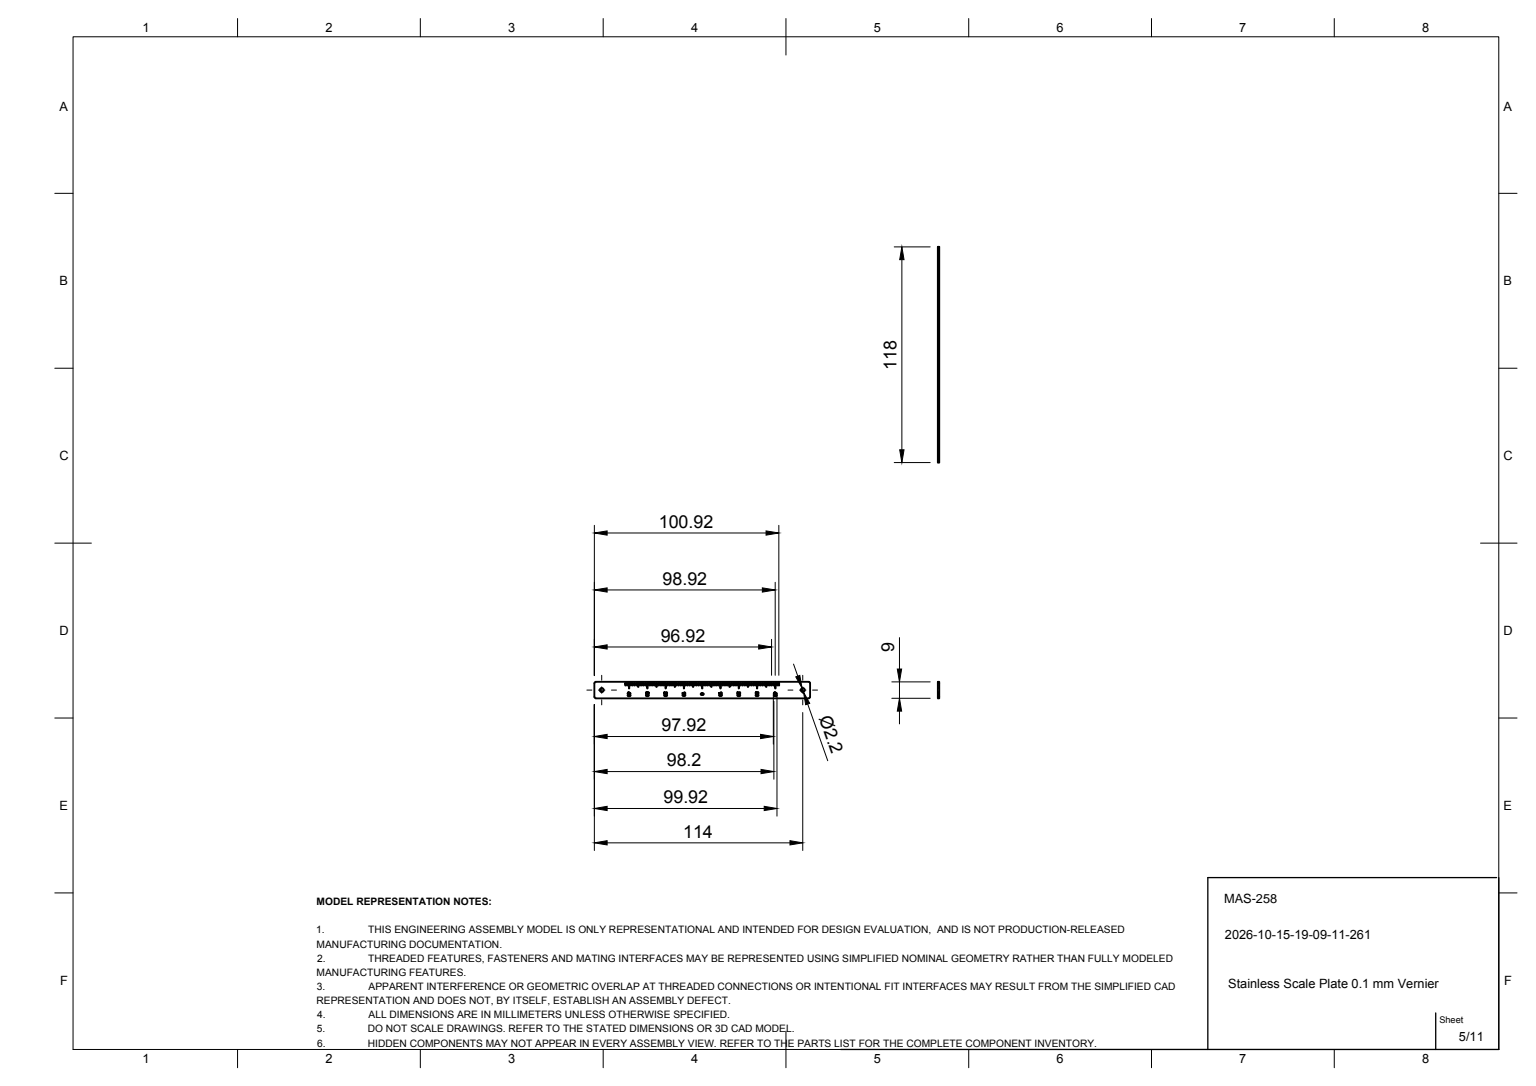
ISO-10303-21;
HEADER;
/* Generated by software containing ST-Developer
 * from STEP Tools, Inc. (www.steptools.com) 
 */

FILE_DESCRIPTION(
/* description */ (''),
/* implementation_level */ '2;1');

FILE_NAME(
/* name */ 'Stainless Scale Plate 0.1 mm Vernier.step',
/* time_stamp */ '2026-10-15T12:29:06-07:00',
/* author */ (''),
/* organization */ (''),
/* preprocessor_version */ 'ST-DEVELOPER v20.2',
/* originating_system */ 'Autodesk Translation Framework v15.15.0.0',
/* authorisation */ '');

FILE_SCHEMA (('AUTOMOTIVE_DESIGN { 1 0 10303 214 3 1 1 }'));
ENDSEC;

DATA;
#10=MECHANICAL_DESIGN_GEOMETRIC_PRESENTATION_REPRESENTATION('',(#1744),#135282);
#331=B_SPLINE_SURFACE_WITH_KNOTS('',2,1,((#69951,#69952),(#69953,#69954),
(#69955,#69956)),.UNSPECIFIED.,.F.,.F.,.F.,(3,3),(2,2),(0.,1.),(0.,0.0172800000000002),
 .UNSPECIFIED.);
#332=B_SPLINE_SURFACE_WITH_KNOTS('',2,1,((#69969,#69970),(#69971,#69972),
(#69973,#69974)),.UNSPECIFIED.,.F.,.F.,.F.,(3,3),(2,2),(0.,1.),(0.,0.0172800000000002),
 .UNSPECIFIED.);
#333=B_SPLINE_SURFACE_WITH_KNOTS('',2,1,((#69984,#69985),(#69986,#69987),
(#69988,#69989)),.UNSPECIFIED.,.F.,.F.,.F.,(3,3),(2,2),(0.,1.),(0.,0.0172800000000002),
 .UNSPECIFIED.);
#334=B_SPLINE_SURFACE_WITH_KNOTS('',2,1,((#69999,#70000),(#70001,#70002),
(#70003,#70004)),.UNSPECIFIED.,.F.,.F.,.F.,(3,3),(2,2),(0.,1.),(0.,0.0172800000000002),
 .UNSPECIFIED.);
#335=B_SPLINE_SURFACE_WITH_KNOTS('',2,1,((#70014,#70015),(#70016,#70017),
(#70018,#70019)),.UNSPECIFIED.,.F.,.F.,.F.,(3,3),(2,2),(0.,1.),(0.,0.0172800000000002),
 .UNSPECIFIED.);
#336=B_SPLINE_SURFACE_WITH_KNOTS('',2,1,((#70029,#70030),(#70031,#70032),
(#70033,#70034)),.UNSPECIFIED.,.F.,.F.,.F.,(3,3),(2,2),(0.,1.),(0.,0.0172800000000002),
 .UNSPECIFIED.);
#337=B_SPLINE_SURFACE_WITH_KNOTS('',2,1,((#70044,#70045),(#70046,#70047),
(#70048,#70049)),.UNSPECIFIED.,.F.,.F.,.F.,(3,3),(2,2),(0.,1.),(0.,0.0172800000000002),
 .UNSPECIFIED.);
#338=B_SPLINE_SURFACE_WITH_KNOTS('',2,1,((#70059,#70060),(#70061,#70062),
(#70063,#70064)),.UNSPECIFIED.,.F.,.F.,.F.,(3,3),(2,2),(0.,1.),(0.,0.0172800000000002),
 .UNSPECIFIED.);
#339=B_SPLINE_SURFACE_WITH_KNOTS('',2,1,((#70071,#70072),(#70073,#70074),
(#70075,#70076)),.UNSPECIFIED.,.F.,.F.,.F.,(3,3),(2,2),(0.,1.),(0.,0.0172800000000002),
 .UNSPECIFIED.);
#340=B_SPLINE_SURFACE_WITH_KNOTS('',2,1,((#70089,#70090),(#70091,#70092),
(#70093,#70094)),.UNSPECIFIED.,.F.,.F.,.F.,(3,3),(2,2),(0.,1.),(0.,0.0172800000000002),
 .UNSPECIFIED.);
#341=B_SPLINE_SURFACE_WITH_KNOTS('',2,1,((#70104,#70105),(#70106,#70107),
(#70108,#70109)),.UNSPECIFIED.,.F.,.F.,.F.,(3,3),(2,2),(0.,1.),(0.,0.0172800000000002),
 .UNSPECIFIED.);
#342=B_SPLINE_SURFACE_WITH_KNOTS('',2,1,((#70119,#70120),(#70121,#70122),
(#70123,#70124)),.UNSPECIFIED.,.F.,.F.,.F.,(3,3),(2,2),(0.,1.),(0.,0.0172800000000002),
 .UNSPECIFIED.);
#343=B_SPLINE_SURFACE_WITH_KNOTS('',2,1,((#70134,#70135),(#70136,#70137),
(#70138,#70139)),.UNSPECIFIED.,.F.,.F.,.F.,(3,3),(2,2),(0.,1.),(0.,0.0172800000000002),
 .UNSPECIFIED.);
#344=B_SPLINE_SURFACE_WITH_KNOTS('',2,1,((#70149,#70150),(#70151,#70152),
(#70153,#70154)),.UNSPECIFIED.,.F.,.F.,.F.,(3,3),(2,2),(0.,1.),(0.,0.0172800000000002),
 .UNSPECIFIED.);
#345=B_SPLINE_SURFACE_WITH_KNOTS('',2,1,((#70164,#70165),(#70166,#70167),
(#70168,#70169)),.UNSPECIFIED.,.F.,.F.,.F.,(3,3),(2,2),(0.,1.),(0.,0.0172800000000002),
 .UNSPECIFIED.);
#346=B_SPLINE_SURFACE_WITH_KNOTS('',2,1,((#70179,#70180),(#70181,#70182),
(#70183,#70184)),.UNSPECIFIED.,.F.,.F.,.F.,(3,3),(2,2),(0.,1.),(0.,0.0172800000000002),
 .UNSPECIFIED.);
#347=B_SPLINE_SURFACE_WITH_KNOTS('',2,1,((#70194,#70195),(#70196,#70197),
(#70198,#70199)),.UNSPECIFIED.,.F.,.F.,.F.,(3,3),(2,2),(0.,1.),(0.,0.0172800000000002),
 .UNSPECIFIED.);
#348=B_SPLINE_SURFACE_WITH_KNOTS('',2,1,((#70209,#70210),(#70211,#70212),
(#70213,#70214)),.UNSPECIFIED.,.F.,.F.,.F.,(3,3),(2,2),(0.,1.),(0.,0.0172800000000002),
 .UNSPECIFIED.);
#349=B_SPLINE_SURFACE_WITH_KNOTS('',2,1,((#70224,#70225),(#70226,#70227),
(#70228,#70229)),.UNSPECIFIED.,.F.,.F.,.F.,(3,3),(2,2),(0.,1.),(0.,0.0172800000000002),
 .UNSPECIFIED.);
#350=B_SPLINE_SURFACE_WITH_KNOTS('',2,1,((#70239,#70240),(#70241,#70242),
(#70243,#70244)),.UNSPECIFIED.,.F.,.F.,.F.,(3,3),(2,2),(0.,1.),(0.,0.0172800000000002),
 .UNSPECIFIED.);
#351=B_SPLINE_SURFACE_WITH_KNOTS('',2,1,((#70339,#70340),(#70341,#70342),
(#70343,#70344)),.UNSPECIFIED.,.F.,.F.,.F.,(3,3),(2,2),(0.,1.),(0.,0.0172800000000002),
 .UNSPECIFIED.);
#352=B_SPLINE_SURFACE_WITH_KNOTS('',2,1,((#70357,#70358),(#70359,#70360),
(#70361,#70362)),.UNSPECIFIED.,.F.,.F.,.F.,(3,3),(2,2),(0.,1.),(0.,0.0172800000000002),
 .UNSPECIFIED.);
#353=B_SPLINE_SURFACE_WITH_KNOTS('',2,1,((#70372,#70373),(#70374,#70375),
(#70376,#70377)),.UNSPECIFIED.,.F.,.F.,.F.,(3,3),(2,2),(0.,1.),(0.,0.0172800000000002),
 .UNSPECIFIED.);
#354=B_SPLINE_SURFACE_WITH_KNOTS('',2,1,((#70387,#70388),(#70389,#70390),
(#70391,#70392)),.UNSPECIFIED.,.F.,.F.,.F.,(3,3),(2,2),(0.,1.),(0.,0.0172800000000002),
 .UNSPECIFIED.);
#355=B_SPLINE_SURFACE_WITH_KNOTS('',2,1,((#70402,#70403),(#70404,#70405),
(#70406,#70407)),.UNSPECIFIED.,.F.,.F.,.F.,(3,3),(2,2),(0.,1.),(0.,0.0172800000000002),
 .UNSPECIFIED.);
#356=B_SPLINE_SURFACE_WITH_KNOTS('',2,1,((#70417,#70418),(#70419,#70420),
(#70421,#70422)),.UNSPECIFIED.,.F.,.F.,.F.,(3,3),(2,2),(0.,1.),(0.,0.0172800000000002),
 .UNSPECIFIED.);
#357=B_SPLINE_SURFACE_WITH_KNOTS('',2,1,((#70432,#70433),(#70434,#70435),
(#70436,#70437)),.UNSPECIFIED.,.F.,.F.,.F.,(3,3),(2,2),(0.,1.),(0.,0.0172800000000002),
 .UNSPECIFIED.);
#358=B_SPLINE_SURFACE_WITH_KNOTS('',2,1,((#70447,#70448),(#70449,#70450),
(#70451,#70452)),.UNSPECIFIED.,.F.,.F.,.F.,(3,3),(2,2),(0.,1.),(0.,0.0172800000000002),
 .UNSPECIFIED.);
#359=B_SPLINE_SURFACE_WITH_KNOTS('',2,1,((#70459,#70460),(#70461,#70462),
(#70463,#70464)),.UNSPECIFIED.,.F.,.F.,.F.,(3,3),(2,2),(0.,1.),(0.,0.0172800000000002),
 .UNSPECIFIED.);
#360=B_SPLINE_SURFACE_WITH_KNOTS('',2,1,((#70477,#70478),(#70479,#70480),
(#70481,#70482)),.UNSPECIFIED.,.F.,.F.,.F.,(3,3),(2,2),(0.,1.),(0.,0.0172800000000002),
 .UNSPECIFIED.);
#361=B_SPLINE_SURFACE_WITH_KNOTS('',2,1,((#70492,#70493),(#70494,#70495),
(#70496,#70497)),.UNSPECIFIED.,.F.,.F.,.F.,(3,3),(2,2),(0.,1.),(0.,0.0172800000000002),
 .UNSPECIFIED.);
#362=B_SPLINE_SURFACE_WITH_KNOTS('',2,1,((#70507,#70508),(#70509,#70510),
(#70511,#70512)),.UNSPECIFIED.,.F.,.F.,.F.,(3,3),(2,2),(0.,1.),(0.,0.0172800000000002),
 .UNSPECIFIED.);
#363=B_SPLINE_SURFACE_WITH_KNOTS('',2,1,((#70522,#70523),(#70524,#70525),
(#70526,#70527)),.UNSPECIFIED.,.F.,.F.,.F.,(3,3),(2,2),(0.,1.),(0.,0.0172800000000002),
 .UNSPECIFIED.);
#364=B_SPLINE_SURFACE_WITH_KNOTS('',2,1,((#70537,#70538),(#70539,#70540),
(#70541,#70542)),.UNSPECIFIED.,.F.,.F.,.F.,(3,3),(2,2),(0.,1.),(0.,0.0172800000000002),
 .UNSPECIFIED.);
#365=B_SPLINE_SURFACE_WITH_KNOTS('',2,1,((#70552,#70553),(#70554,#70555),
(#70556,#70557)),.UNSPECIFIED.,.F.,.F.,.F.,(3,3),(2,2),(0.,1.),(0.,0.0172800000000002),
 .UNSPECIFIED.);
#366=B_SPLINE_SURFACE_WITH_KNOTS('',2,1,((#70567,#70568),(#70569,#70570),
(#70571,#70572)),.UNSPECIFIED.,.F.,.F.,.F.,(3,3),(2,2),(0.,1.),(0.,0.0172800000000002),
 .UNSPECIFIED.);
#367=B_SPLINE_SURFACE_WITH_KNOTS('',2,1,((#70582,#70583),(#70584,#70585),
(#70586,#70587)),.UNSPECIFIED.,.F.,.F.,.F.,(3,3),(2,2),(0.,1.),(0.,0.0172800000000002),
 .UNSPECIFIED.);
#368=B_SPLINE_SURFACE_WITH_KNOTS('',2,1,((#70597,#70598),(#70599,#70600),
(#70601,#70602)),.UNSPECIFIED.,.F.,.F.,.F.,(3,3),(2,2),(0.,1.),(0.,0.0172800000000002),
 .UNSPECIFIED.);
#369=B_SPLINE_SURFACE_WITH_KNOTS('',2,1,((#70612,#70613),(#70614,#70615),
(#70616,#70617)),.UNSPECIFIED.,.F.,.F.,.F.,(3,3),(2,2),(0.,1.),(0.,0.0172800000000002),
 .UNSPECIFIED.);
#370=B_SPLINE_SURFACE_WITH_KNOTS('',2,1,((#70627,#70628),(#70629,#70630),
(#70631,#70632)),.UNSPECIFIED.,.F.,.F.,.F.,(3,3),(2,2),(0.,1.),(0.,0.0172800000000002),
 .UNSPECIFIED.);
#371=B_SPLINE_SURFACE_WITH_KNOTS('',2,1,((#70640,#70641),(#70642,#70643),
(#70644,#70645)),.UNSPECIFIED.,.F.,.F.,.F.,(3,3),(2,2),(0.,1.),(0.,0.0172800000000002),
 .UNSPECIFIED.);
#372=B_SPLINE_SURFACE_WITH_KNOTS('',2,1,((#70658,#70659),(#70660,#70661),
(#70662,#70663)),.UNSPECIFIED.,.F.,.F.,.F.,(3,3),(2,2),(0.,1.),(0.,0.0172800000000002),
 .UNSPECIFIED.);
#373=B_SPLINE_SURFACE_WITH_KNOTS('',2,1,((#70673,#70674),(#70675,#70676),
(#70677,#70678)),.UNSPECIFIED.,.F.,.F.,.F.,(3,3),(2,2),(0.,1.),(0.,0.0172800000000002),
 .UNSPECIFIED.);
#374=B_SPLINE_SURFACE_WITH_KNOTS('',2,1,((#70688,#70689),(#70690,#70691),
(#70692,#70693)),.UNSPECIFIED.,.F.,.F.,.F.,(3,3),(2,2),(0.,1.),(0.,0.0172800000000002),
 .UNSPECIFIED.);
#375=B_SPLINE_SURFACE_WITH_KNOTS('',2,1,((#70703,#70704),(#70705,#70706),
(#70707,#70708)),.UNSPECIFIED.,.F.,.F.,.F.,(3,3),(2,2),(0.,1.),(0.,0.0172800000000002),
 .UNSPECIFIED.);
#376=B_SPLINE_SURFACE_WITH_KNOTS('',2,1,((#70718,#70719),(#70720,#70721),
(#70722,#70723)),.UNSPECIFIED.,.F.,.F.,.F.,(3,3),(2,2),(0.,1.),(0.,0.0172800000000002),
 .UNSPECIFIED.);
#377=B_SPLINE_SURFACE_WITH_KNOTS('',2,1,((#70733,#70734),(#70735,#70736),
(#70737,#70738)),.UNSPECIFIED.,.F.,.F.,.F.,(3,3),(2,2),(0.,1.),(0.,0.0172800000000002),
 .UNSPECIFIED.);
#378=B_SPLINE_SURFACE_WITH_KNOTS('',2,1,((#70748,#70749),(#70750,#70751),
(#70752,#70753)),.UNSPECIFIED.,.F.,.F.,.F.,(3,3),(2,2),(0.,1.),(0.,0.0172800000000002),
 .UNSPECIFIED.);
#379=B_SPLINE_SURFACE_WITH_KNOTS('',2,1,((#70763,#70764),(#70765,#70766),
(#70767,#70768)),.UNSPECIFIED.,.F.,.F.,.F.,(3,3),(2,2),(0.,1.),(0.,0.0172800000000002),
 .UNSPECIFIED.);
#380=B_SPLINE_SURFACE_WITH_KNOTS('',2,1,((#70778,#70779),(#70780,#70781),
(#70782,#70783)),.UNSPECIFIED.,.F.,.F.,.F.,(3,3),(2,2),(0.,1.),(0.,0.0172800000000002),
 .UNSPECIFIED.);
#381=B_SPLINE_SURFACE_WITH_KNOTS('',2,1,((#70793,#70794),(#70795,#70796),
(#70797,#70798)),.UNSPECIFIED.,.F.,.F.,.F.,(3,3),(2,2),(0.,1.),(0.,0.0172800000000002),
 .UNSPECIFIED.);
#382=B_SPLINE_SURFACE_WITH_KNOTS('',2,1,((#70808,#70809),(#70810,#70811),
(#70812,#70813)),.UNSPECIFIED.,.F.,.F.,.F.,(3,3),(2,2),(0.,1.),(0.,0.0172800000000002),
 .UNSPECIFIED.);
#383=B_SPLINE_SURFACE_WITH_KNOTS('',2,1,((#70829,#70830),(#70831,#70832),
(#70833,#70834)),.UNSPECIFIED.,.F.,.F.,.F.,(3,3),(2,2),(0.,1.),(0.,0.0172800000000002),
 .UNSPECIFIED.);
#384=B_SPLINE_SURFACE_WITH_KNOTS('',2,1,((#70844,#70845),(#70846,#70847),
(#70848,#70849)),.UNSPECIFIED.,.F.,.F.,.F.,(3,3),(2,2),(0.,1.),(0.,0.0172800000000002),
 .UNSPECIFIED.);
#385=B_SPLINE_SURFACE_WITH_KNOTS('',2,1,((#70859,#70860),(#70861,#70862),
(#70863,#70864)),.UNSPECIFIED.,.F.,.F.,.F.,(3,3),(2,2),(0.,1.),(0.,0.0172800000000002),
 .UNSPECIFIED.);
#386=B_SPLINE_SURFACE_WITH_KNOTS('',2,1,((#70874,#70875),(#70876,#70877),
(#70878,#70879)),.UNSPECIFIED.,.F.,.F.,.F.,(3,3),(2,2),(0.,1.),(0.,0.0172800000000002),
 .UNSPECIFIED.);
#387=B_SPLINE_SURFACE_WITH_KNOTS('',2,1,((#70889,#70890),(#70891,#70892),
(#70893,#70894)),.UNSPECIFIED.,.F.,.F.,.F.,(3,3),(2,2),(0.,1.),(0.,0.0172800000000002),
 .UNSPECIFIED.);
#388=B_SPLINE_SURFACE_WITH_KNOTS('',2,1,((#70904,#70905),(#70906,#70907),
(#70908,#70909)),.UNSPECIFIED.,.F.,.F.,.F.,(3,3),(2,2),(0.,1.),(0.,0.0172800000000002),
 .UNSPECIFIED.);
#389=B_SPLINE_SURFACE_WITH_KNOTS('',2,1,((#70919,#70920),(#70921,#70922),
(#70923,#70924)),.UNSPECIFIED.,.F.,.F.,.F.,(3,3),(2,2),(0.,1.),(0.,0.0172800000000002),
 .UNSPECIFIED.);
#390=B_SPLINE_SURFACE_WITH_KNOTS('',2,1,((#70940,#70941),(#70942,#70943),
(#70944,#70945)),.UNSPECIFIED.,.F.,.F.,.F.,(3,3),(2,2),(0.,1.),(0.,0.0172800000000002),
 .UNSPECIFIED.);
#391=B_SPLINE_SURFACE_WITH_KNOTS('',2,1,((#70955,#70956),(#70957,#70958),
(#70959,#70960)),.UNSPECIFIED.,.F.,.F.,.F.,(3,3),(2,2),(0.,1.),(0.,0.0172800000000002),
 .UNSPECIFIED.);
#392=B_SPLINE_SURFACE_WITH_KNOTS('',2,1,((#70970,#70971),(#70972,#70973),
(#70974,#70975)),.UNSPECIFIED.,.F.,.F.,.F.,(3,3),(2,2),(0.,1.),(0.,0.0172800000000002),
 .UNSPECIFIED.);
#393=B_SPLINE_SURFACE_WITH_KNOTS('',2,1,((#70985,#70986),(#70987,#70988),
(#70989,#70990)),.UNSPECIFIED.,.F.,.F.,.F.,(3,3),(2,2),(0.,1.),(0.,0.0172800000000002),
 .UNSPECIFIED.);
#394=B_SPLINE_SURFACE_WITH_KNOTS('',2,1,((#71000,#71001),(#71002,#71003),
(#71004,#71005)),.UNSPECIFIED.,.F.,.F.,.F.,(3,3),(2,2),(0.,1.),(0.,0.0172800000000002),
 .UNSPECIFIED.);
#395=B_SPLINE_SURFACE_WITH_KNOTS('',2,1,((#71015,#71016),(#71017,#71018),
(#71019,#71020)),.UNSPECIFIED.,.F.,.F.,.F.,(3,3),(2,2),(0.,1.),(0.,0.0172800000000002),
 .UNSPECIFIED.);
#396=B_SPLINE_SURFACE_WITH_KNOTS('',2,1,((#71030,#71031),(#71032,#71033),
(#71034,#71035)),.UNSPECIFIED.,.F.,.F.,.F.,(3,3),(2,2),(0.,1.),(0.,0.0172800000000002),
 .UNSPECIFIED.);
#397=B_SPLINE_SURFACE_WITH_KNOTS('',2,1,((#71051,#71052),(#71053,#71054),
(#71055,#71056)),.UNSPECIFIED.,.F.,.F.,.F.,(3,3),(2,2),(0.,1.),(0.,0.0172800000000002),
 .UNSPECIFIED.);
#398=B_SPLINE_SURFACE_WITH_KNOTS('',2,1,((#71065,#71066),(#71067,#71068),
(#71069,#71070)),.UNSPECIFIED.,.F.,.F.,.F.,(3,3),(2,2),(0.,1.),(0.,0.0172800000000002),
 .UNSPECIFIED.);
#399=B_SPLINE_SURFACE_WITH_KNOTS('',2,1,((#71083,#71084),(#71085,#71086),
(#71087,#71088)),.UNSPECIFIED.,.F.,.F.,.F.,(3,3),(2,2),(0.,1.),(0.,0.0172800000000002),
 .UNSPECIFIED.);
#400=B_SPLINE_SURFACE_WITH_KNOTS('',2,1,((#71098,#71099),(#71100,#71101),
(#71102,#71103)),.UNSPECIFIED.,.F.,.F.,.F.,(3,3),(2,2),(0.,1.),(0.,0.0172800000000002),
 .UNSPECIFIED.);
#401=B_SPLINE_SURFACE_WITH_KNOTS('',2,1,((#71113,#71114),(#71115,#71116),
(#71117,#71118)),.UNSPECIFIED.,.F.,.F.,.F.,(3,3),(2,2),(0.,1.),(0.,0.0172800000000002),
 .UNSPECIFIED.);
#402=B_SPLINE_SURFACE_WITH_KNOTS('',2,1,((#71128,#71129),(#71130,#71131),
(#71132,#71133)),.UNSPECIFIED.,.F.,.F.,.F.,(3,3),(2,2),(0.,1.),(0.,0.0172800000000002),
 .UNSPECIFIED.);
#403=B_SPLINE_SURFACE_WITH_KNOTS('',2,1,((#71143,#71144),(#71145,#71146),
(#71147,#71148)),.UNSPECIFIED.,.F.,.F.,.F.,(3,3),(2,2),(0.,1.),(0.,0.0172800000000002),
 .UNSPECIFIED.);
#404=B_SPLINE_SURFACE_WITH_KNOTS('',2,1,((#71158,#71159),(#71160,#71161),
(#71162,#71163)),.UNSPECIFIED.,.F.,.F.,.F.,(3,3),(2,2),(0.,1.),(0.,0.0172800000000002),
 .UNSPECIFIED.);
#405=B_SPLINE_SURFACE_WITH_KNOTS('',2,1,((#71173,#71174),(#71175,#71176),
(#71177,#71178)),.UNSPECIFIED.,.F.,.F.,.F.,(3,3),(2,2),(0.,1.),(0.,0.0172800000000002),
 .UNSPECIFIED.);
#406=B_SPLINE_SURFACE_WITH_KNOTS('',2,1,((#71185,#71186),(#71187,#71188),
(#71189,#71190)),.UNSPECIFIED.,.F.,.F.,.F.,(3,3),(2,2),(0.,1.),(0.,0.0172800000000002),
 .UNSPECIFIED.);
#407=B_SPLINE_SURFACE_WITH_KNOTS('',2,1,((#71203,#71204),(#71205,#71206),
(#71207,#71208)),.UNSPECIFIED.,.F.,.F.,.F.,(3,3),(2,2),(0.,1.),(0.,0.0172800000000002),
 .UNSPECIFIED.);
#408=B_SPLINE_SURFACE_WITH_KNOTS('',2,1,((#71218,#71219),(#71220,#71221),
(#71222,#71223)),.UNSPECIFIED.,.F.,.F.,.F.,(3,3),(2,2),(0.,1.),(0.,0.0172800000000002),
 .UNSPECIFIED.);
#409=B_SPLINE_SURFACE_WITH_KNOTS('',2,1,((#71233,#71234),(#71235,#71236),
(#71237,#71238)),.UNSPECIFIED.,.F.,.F.,.F.,(3,3),(2,2),(0.,1.),(0.,0.0172800000000002),
 .UNSPECIFIED.);
#410=B_SPLINE_SURFACE_WITH_KNOTS('',2,1,((#71248,#71249),(#71250,#71251),
(#71252,#71253)),.UNSPECIFIED.,.F.,.F.,.F.,(3,3),(2,2),(0.,1.),(0.,0.0172800000000002),
 .UNSPECIFIED.);
#411=B_SPLINE_SURFACE_WITH_KNOTS('',2,1,((#71263,#71264),(#71265,#71266),
(#71267,#71268)),.UNSPECIFIED.,.F.,.F.,.F.,(3,3),(2,2),(0.,1.),(0.,0.0172800000000002),
 .UNSPECIFIED.);
#412=B_SPLINE_SURFACE_WITH_KNOTS('',2,1,((#71278,#71279),(#71280,#71281),
(#71282,#71283)),.UNSPECIFIED.,.F.,.F.,.F.,(3,3),(2,2),(0.,1.),(0.,0.0172800000000002),
 .UNSPECIFIED.);
#413=B_SPLINE_SURFACE_WITH_KNOTS('',2,1,((#71293,#71294),(#71295,#71296),
(#71297,#71298)),.UNSPECIFIED.,.F.,.F.,.F.,(3,3),(2,2),(0.,1.),(0.,0.0172800000000002),
 .UNSPECIFIED.);
#414=B_SPLINE_SURFACE_WITH_KNOTS('',2,1,((#71308,#71309),(#71310,#71311),
(#71312,#71313)),.UNSPECIFIED.,.F.,.F.,.F.,(3,3),(2,2),(0.,1.),(0.,0.0172800000000002),
 .UNSPECIFIED.);
#415=B_SPLINE_SURFACE_WITH_KNOTS('',2,1,((#71323,#71324),(#71325,#71326),
(#71327,#71328)),.UNSPECIFIED.,.F.,.F.,.F.,(3,3),(2,2),(0.,1.),(0.,0.0172800000000002),
 .UNSPECIFIED.);
#416=B_SPLINE_SURFACE_WITH_KNOTS('',2,1,((#71338,#71339),(#71340,#71341),
(#71342,#71343)),.UNSPECIFIED.,.F.,.F.,.F.,(3,3),(2,2),(0.,1.),(0.,0.0172800000000002),
 .UNSPECIFIED.);
#417=B_SPLINE_SURFACE_WITH_KNOTS('',2,1,((#71353,#71354),(#71355,#71356),
(#71357,#71358)),.UNSPECIFIED.,.F.,.F.,.F.,(3,3),(2,2),(0.,1.),(0.,0.0172800000000002),
 .UNSPECIFIED.);
#418=B_SPLINE_SURFACE_WITH_KNOTS('',2,1,((#71366,#71367),(#71368,#71369),
(#71370,#71371)),.UNSPECIFIED.,.F.,.F.,.F.,(3,3),(2,2),(0.,1.),(0.,0.0172800000000002),
 .UNSPECIFIED.);
#419=B_SPLINE_SURFACE_WITH_KNOTS('',2,1,((#71384,#71385),(#71386,#71387),
(#71388,#71389)),.UNSPECIFIED.,.F.,.F.,.F.,(3,3),(2,2),(0.,1.),(0.,0.0172800000000002),
 .UNSPECIFIED.);
#420=B_SPLINE_SURFACE_WITH_KNOTS('',2,1,((#71399,#71400),(#71401,#71402),
(#71403,#71404)),.UNSPECIFIED.,.F.,.F.,.F.,(3,3),(2,2),(0.,1.),(0.,0.0172800000000002),
 .UNSPECIFIED.);
#421=B_SPLINE_SURFACE_WITH_KNOTS('',2,1,((#71414,#71415),(#71416,#71417),
(#71418,#71419)),.UNSPECIFIED.,.F.,.F.,.F.,(3,3),(2,2),(0.,1.),(0.,0.0172800000000002),
 .UNSPECIFIED.);
#422=B_SPLINE_SURFACE_WITH_KNOTS('',2,1,((#71429,#71430),(#71431,#71432),
(#71433,#71434)),.UNSPECIFIED.,.F.,.F.,.F.,(3,3),(2,2),(0.,1.),(0.,0.0172800000000002),
 .UNSPECIFIED.);
#423=B_SPLINE_SURFACE_WITH_KNOTS('',2,1,((#71444,#71445),(#71446,#71447),
(#71448,#71449)),.UNSPECIFIED.,.F.,.F.,.F.,(3,3),(2,2),(0.,1.),(0.,0.0172800000000002),
 .UNSPECIFIED.);
#424=B_SPLINE_SURFACE_WITH_KNOTS('',2,1,((#71459,#71460),(#71461,#71462),
(#71463,#71464)),.UNSPECIFIED.,.F.,.F.,.F.,(3,3),(2,2),(0.,1.),(0.,0.0172800000000002),
 .UNSPECIFIED.);
#425=B_SPLINE_SURFACE_WITH_KNOTS('',2,1,((#71474,#71475),(#71476,#71477),
(#71478,#71479)),.UNSPECIFIED.,.F.,.F.,.F.,(3,3),(2,2),(0.,1.),(0.,0.0172800000000002),
 .UNSPECIFIED.);
#426=B_SPLINE_SURFACE_WITH_KNOTS('',2,1,((#71489,#71490),(#71491,#71492),
(#71493,#71494)),.UNSPECIFIED.,.F.,.F.,.F.,(3,3),(2,2),(0.,1.),(0.,0.0172800000000002),
 .UNSPECIFIED.);
#427=B_SPLINE_SURFACE_WITH_KNOTS('',2,1,((#71510,#71511),(#71512,#71513),
(#71514,#71515)),.UNSPECIFIED.,.F.,.F.,.F.,(3,3),(2,2),(0.,1.),(0.,0.0172800000000002),
 .UNSPECIFIED.);
#428=B_SPLINE_SURFACE_WITH_KNOTS('',2,1,((#71525,#71526),(#71527,#71528),
(#71529,#71530)),.UNSPECIFIED.,.F.,.F.,.F.,(3,3),(2,2),(0.,1.),(0.,0.0172800000000002),
 .UNSPECIFIED.);
#429=B_SPLINE_SURFACE_WITH_KNOTS('',2,1,((#71540,#71541),(#71542,#71543),
(#71544,#71545)),.UNSPECIFIED.,.F.,.F.,.F.,(3,3),(2,2),(0.,1.),(0.,0.0172800000000002),
 .UNSPECIFIED.);
#430=B_SPLINE_SURFACE_WITH_KNOTS('',2,1,((#71555,#71556),(#71557,#71558),
(#71559,#71560)),.UNSPECIFIED.,.F.,.F.,.F.,(3,3),(2,2),(0.,1.),(0.,0.0172800000000002),
 .UNSPECIFIED.);
#431=B_SPLINE_SURFACE_WITH_KNOTS('',2,1,((#71570,#71571),(#71572,#71573),
(#71574,#71575)),.UNSPECIFIED.,.F.,.F.,.F.,(3,3),(2,2),(0.,1.),(0.,0.0172800000000002),
 .UNSPECIFIED.);
#432=B_SPLINE_SURFACE_WITH_KNOTS('',2,1,((#71585,#71586),(#71587,#71588),
(#71589,#71590)),.UNSPECIFIED.,.F.,.F.,.F.,(3,3),(2,2),(0.,1.),(0.,0.0172800000000002),
 .UNSPECIFIED.);
#433=B_SPLINE_SURFACE_WITH_KNOTS('',2,1,((#71600,#71601),(#71602,#71603),
(#71604,#71605)),.UNSPECIFIED.,.F.,.F.,.F.,(3,3),(2,2),(0.,1.),(0.,0.0172800000000002),
 .UNSPECIFIED.);
#434=B_SPLINE_SURFACE_WITH_KNOTS('',2,1,((#71615,#71616),(#71617,#71618),
(#71619,#71620)),.UNSPECIFIED.,.F.,.F.,.F.,(3,3),(2,2),(0.,1.),(0.,0.0172800000000002),
 .UNSPECIFIED.);
#435=B_SPLINE_SURFACE_WITH_KNOTS('',2,1,((#71630,#71631),(#71632,#71633),
(#71634,#71635)),.UNSPECIFIED.,.F.,.F.,.F.,(3,3),(2,2),(0.,1.),(0.,0.0172800000000002),
 .UNSPECIFIED.);
#436=B_SPLINE_SURFACE_WITH_KNOTS('',2,1,((#71662,#71663),(#71664,#71665),
(#71666,#71667)),.UNSPECIFIED.,.F.,.F.,.F.,(3,3),(2,2),(0.,1.),(0.,0.0172800000000002),
 .UNSPECIFIED.);
#437=B_SPLINE_SURFACE_WITH_KNOTS('',2,1,((#71680,#71681),(#71682,#71683),
(#71684,#71685)),.UNSPECIFIED.,.F.,.F.,.F.,(3,3),(2,2),(0.,1.),(0.,0.0172800000000002),
 .UNSPECIFIED.);
#438=B_SPLINE_SURFACE_WITH_KNOTS('',2,1,((#71695,#71696),(#71697,#71698),
(#71699,#71700)),.UNSPECIFIED.,.F.,.F.,.F.,(3,3),(2,2),(0.,1.),(0.,0.0172800000000002),
 .UNSPECIFIED.);
#439=B_SPLINE_SURFACE_WITH_KNOTS('',2,1,((#71710,#71711),(#71712,#71713),
(#71714,#71715)),.UNSPECIFIED.,.F.,.F.,.F.,(3,3),(2,2),(0.,1.),(0.,0.0172800000000002),
 .UNSPECIFIED.);
#440=B_SPLINE_SURFACE_WITH_KNOTS('',2,1,((#71725,#71726),(#71727,#71728),
(#71729,#71730)),.UNSPECIFIED.,.F.,.F.,.F.,(3,3),(2,2),(0.,1.),(0.,0.0172800000000002),
 .UNSPECIFIED.);
#441=B_SPLINE_SURFACE_WITH_KNOTS('',2,1,((#71740,#71741),(#71742,#71743),
(#71744,#71745)),.UNSPECIFIED.,.F.,.F.,.F.,(3,3),(2,2),(0.,1.),(0.,0.0172800000000002),
 .UNSPECIFIED.);
#442=B_SPLINE_SURFACE_WITH_KNOTS('',2,1,((#71755,#71756),(#71757,#71758),
(#71759,#71760)),.UNSPECIFIED.,.F.,.F.,.F.,(3,3),(2,2),(0.,1.),(0.,0.0172800000000002),
 .UNSPECIFIED.);
#443=B_SPLINE_SURFACE_WITH_KNOTS('',2,1,((#71770,#71771),(#71772,#71773),
(#71774,#71775)),.UNSPECIFIED.,.F.,.F.,.F.,(3,3),(2,2),(0.,1.),(0.,0.0172800000000002),
 .UNSPECIFIED.);
#444=B_SPLINE_SURFACE_WITH_KNOTS('',2,1,((#71782,#71783),(#71784,#71785),
(#71786,#71787)),.UNSPECIFIED.,.F.,.F.,.F.,(3,3),(2,2),(0.,1.),(0.,0.0172800000000002),
 .UNSPECIFIED.);
#445=B_SPLINE_SURFACE_WITH_KNOTS('',2,1,((#71800,#71801),(#71802,#71803),
(#71804,#71805)),.UNSPECIFIED.,.F.,.F.,.F.,(3,3),(2,2),(0.,1.),(0.,0.0172800000000002),
 .UNSPECIFIED.);
#446=B_SPLINE_SURFACE_WITH_KNOTS('',2,1,((#71815,#71816),(#71817,#71818),
(#71819,#71820)),.UNSPECIFIED.,.F.,.F.,.F.,(3,3),(2,2),(0.,1.),(0.,0.0172800000000002),
 .UNSPECIFIED.);
#447=B_SPLINE_SURFACE_WITH_KNOTS('',2,1,((#71830,#71831),(#71832,#71833),
(#71834,#71835)),.UNSPECIFIED.,.F.,.F.,.F.,(3,3),(2,2),(0.,1.),(0.,0.0172800000000002),
 .UNSPECIFIED.);
#448=B_SPLINE_SURFACE_WITH_KNOTS('',2,1,((#71845,#71846),(#71847,#71848),
(#71849,#71850)),.UNSPECIFIED.,.F.,.F.,.F.,(3,3),(2,2),(0.,1.),(0.,0.0172800000000002),
 .UNSPECIFIED.);
#449=B_SPLINE_SURFACE_WITH_KNOTS('',2,1,((#71860,#71861),(#71862,#71863),
(#71864,#71865)),.UNSPECIFIED.,.F.,.F.,.F.,(3,3),(2,2),(0.,1.),(0.,0.0172800000000002),
 .UNSPECIFIED.);
#450=B_SPLINE_SURFACE_WITH_KNOTS('',2,1,((#71875,#71876),(#71877,#71878),
(#71879,#71880)),.UNSPECIFIED.,.F.,.F.,.F.,(3,3),(2,2),(0.,1.),(0.,0.0172800000000002),
 .UNSPECIFIED.);
#451=B_SPLINE_SURFACE_WITH_KNOTS('',2,1,((#71890,#71891),(#71892,#71893),
(#71894,#71895)),.UNSPECIFIED.,.F.,.F.,.F.,(3,3),(2,2),(0.,1.),(0.,0.0172800000000002),
 .UNSPECIFIED.);
#452=B_SPLINE_SURFACE_WITH_KNOTS('',2,1,((#71905,#71906),(#71907,#71908),
(#71909,#71910)),.UNSPECIFIED.,.F.,.F.,.F.,(3,3),(2,2),(0.,1.),(0.,0.0172800000000002),
 .UNSPECIFIED.);
#453=B_SPLINE_SURFACE_WITH_KNOTS('',2,1,((#71920,#71921),(#71922,#71923),
(#71924,#71925)),.UNSPECIFIED.,.F.,.F.,.F.,(3,3),(2,2),(0.,1.),(0.,0.0172800000000002),
 .UNSPECIFIED.);
#454=B_SPLINE_SURFACE_WITH_KNOTS('',2,1,((#71935,#71936),(#71937,#71938),
(#71939,#71940)),.UNSPECIFIED.,.F.,.F.,.F.,(3,3),(2,2),(0.,1.),(0.,0.0172800000000002),
 .UNSPECIFIED.);
#455=B_SPLINE_SURFACE_WITH_KNOTS('',2,1,((#71950,#71951),(#71952,#71953),
(#71954,#71955)),.UNSPECIFIED.,.F.,.F.,.F.,(3,3),(2,2),(0.,1.),(0.,0.0172800000000002),
 .UNSPECIFIED.);
#456=B_SPLINE_SURFACE_WITH_KNOTS('',2,1,((#71972,#71973),(#71974,#71975),
(#71976,#71977)),.UNSPECIFIED.,.F.,.F.,.F.,(3,3),(2,2),(0.,1.),(0.,0.0172800000000002),
 .UNSPECIFIED.);
#457=B_SPLINE_SURFACE_WITH_KNOTS('',2,1,((#71987,#71988),(#71989,#71990),
(#71991,#71992)),.UNSPECIFIED.,.F.,.F.,.F.,(3,3),(2,2),(0.,1.),(0.,0.0172800000000002),
 .UNSPECIFIED.);
#458=B_SPLINE_SURFACE_WITH_KNOTS('',2,1,((#72008,#72009),(#72010,#72011),
(#72012,#72013)),.UNSPECIFIED.,.F.,.F.,.F.,(3,3),(2,2),(0.,1.),(0.,0.0172800000000002),
 .UNSPECIFIED.);
#459=B_SPLINE_SURFACE_WITH_KNOTS('',2,1,((#72023,#72024),(#72025,#72026),
(#72027,#72028)),.UNSPECIFIED.,.F.,.F.,.F.,(3,3),(2,2),(0.,1.),(0.,0.0172800000000002),
 .UNSPECIFIED.);
#460=B_SPLINE_SURFACE_WITH_KNOTS('',2,1,((#72055,#72056),(#72057,#72058),
(#72059,#72060)),.UNSPECIFIED.,.F.,.F.,.F.,(3,3),(2,2),(0.,1.),(0.,0.0172800000000002),
 .UNSPECIFIED.);
#461=B_SPLINE_SURFACE_WITH_KNOTS('',2,1,((#72073,#72074),(#72075,#72076),
(#72077,#72078)),.UNSPECIFIED.,.F.,.F.,.F.,(3,3),(2,2),(0.,1.),(0.,0.0172800000000002),
 .UNSPECIFIED.);
#462=B_SPLINE_SURFACE_WITH_KNOTS('',2,1,((#72088,#72089),(#72090,#72091),
(#72092,#72093)),.UNSPECIFIED.,.F.,.F.,.F.,(3,3),(2,2),(0.,1.),(0.,0.0172800000000002),
 .UNSPECIFIED.);
#463=B_SPLINE_SURFACE_WITH_KNOTS('',2,1,((#72103,#72104),(#72105,#72106),
(#72107,#72108)),.UNSPECIFIED.,.F.,.F.,.F.,(3,3),(2,2),(0.,1.),(0.,0.0172800000000002),
 .UNSPECIFIED.);
#464=B_SPLINE_SURFACE_WITH_KNOTS('',2,1,((#72118,#72119),(#72120,#72121),
(#72122,#72123)),.UNSPECIFIED.,.F.,.F.,.F.,(3,3),(2,2),(0.,1.),(0.,0.0172800000000002),
 .UNSPECIFIED.);
#465=B_SPLINE_SURFACE_WITH_KNOTS('',2,1,((#72133,#72134),(#72135,#72136),
(#72137,#72138)),.UNSPECIFIED.,.F.,.F.,.F.,(3,3),(2,2),(0.,1.),(0.,0.0172800000000002),
 .UNSPECIFIED.);
#466=B_SPLINE_SURFACE_WITH_KNOTS('',2,1,((#72148,#72149),(#72150,#72151),
(#72152,#72153)),.UNSPECIFIED.,.F.,.F.,.F.,(3,3),(2,2),(0.,1.),(0.,0.0172800000000002),
 .UNSPECIFIED.);
#467=B_SPLINE_SURFACE_WITH_KNOTS('',2,1,((#72163,#72164),(#72165,#72166),
(#72167,#72168)),.UNSPECIFIED.,.F.,.F.,.F.,(3,3),(2,2),(0.,1.),(0.,0.0172800000000002),
 .UNSPECIFIED.);
#468=B_SPLINE_SURFACE_WITH_KNOTS('',2,1,((#72175,#72176),(#72177,#72178),
(#72179,#72180)),.UNSPECIFIED.,.F.,.F.,.F.,(3,3),(2,2),(0.,1.),(0.,0.0172800000000002),
 .UNSPECIFIED.);
#469=B_SPLINE_SURFACE_WITH_KNOTS('',2,1,((#72193,#72194),(#72195,#72196),
(#72197,#72198)),.UNSPECIFIED.,.F.,.F.,.F.,(3,3),(2,2),(0.,1.),(0.,0.0172800000000002),
 .UNSPECIFIED.);
#470=B_SPLINE_SURFACE_WITH_KNOTS('',2,1,((#72208,#72209),(#72210,#72211),
(#72212,#72213)),.UNSPECIFIED.,.F.,.F.,.F.,(3,3),(2,2),(0.,1.),(0.,0.0172800000000002),
 .UNSPECIFIED.);
#471=B_SPLINE_SURFACE_WITH_KNOTS('',2,1,((#72223,#72224),(#72225,#72226),
(#72227,#72228)),.UNSPECIFIED.,.F.,.F.,.F.,(3,3),(2,2),(0.,1.),(0.,0.0172800000000002),
 .UNSPECIFIED.);
#472=B_SPLINE_SURFACE_WITH_KNOTS('',2,1,((#72238,#72239),(#72240,#72241),
(#72242,#72243)),.UNSPECIFIED.,.F.,.F.,.F.,(3,3),(2,2),(0.,1.),(0.,0.0172800000000002),
 .UNSPECIFIED.);
#473=B_SPLINE_SURFACE_WITH_KNOTS('',2,1,((#72253,#72254),(#72255,#72256),
(#72257,#72258)),.UNSPECIFIED.,.F.,.F.,.F.,(3,3),(2,2),(0.,1.),(0.,0.0172800000000002),
 .UNSPECIFIED.);
#474=B_SPLINE_SURFACE_WITH_KNOTS('',2,1,((#72268,#72269),(#72270,#72271),
(#72272,#72273)),.UNSPECIFIED.,.F.,.F.,.F.,(3,3),(2,2),(0.,1.),(0.,0.0172800000000002),
 .UNSPECIFIED.);
#475=B_SPLINE_SURFACE_WITH_KNOTS('',2,1,((#72283,#72284),(#72285,#72286),
(#72287,#72288)),.UNSPECIFIED.,.F.,.F.,.F.,(3,3),(2,2),(0.,1.),(0.,0.0172800000000002),
 .UNSPECIFIED.);
#476=B_SPLINE_SURFACE_WITH_KNOTS('',2,1,((#72298,#72299),(#72300,#72301),
(#72302,#72303)),.UNSPECIFIED.,.F.,.F.,.F.,(3,3),(2,2),(0.,1.),(0.,0.0172800000000002),
 .UNSPECIFIED.);
#477=B_SPLINE_SURFACE_WITH_KNOTS('',2,1,((#72313,#72314),(#72315,#72316),
(#72317,#72318)),.UNSPECIFIED.,.F.,.F.,.F.,(3,3),(2,2),(0.,1.),(0.,0.0172800000000002),
 .UNSPECIFIED.);
#478=B_SPLINE_SURFACE_WITH_KNOTS('',2,1,((#72328,#72329),(#72330,#72331),
(#72332,#72333)),.UNSPECIFIED.,.F.,.F.,.F.,(3,3),(2,2),(0.,1.),(0.,0.0172800000000002),
 .UNSPECIFIED.);
#479=B_SPLINE_SURFACE_WITH_KNOTS('',2,1,((#72343,#72344),(#72345,#72346),
(#72347,#72348)),.UNSPECIFIED.,.F.,.F.,.F.,(3,3),(2,2),(0.,1.),(0.,0.0172800000000002),
 .UNSPECIFIED.);
#480=B_SPLINE_SURFACE_WITH_KNOTS('',2,1,((#72357,#72358),(#72359,#72360),
(#72361,#72362)),.UNSPECIFIED.,.F.,.F.,.F.,(3,3),(2,2),(0.,1.),(0.,0.0172800000000002),
 .UNSPECIFIED.);
#481=B_SPLINE_SURFACE_WITH_KNOTS('',2,1,((#72375,#72376),(#72377,#72378),
(#72379,#72380)),.UNSPECIFIED.,.F.,.F.,.F.,(3,3),(2,2),(0.,1.),(0.,0.0172800000000002),
 .UNSPECIFIED.);
#482=B_SPLINE_SURFACE_WITH_KNOTS('',2,1,((#72390,#72391),(#72392,#72393),
(#72394,#72395)),.UNSPECIFIED.,.F.,.F.,.F.,(3,3),(2,2),(0.,1.),(0.,0.0172800000000002),
 .UNSPECIFIED.);
#483=B_SPLINE_SURFACE_WITH_KNOTS('',2,1,((#72405,#72406),(#72407,#72408),
(#72409,#72410)),.UNSPECIFIED.,.F.,.F.,.F.,(3,3),(2,2),(0.,1.),(0.,0.0172800000000002),
 .UNSPECIFIED.);
#484=B_SPLINE_SURFACE_WITH_KNOTS('',2,1,((#72420,#72421),(#72422,#72423),
(#72424,#72425)),.UNSPECIFIED.,.F.,.F.,.F.,(3,3),(2,2),(0.,1.),(0.,0.0172800000000002),
 .UNSPECIFIED.);
#485=B_SPLINE_SURFACE_WITH_KNOTS('',2,1,((#72435,#72436),(#72437,#72438),
(#72439,#72440)),.UNSPECIFIED.,.F.,.F.,.F.,(3,3),(2,2),(0.,1.),(0.,0.0172800000000002),
 .UNSPECIFIED.);
#486=B_SPLINE_SURFACE_WITH_KNOTS('',2,1,((#72450,#72451),(#72452,#72453),
(#72454,#72455)),.UNSPECIFIED.,.F.,.F.,.F.,(3,3),(2,2),(0.,1.),(0.,0.0172800000000002),
 .UNSPECIFIED.);
#487=B_SPLINE_SURFACE_WITH_KNOTS('',2,1,((#72465,#72466),(#72467,#72468),
(#72469,#72470)),.UNSPECIFIED.,.F.,.F.,.F.,(3,3),(2,2),(0.,1.),(0.,0.0172800000000002),
 .UNSPECIFIED.);
#488=B_SPLINE_SURFACE_WITH_KNOTS('',2,1,((#72477,#72478),(#72479,#72480),
(#72481,#72482)),.UNSPECIFIED.,.F.,.F.,.F.,(3,3),(2,2),(0.,1.),(0.,0.0172800000000002),
 .UNSPECIFIED.);
#489=B_SPLINE_SURFACE_WITH_KNOTS('',2,1,((#72495,#72496),(#72497,#72498),
(#72499,#72500)),.UNSPECIFIED.,.F.,.F.,.F.,(3,3),(2,2),(0.,1.),(0.,0.0172800000000002),
 .UNSPECIFIED.);
#490=B_SPLINE_SURFACE_WITH_KNOTS('',2,1,((#72510,#72511),(#72512,#72513),
(#72514,#72515)),.UNSPECIFIED.,.F.,.F.,.F.,(3,3),(2,2),(0.,1.),(0.,0.0172800000000002),
 .UNSPECIFIED.);
#491=B_SPLINE_SURFACE_WITH_KNOTS('',2,1,((#72525,#72526),(#72527,#72528),
(#72529,#72530)),.UNSPECIFIED.,.F.,.F.,.F.,(3,3),(2,2),(0.,1.),(0.,0.0172800000000002),
 .UNSPECIFIED.);
#492=B_SPLINE_SURFACE_WITH_KNOTS('',2,1,((#72540,#72541),(#72542,#72543),
(#72544,#72545)),.UNSPECIFIED.,.F.,.F.,.F.,(3,3),(2,2),(0.,1.),(0.,0.0172800000000002),
 .UNSPECIFIED.);
#493=B_SPLINE_SURFACE_WITH_KNOTS('',2,1,((#72555,#72556),(#72557,#72558),
(#72559,#72560)),.UNSPECIFIED.,.F.,.F.,.F.,(3,3),(2,2),(0.,1.),(0.,0.0172800000000002),
 .UNSPECIFIED.);
#494=B_SPLINE_SURFACE_WITH_KNOTS('',2,1,((#72570,#72571),(#72572,#72573),
(#72574,#72575)),.UNSPECIFIED.,.F.,.F.,.F.,(3,3),(2,2),(0.,1.),(0.,0.0172800000000002),
 .UNSPECIFIED.);
#495=B_SPLINE_SURFACE_WITH_KNOTS('',2,1,((#72585,#72586),(#72587,#72588),
(#72589,#72590)),.UNSPECIFIED.,.F.,.F.,.F.,(3,3),(2,2),(0.,1.),(0.,0.0172800000000002),
 .UNSPECIFIED.);
#496=B_SPLINE_SURFACE_WITH_KNOTS('',2,1,((#72600,#72601),(#72602,#72603),
(#72604,#72605)),.UNSPECIFIED.,.F.,.F.,.F.,(3,3),(2,2),(0.,1.),(0.,0.0172800000000002),
 .UNSPECIFIED.);
#497=B_SPLINE_SURFACE_WITH_KNOTS('',2,1,((#72615,#72616),(#72617,#72618),
(#72619,#72620)),.UNSPECIFIED.,.F.,.F.,.F.,(3,3),(2,2),(0.,1.),(0.,0.0172800000000002),
 .UNSPECIFIED.);
#498=B_SPLINE_SURFACE_WITH_KNOTS('',2,1,((#72630,#72631),(#72632,#72633),
(#72634,#72635)),.UNSPECIFIED.,.F.,.F.,.F.,(3,3),(2,2),(0.,1.),(0.,0.0172800000000002),
 .UNSPECIFIED.);
#499=B_SPLINE_SURFACE_WITH_KNOTS('',2,1,((#72645,#72646),(#72647,#72648),
(#72649,#72650)),.UNSPECIFIED.,.F.,.F.,.F.,(3,3),(2,2),(0.,1.),(0.,0.0172800000000002),
 .UNSPECIFIED.);
#500=B_SPLINE_SURFACE_WITH_KNOTS('',2,1,((#72667,#72668),(#72669,#72670),
(#72671,#72672)),.UNSPECIFIED.,.F.,.F.,.F.,(3,3),(2,2),(0.,1.),(0.,0.0172800000000002),
 .UNSPECIFIED.);
#501=B_SPLINE_SURFACE_WITH_KNOTS('',2,1,((#72682,#72683),(#72684,#72685),
(#72686,#72687)),.UNSPECIFIED.,.F.,.F.,.F.,(3,3),(2,2),(0.,1.),(0.,0.0172800000000002),
 .UNSPECIFIED.);
#502=B_SPLINE_SURFACE_WITH_KNOTS('',2,1,((#72703,#72704),(#72705,#72706),
(#72707,#72708)),.UNSPECIFIED.,.F.,.F.,.F.,(3,3),(2,2),(0.,1.),(0.,0.0172800000000002),
 .UNSPECIFIED.);
#503=B_SPLINE_SURFACE_WITH_KNOTS('',2,1,((#72718,#72719),(#72720,#72721),
(#72722,#72723)),.UNSPECIFIED.,.F.,.F.,.F.,(3,3),(2,2),(0.,1.),(0.,0.0172800000000002),
 .UNSPECIFIED.);
#504=B_SPLINE_SURFACE_WITH_KNOTS('',2,1,((#72750,#72751),(#72752,#72753),
(#72754,#72755)),.UNSPECIFIED.,.F.,.F.,.F.,(3,3),(2,2),(0.,1.),(0.,0.0172800000000002),
 .UNSPECIFIED.);
#505=B_SPLINE_SURFACE_WITH_KNOTS('',2,1,((#72768,#72769),(#72770,#72771),
(#72772,#72773)),.UNSPECIFIED.,.F.,.F.,.F.,(3,3),(2,2),(0.,1.),(0.,0.0172800000000002),
 .UNSPECIFIED.);
#506=B_SPLINE_SURFACE_WITH_KNOTS('',2,1,((#72783,#72784),(#72785,#72786),
(#72787,#72788)),.UNSPECIFIED.,.F.,.F.,.F.,(3,3),(2,2),(0.,1.),(0.,0.0172800000000002),
 .UNSPECIFIED.);
#507=B_SPLINE_SURFACE_WITH_KNOTS('',2,1,((#72798,#72799),(#72800,#72801),
(#72802,#72803)),.UNSPECIFIED.,.F.,.F.,.F.,(3,3),(2,2),(0.,1.),(0.,0.0172800000000002),
 .UNSPECIFIED.);
#508=B_SPLINE_SURFACE_WITH_KNOTS('',2,1,((#72813,#72814),(#72815,#72816),
(#72817,#72818)),.UNSPECIFIED.,.F.,.F.,.F.,(3,3),(2,2),(0.,1.),(0.,0.0172800000000002),
 .UNSPECIFIED.);
#509=B_SPLINE_SURFACE_WITH_KNOTS('',2,1,((#72828,#72829),(#72830,#72831),
(#72832,#72833)),.UNSPECIFIED.,.F.,.F.,.F.,(3,3),(2,2),(0.,1.),(0.,0.0172800000000002),
 .UNSPECIFIED.);
#510=B_SPLINE_SURFACE_WITH_KNOTS('',2,1,((#72843,#72844),(#72845,#72846),
(#72847,#72848)),.UNSPECIFIED.,.F.,.F.,.F.,(3,3),(2,2),(0.,1.),(0.,0.0172800000000002),
 .UNSPECIFIED.);
#511=B_SPLINE_SURFACE_WITH_KNOTS('',2,1,((#72858,#72859),(#72860,#72861),
(#72862,#72863)),.UNSPECIFIED.,.F.,.F.,.F.,(3,3),(2,2),(0.,1.),(0.,0.0172800000000002),
 .UNSPECIFIED.);
#512=B_SPLINE_SURFACE_WITH_KNOTS('',2,1,((#72870,#72871),(#72872,#72873),
(#72874,#72875)),.UNSPECIFIED.,.F.,.F.,.F.,(3,3),(2,2),(0.,1.),(0.,0.0172800000000002),
 .UNSPECIFIED.);
#513=B_SPLINE_SURFACE_WITH_KNOTS('',2,1,((#72888,#72889),(#72890,#72891),
(#72892,#72893)),.UNSPECIFIED.,.F.,.F.,.F.,(3,3),(2,2),(0.,1.),(0.,0.0172800000000002),
 .UNSPECIFIED.);
#514=B_SPLINE_SURFACE_WITH_KNOTS('',2,1,((#72903,#72904),(#72905,#72906),
(#72907,#72908)),.UNSPECIFIED.,.F.,.F.,.F.,(3,3),(2,2),(0.,1.),(0.,0.0172800000000002),
 .UNSPECIFIED.);
#515=B_SPLINE_SURFACE_WITH_KNOTS('',2,1,((#72918,#72919),(#72920,#72921),
(#72922,#72923)),.UNSPECIFIED.,.F.,.F.,.F.,(3,3),(2,2),(0.,1.),(0.,0.0172800000000002),
 .UNSPECIFIED.);
#516=B_SPLINE_SURFACE_WITH_KNOTS('',2,1,((#72933,#72934),(#72935,#72936),
(#72937,#72938)),.UNSPECIFIED.,.F.,.F.,.F.,(3,3),(2,2),(0.,1.),(0.,0.0172800000000002),
 .UNSPECIFIED.);
#517=B_SPLINE_SURFACE_WITH_KNOTS('',2,1,((#72948,#72949),(#72950,#72951),
(#72952,#72953)),.UNSPECIFIED.,.F.,.F.,.F.,(3,3),(2,2),(0.,1.),(0.,0.0172800000000002),
 .UNSPECIFIED.);
#518=B_SPLINE_SURFACE_WITH_KNOTS('',2,1,((#72963,#72964),(#72965,#72966),
(#72967,#72968)),.UNSPECIFIED.,.F.,.F.,.F.,(3,3),(2,2),(0.,1.),(0.,0.0172800000000002),
 .UNSPECIFIED.);
#519=B_SPLINE_SURFACE_WITH_KNOTS('',2,1,((#72978,#72979),(#72980,#72981),
(#72982,#72983)),.UNSPECIFIED.,.F.,.F.,.F.,(3,3),(2,2),(0.,1.),(0.,0.0172800000000002),
 .UNSPECIFIED.);
#520=B_SPLINE_SURFACE_WITH_KNOTS('',2,1,((#72993,#72994),(#72995,#72996),
(#72997,#72998)),.UNSPECIFIED.,.F.,.F.,.F.,(3,3),(2,2),(0.,1.),(0.,0.0172800000000002),
 .UNSPECIFIED.);
#521=B_SPLINE_SURFACE_WITH_KNOTS('',2,1,((#73008,#73009),(#73010,#73011),
(#73012,#73013)),.UNSPECIFIED.,.F.,.F.,.F.,(3,3),(2,2),(0.,1.),(0.,0.0172800000000002),
 .UNSPECIFIED.);
#522=B_SPLINE_SURFACE_WITH_KNOTS('',2,1,((#73023,#73024),(#73025,#73026),
(#73027,#73028)),.UNSPECIFIED.,.F.,.F.,.F.,(3,3),(2,2),(0.,1.),(0.,0.0172800000000002),
 .UNSPECIFIED.);
#523=B_SPLINE_SURFACE_WITH_KNOTS('',2,1,((#73038,#73039),(#73040,#73041),
(#73042,#73043)),.UNSPECIFIED.,.F.,.F.,.F.,(3,3),(2,2),(0.,1.),(0.,0.0172800000000002),
 .UNSPECIFIED.);
#524=B_SPLINE_SURFACE_WITH_KNOTS('',2,1,((#73051,#73052),(#73053,#73054),
(#73055,#73056)),.UNSPECIFIED.,.F.,.F.,.F.,(3,3),(2,2),(0.,1.),(0.,0.0172800000000002),
 .UNSPECIFIED.);
#525=B_SPLINE_SURFACE_WITH_KNOTS('',2,1,((#73069,#73070),(#73071,#73072),
(#73073,#73074)),.UNSPECIFIED.,.F.,.F.,.F.,(3,3),(2,2),(0.,1.),(0.,0.0172800000000002),
 .UNSPECIFIED.);
#526=B_SPLINE_SURFACE_WITH_KNOTS('',2,1,((#73084,#73085),(#73086,#73087),
(#73088,#73089)),.UNSPECIFIED.,.F.,.F.,.F.,(3,3),(2,2),(0.,1.),(0.,0.0172800000000002),
 .UNSPECIFIED.);
#527=B_SPLINE_SURFACE_WITH_KNOTS('',2,1,((#73099,#73100),(#73101,#73102),
(#73103,#73104)),.UNSPECIFIED.,.F.,.F.,.F.,(3,3),(2,2),(0.,1.),(0.,0.0172800000000002),
 .UNSPECIFIED.);
#528=B_SPLINE_SURFACE_WITH_KNOTS('',2,1,((#73114,#73115),(#73116,#73117),
(#73118,#73119)),.UNSPECIFIED.,.F.,.F.,.F.,(3,3),(2,2),(0.,1.),(0.,0.0172800000000002),
 .UNSPECIFIED.);
#529=B_SPLINE_SURFACE_WITH_KNOTS('',2,1,((#73129,#73130),(#73131,#73132),
(#73133,#73134)),.UNSPECIFIED.,.F.,.F.,.F.,(3,3),(2,2),(0.,1.),(0.,0.0172800000000002),
 .UNSPECIFIED.);
#530=B_SPLINE_SURFACE_WITH_KNOTS('',2,1,((#73144,#73145),(#73146,#73147),
(#73148,#73149)),.UNSPECIFIED.,.F.,.F.,.F.,(3,3),(2,2),(0.,1.),(0.,0.0172800000000002),
 .UNSPECIFIED.);
#531=B_SPLINE_SURFACE_WITH_KNOTS('',2,1,((#73159,#73160),(#73161,#73162),
(#73163,#73164)),.UNSPECIFIED.,.F.,.F.,.F.,(3,3),(2,2),(0.,1.),(0.,0.0172800000000002),
 .UNSPECIFIED.);
#532=B_SPLINE_SURFACE_WITH_KNOTS('',2,1,((#73174,#73175),(#73176,#73177),
(#73178,#73179)),.UNSPECIFIED.,.F.,.F.,.F.,(3,3),(2,2),(0.,1.),(0.,0.0172800000000002),
 .UNSPECIFIED.);
#533=B_SPLINE_SURFACE_WITH_KNOTS('',2,1,((#73195,#73196),(#73197,#73198),
(#73199,#73200)),.UNSPECIFIED.,.F.,.F.,.F.,(3,3),(2,2),(0.,1.),(0.,0.0172800000000002),
 .UNSPECIFIED.);
#534=B_SPLINE_SURFACE_WITH_KNOTS('',2,1,((#73210,#73211),(#73212,#73213),
(#73214,#73215)),.UNSPECIFIED.,.F.,.F.,.F.,(3,3),(2,2),(0.,1.),(0.,0.0172800000000002),
 .UNSPECIFIED.);
#535=B_SPLINE_SURFACE_WITH_KNOTS('',2,1,((#73225,#73226),(#73227,#73228),
(#73229,#73230)),.UNSPECIFIED.,.F.,.F.,.F.,(3,3),(2,2),(0.,1.),(0.,0.0172800000000002),
 .UNSPECIFIED.);
#536=B_SPLINE_SURFACE_WITH_KNOTS('',2,1,((#73240,#73241),(#73242,#73243),
(#73244,#73245)),.UNSPECIFIED.,.F.,.F.,.F.,(3,3),(2,2),(0.,1.),(0.,0.0172800000000002),
 .UNSPECIFIED.);
#537=B_SPLINE_SURFACE_WITH_KNOTS('',2,1,((#73255,#73256),(#73257,#73258),
(#73259,#73260)),.UNSPECIFIED.,.F.,.F.,.F.,(3,3),(2,2),(0.,1.),(0.,0.0172800000000002),
 .UNSPECIFIED.);
#538=B_SPLINE_SURFACE_WITH_KNOTS('',2,1,((#73270,#73271),(#73272,#73273),
(#73274,#73275)),.UNSPECIFIED.,.F.,.F.,.F.,(3,3),(2,2),(0.,1.),(0.,0.0172800000000002),
 .UNSPECIFIED.);
#539=B_SPLINE_SURFACE_WITH_KNOTS('',2,1,((#73285,#73286),(#73287,#73288),
(#73289,#73290)),.UNSPECIFIED.,.F.,.F.,.F.,(3,3),(2,2),(0.,1.),(0.,0.0172800000000002),
 .UNSPECIFIED.);
#540=B_SPLINE_SURFACE_WITH_KNOTS('',2,1,((#73300,#73301),(#73302,#73303),
(#73304,#73305)),.UNSPECIFIED.,.F.,.F.,.F.,(3,3),(2,2),(0.,1.),(0.,0.0172800000000002),
 .UNSPECIFIED.);
#541=B_SPLINE_SURFACE_WITH_KNOTS('',2,1,((#73315,#73316),(#73317,#73318),
(#73319,#73320)),.UNSPECIFIED.,.F.,.F.,.F.,(3,3),(2,2),(0.,1.),(0.,0.0172800000000002),
 .UNSPECIFIED.);
#542=B_SPLINE_SURFACE_WITH_KNOTS('',2,1,((#73347,#73348),(#73349,#73350),
(#73351,#73352)),.UNSPECIFIED.,.F.,.F.,.F.,(3,3),(2,2),(0.,1.),(0.,0.0172800000000002),
 .UNSPECIFIED.);
#543=B_SPLINE_SURFACE_WITH_KNOTS('',2,1,((#73365,#73366),(#73367,#73368),
(#73369,#73370)),.UNSPECIFIED.,.F.,.F.,.F.,(3,3),(2,2),(0.,1.),(0.,0.0172800000000002),
 .UNSPECIFIED.);
#544=B_SPLINE_SURFACE_WITH_KNOTS('',2,1,((#73380,#73381),(#73382,#73383),
(#73384,#73385)),.UNSPECIFIED.,.F.,.F.,.F.,(3,3),(2,2),(0.,1.),(0.,0.0172800000000002),
 .UNSPECIFIED.);
#545=B_SPLINE_SURFACE_WITH_KNOTS('',2,1,((#73395,#73396),(#73397,#73398),
(#73399,#73400)),.UNSPECIFIED.,.F.,.F.,.F.,(3,3),(2,2),(0.,1.),(0.,0.0172800000000002),
 .UNSPECIFIED.);
#546=B_SPLINE_SURFACE_WITH_KNOTS('',2,1,((#73410,#73411),(#73412,#73413),
(#73414,#73415)),.UNSPECIFIED.,.F.,.F.,.F.,(3,3),(2,2),(0.,1.),(0.,0.0172800000000002),
 .UNSPECIFIED.);
#547=B_SPLINE_SURFACE_WITH_KNOTS('',2,1,((#73425,#73426),(#73427,#73428),
(#73429,#73430)),.UNSPECIFIED.,.F.,.F.,.F.,(3,3),(2,2),(0.,1.),(0.,0.0172800000000002),
 .UNSPECIFIED.);
#548=B_SPLINE_SURFACE_WITH_KNOTS('',2,1,((#73440,#73441),(#73442,#73443),
(#73444,#73445)),.UNSPECIFIED.,.F.,.F.,.F.,(3,3),(2,2),(0.,1.),(0.,0.0172800000000002),
 .UNSPECIFIED.);
#549=B_SPLINE_SURFACE_WITH_KNOTS('',2,1,((#73455,#73456),(#73457,#73458),
(#73459,#73460)),.UNSPECIFIED.,.F.,.F.,.F.,(3,3),(2,2),(0.,1.),(0.,0.0172800000000002),
 .UNSPECIFIED.);
#550=B_SPLINE_SURFACE_WITH_KNOTS('',2,1,((#73467,#73468),(#73469,#73470),
(#73471,#73472)),.UNSPECIFIED.,.F.,.F.,.F.,(3,3),(2,2),(0.,1.),(0.,0.0172800000000002),
 .UNSPECIFIED.);
#551=B_SPLINE_SURFACE_WITH_KNOTS('',2,1,((#73485,#73486),(#73487,#73488),
(#73489,#73490)),.UNSPECIFIED.,.F.,.F.,.F.,(3,3),(2,2),(0.,1.),(0.,0.0172800000000002),
 .UNSPECIFIED.);
#552=B_SPLINE_SURFACE_WITH_KNOTS('',2,1,((#73500,#73501),(#73502,#73503),
(#73504,#73505)),.UNSPECIFIED.,.F.,.F.,.F.,(3,3),(2,2),(0.,1.),(0.,0.0172800000000002),
 .UNSPECIFIED.);
#553=B_SPLINE_SURFACE_WITH_KNOTS('',2,1,((#73515,#73516),(#73517,#73518),
(#73519,#73520)),.UNSPECIFIED.,.F.,.F.,.F.,(3,3),(2,2),(0.,1.),(0.,0.0172800000000002),
 .UNSPECIFIED.);
#554=B_SPLINE_SURFACE_WITH_KNOTS('',2,1,((#73530,#73531),(#73532,#73533),
(#73534,#73535)),.UNSPECIFIED.,.F.,.F.,.F.,(3,3),(2,2),(0.,1.),(0.,0.0172800000000002),
 .UNSPECIFIED.);
#555=B_SPLINE_SURFACE_WITH_KNOTS('',2,1,((#73545,#73546),(#73547,#73548),
(#73549,#73550)),.UNSPECIFIED.,.F.,.F.,.F.,(3,3),(2,2),(0.,1.),(0.,0.0172800000000002),
 .UNSPECIFIED.);
#556=B_SPLINE_SURFACE_WITH_KNOTS('',2,1,((#73560,#73561),(#73562,#73563),
(#73564,#73565)),.UNSPECIFIED.,.F.,.F.,.F.,(3,3),(2,2),(0.,1.),(0.,0.0172800000000002),
 .UNSPECIFIED.);
#557=B_SPLINE_SURFACE_WITH_KNOTS('',2,1,((#73575,#73576),(#73577,#73578),
(#73579,#73580)),.UNSPECIFIED.,.F.,.F.,.F.,(3,3),(2,2),(0.,1.),(0.,0.0172800000000002),
 .UNSPECIFIED.);
#558=B_SPLINE_SURFACE_WITH_KNOTS('',2,1,((#73590,#73591),(#73592,#73593),
(#73594,#73595)),.UNSPECIFIED.,.F.,.F.,.F.,(3,3),(2,2),(0.,1.),(0.,0.0172800000000002),
 .UNSPECIFIED.);
#559=B_SPLINE_SURFACE_WITH_KNOTS('',2,1,((#73605,#73606),(#73607,#73608),
(#73609,#73610)),.UNSPECIFIED.,.F.,.F.,.F.,(3,3),(2,2),(0.,1.),(0.,0.0172800000000002),
 .UNSPECIFIED.);
#560=B_SPLINE_SURFACE_WITH_KNOTS('',2,1,((#73620,#73621),(#73622,#73623),
(#73624,#73625)),.UNSPECIFIED.,.F.,.F.,.F.,(3,3),(2,2),(0.,1.),(0.,0.0172800000000002),
 .UNSPECIFIED.);
#561=B_SPLINE_SURFACE_WITH_KNOTS('',2,1,((#73635,#73636),(#73637,#73638),
(#73639,#73640)),.UNSPECIFIED.,.F.,.F.,.F.,(3,3),(2,2),(0.,1.),(0.,0.0172800000000002),
 .UNSPECIFIED.);
#562=B_SPLINE_SURFACE_WITH_KNOTS('',2,1,((#73648,#73649),(#73650,#73651),
(#73652,#73653)),.UNSPECIFIED.,.F.,.F.,.F.,(3,3),(2,2),(0.,1.),(0.,0.0172800000000002),
 .UNSPECIFIED.);
#563=B_SPLINE_SURFACE_WITH_KNOTS('',2,1,((#73666,#73667),(#73668,#73669),
(#73670,#73671)),.UNSPECIFIED.,.F.,.F.,.F.,(3,3),(2,2),(0.,1.),(0.,0.0172800000000002),
 .UNSPECIFIED.);
#564=B_SPLINE_SURFACE_WITH_KNOTS('',2,1,((#73681,#73682),(#73683,#73684),
(#73685,#73686)),.UNSPECIFIED.,.F.,.F.,.F.,(3,3),(2,2),(0.,1.),(0.,0.0172800000000002),
 .UNSPECIFIED.);
#565=B_SPLINE_SURFACE_WITH_KNOTS('',2,1,((#73696,#73697),(#73698,#73699),
(#73700,#73701)),.UNSPECIFIED.,.F.,.F.,.F.,(3,3),(2,2),(0.,1.),(0.,0.0172800000000002),
 .UNSPECIFIED.);
#566=B_SPLINE_SURFACE_WITH_KNOTS('',2,1,((#73711,#73712),(#73713,#73714),
(#73715,#73716)),.UNSPECIFIED.,.F.,.F.,.F.,(3,3),(2,2),(0.,1.),(0.,0.0172800000000002),
 .UNSPECIFIED.);
#567=B_SPLINE_SURFACE_WITH_KNOTS('',2,1,((#73726,#73727),(#73728,#73729),
(#73730,#73731)),.UNSPECIFIED.,.F.,.F.,.F.,(3,3),(2,2),(0.,1.),(0.,0.0172800000000002),
 .UNSPECIFIED.);
#568=B_SPLINE_SURFACE_WITH_KNOTS('',2,1,((#73741,#73742),(#73743,#73744),
(#73745,#73746)),.UNSPECIFIED.,.F.,.F.,.F.,(3,3),(2,2),(0.,1.),(0.,0.0172800000000002),
 .UNSPECIFIED.);
#569=B_SPLINE_SURFACE_WITH_KNOTS('',2,1,((#73756,#73757),(#73758,#73759),
(#73760,#73761)),.UNSPECIFIED.,.F.,.F.,.F.,(3,3),(2,2),(0.,1.),(0.,0.0172800000000002),
 .UNSPECIFIED.);
#570=B_SPLINE_SURFACE_WITH_KNOTS('',2,1,((#73771,#73772),(#73773,#73774),
(#73775,#73776)),.UNSPECIFIED.,.F.,.F.,.F.,(3,3),(2,2),(0.,1.),(0.,0.0172800000000002),
 .UNSPECIFIED.);
#571=B_SPLINE_SURFACE_WITH_KNOTS('',2,1,((#73786,#73787),(#73788,#73789),
(#73790,#73791)),.UNSPECIFIED.,.F.,.F.,.F.,(3,3),(2,2),(0.,1.),(0.,0.0172800000000002),
 .UNSPECIFIED.);
#572=B_SPLINE_SURFACE_WITH_KNOTS('',2,1,((#73801,#73802),(#73803,#73804),
(#73805,#73806)),.UNSPECIFIED.,.F.,.F.,.F.,(3,3),(2,2),(0.,1.),(0.,0.0172800000000002),
 .UNSPECIFIED.);
#573=B_SPLINE_SURFACE_WITH_KNOTS('',2,1,((#73816,#73817),(#73818,#73819),
(#73820,#73821)),.UNSPECIFIED.,.F.,.F.,.F.,(3,3),(2,2),(0.,1.),(0.,0.0172800000000002),
 .UNSPECIFIED.);
#574=B_SPLINE_SURFACE_WITH_KNOTS('',2,1,((#73837,#73838),(#73839,#73840),
(#73841,#73842)),.UNSPECIFIED.,.F.,.F.,.F.,(3,3),(2,2),(0.,1.),(0.,0.0172800000000002),
 .UNSPECIFIED.);
#575=B_SPLINE_SURFACE_WITH_KNOTS('',2,1,((#73852,#73853),(#73854,#73855),
(#73856,#73857)),.UNSPECIFIED.,.F.,.F.,.F.,(3,3),(2,2),(0.,1.),(0.,0.0172800000000002),
 .UNSPECIFIED.);
#576=B_SPLINE_SURFACE_WITH_KNOTS('',2,1,((#73867,#73868),(#73869,#73870),
(#73871,#73872)),.UNSPECIFIED.,.F.,.F.,.F.,(3,3),(2,2),(0.,1.),(0.,0.0172800000000002),
 .UNSPECIFIED.);
#577=B_SPLINE_SURFACE_WITH_KNOTS('',2,1,((#73882,#73883),(#73884,#73885),
(#73886,#73887)),.UNSPECIFIED.,.F.,.F.,.F.,(3,3),(2,2),(0.,1.),(0.,0.0172800000000002),
 .UNSPECIFIED.);
#578=B_SPLINE_SURFACE_WITH_KNOTS('',2,1,((#73897,#73898),(#73899,#73900),
(#73901,#73902)),.UNSPECIFIED.,.F.,.F.,.F.,(3,3),(2,2),(0.,1.),(0.,0.0172800000000002),
 .UNSPECIFIED.);
#579=B_SPLINE_SURFACE_WITH_KNOTS('',2,1,((#73912,#73913),(#73914,#73915),
(#73916,#73917)),.UNSPECIFIED.,.F.,.F.,.F.,(3,3),(2,2),(0.,1.),(0.,0.0172800000000002),
 .UNSPECIFIED.);
#580=B_SPLINE_SURFACE_WITH_KNOTS('',2,1,((#73927,#73928),(#73929,#73930),
(#73931,#73932)),.UNSPECIFIED.,.F.,.F.,.F.,(3,3),(2,2),(0.,1.),(0.,0.0172800000000002),
 .UNSPECIFIED.);
#581=B_SPLINE_SURFACE_WITH_KNOTS('',2,1,((#73948,#73949),(#73950,#73951),
(#73952,#73953)),.UNSPECIFIED.,.F.,.F.,.F.,(3,3),(2,2),(0.,1.),(0.,0.0172800000000002),
 .UNSPECIFIED.);
#582=B_SPLINE_SURFACE_WITH_KNOTS('',2,1,((#73963,#73964),(#73965,#73966),
(#73967,#73968)),.UNSPECIFIED.,.F.,.F.,.F.,(3,3),(2,2),(0.,1.),(0.,0.0172800000000002),
 .UNSPECIFIED.);
#583=B_SPLINE_SURFACE_WITH_KNOTS('',2,1,((#73978,#73979),(#73980,#73981),
(#73982,#73983)),.UNSPECIFIED.,.F.,.F.,.F.,(3,3),(2,2),(0.,1.),(0.,0.0172800000000002),
 .UNSPECIFIED.);
#584=B_SPLINE_SURFACE_WITH_KNOTS('',2,1,((#73993,#73994),(#73995,#73996),
(#73997,#73998)),.UNSPECIFIED.,.F.,.F.,.F.,(3,3),(2,2),(0.,1.),(0.,0.0172800000000002),
 .UNSPECIFIED.);
#585=B_SPLINE_SURFACE_WITH_KNOTS('',2,1,((#74008,#74009),(#74010,#74011),
(#74012,#74013)),.UNSPECIFIED.,.F.,.F.,.F.,(3,3),(2,2),(0.,1.),(0.,0.0172800000000002),
 .UNSPECIFIED.);
#586=B_SPLINE_SURFACE_WITH_KNOTS('',2,1,((#74023,#74024),(#74025,#74026),
(#74027,#74028)),.UNSPECIFIED.,.F.,.F.,.F.,(3,3),(2,2),(0.,1.),(0.,0.0172800000000002),
 .UNSPECIFIED.);
#587=B_SPLINE_SURFACE_WITH_KNOTS('',2,1,((#74038,#74039),(#74040,#74041),
(#74042,#74043)),.UNSPECIFIED.,.F.,.F.,.F.,(3,3),(2,2),(0.,1.),(0.,0.0172800000000002),
 .UNSPECIFIED.);
#588=B_SPLINE_SURFACE_WITH_KNOTS('',2,1,((#74059,#74060),(#74061,#74062),
(#74063,#74064)),.UNSPECIFIED.,.F.,.F.,.F.,(3,3),(2,2),(0.,1.),(0.,0.0172800000000002),
 .UNSPECIFIED.);
#589=B_SPLINE_SURFACE_WITH_KNOTS('',2,1,((#74073,#74074),(#74075,#74076),
(#74077,#74078)),.UNSPECIFIED.,.F.,.F.,.F.,(3,3),(2,2),(0.,1.),(0.,0.0172800000000002),
 .UNSPECIFIED.);
#590=B_SPLINE_SURFACE_WITH_KNOTS('',2,1,((#74091,#74092),(#74093,#74094),
(#74095,#74096)),.UNSPECIFIED.,.F.,.F.,.F.,(3,3),(2,2),(0.,1.),(0.,0.0172800000000002),
 .UNSPECIFIED.);
#591=B_SPLINE_SURFACE_WITH_KNOTS('',2,1,((#74106,#74107),(#74108,#74109),
(#74110,#74111)),.UNSPECIFIED.,.F.,.F.,.F.,(3,3),(2,2),(0.,1.),(0.,0.0172800000000002),
 .UNSPECIFIED.);
#592=B_SPLINE_SURFACE_WITH_KNOTS('',2,1,((#74121,#74122),(#74123,#74124),
(#74125,#74126)),.UNSPECIFIED.,.F.,.F.,.F.,(3,3),(2,2),(0.,1.),(0.,0.0172800000000002),
 .UNSPECIFIED.);
#593=B_SPLINE_SURFACE_WITH_KNOTS('',2,1,((#74136,#74137),(#74138,#74139),
(#74140,#74141)),.UNSPECIFIED.,.F.,.F.,.F.,(3,3),(2,2),(0.,1.),(0.,0.0172800000000002),
 .UNSPECIFIED.);
#594=B_SPLINE_SURFACE_WITH_KNOTS('',2,1,((#74151,#74152),(#74153,#74154),
(#74155,#74156)),.UNSPECIFIED.,.F.,.F.,.F.,(3,3),(2,2),(0.,1.),(0.,0.0172800000000002),
 .UNSPECIFIED.);
#595=B_SPLINE_SURFACE_WITH_KNOTS('',2,1,((#74166,#74167),(#74168,#74169),
(#74170,#74171)),.UNSPECIFIED.,.F.,.F.,.F.,(3,3),(2,2),(0.,1.),(0.,0.0172800000000002),
 .UNSPECIFIED.);
#596=B_SPLINE_SURFACE_WITH_KNOTS('',2,1,((#74181,#74182),(#74183,#74184),
(#74185,#74186)),.UNSPECIFIED.,.F.,.F.,.F.,(3,3),(2,2),(0.,1.),(0.,0.0172800000000002),
 .UNSPECIFIED.);
#597=B_SPLINE_SURFACE_WITH_KNOTS('',2,1,((#74193,#74194),(#74195,#74196),
(#74197,#74198)),.UNSPECIFIED.,.F.,.F.,.F.,(3,3),(2,2),(0.,1.),(0.,0.0172800000000002),
 .UNSPECIFIED.);
#598=B_SPLINE_SURFACE_WITH_KNOTS('',2,1,((#74211,#74212),(#74213,#74214),
(#74215,#74216)),.UNSPECIFIED.,.F.,.F.,.F.,(3,3),(2,2),(0.,1.),(0.,0.0172800000000002),
 .UNSPECIFIED.);
#599=B_SPLINE_SURFACE_WITH_KNOTS('',2,1,((#74226,#74227),(#74228,#74229),
(#74230,#74231)),.UNSPECIFIED.,.F.,.F.,.F.,(3,3),(2,2),(0.,1.),(0.,0.0172800000000002),
 .UNSPECIFIED.);
#600=B_SPLINE_SURFACE_WITH_KNOTS('',2,1,((#74241,#74242),(#74243,#74244),
(#74245,#74246)),.UNSPECIFIED.,.F.,.F.,.F.,(3,3),(2,2),(0.,1.),(0.,0.0172800000000002),
 .UNSPECIFIED.);
#601=B_SPLINE_SURFACE_WITH_KNOTS('',2,1,((#74256,#74257),(#74258,#74259),
(#74260,#74261)),.UNSPECIFIED.,.F.,.F.,.F.,(3,3),(2,2),(0.,1.),(0.,0.0172800000000002),
 .UNSPECIFIED.);
#602=B_SPLINE_SURFACE_WITH_KNOTS('',2,1,((#74271,#74272),(#74273,#74274),
(#74275,#74276)),.UNSPECIFIED.,.F.,.F.,.F.,(3,3),(2,2),(0.,1.),(0.,0.0172800000000002),
 .UNSPECIFIED.);
#603=B_SPLINE_SURFACE_WITH_KNOTS('',2,1,((#74286,#74287),(#74288,#74289),
(#74290,#74291)),.UNSPECIFIED.,.F.,.F.,.F.,(3,3),(2,2),(0.,1.),(0.,0.0172800000000002),
 .UNSPECIFIED.);
#604=B_SPLINE_SURFACE_WITH_KNOTS('',2,1,((#74301,#74302),(#74303,#74304),
(#74305,#74306)),.UNSPECIFIED.,.F.,.F.,.F.,(3,3),(2,2),(0.,1.),(0.,0.0172800000000002),
 .UNSPECIFIED.);
#605=B_SPLINE_SURFACE_WITH_KNOTS('',2,1,((#74316,#74317),(#74318,#74319),
(#74320,#74321)),.UNSPECIFIED.,.F.,.F.,.F.,(3,3),(2,2),(0.,1.),(0.,0.0172800000000002),
 .UNSPECIFIED.);
#606=B_SPLINE_SURFACE_WITH_KNOTS('',2,1,((#74331,#74332),(#74333,#74334),
(#74335,#74336)),.UNSPECIFIED.,.F.,.F.,.F.,(3,3),(2,2),(0.,1.),(0.,0.0172800000000002),
 .UNSPECIFIED.);
#607=B_SPLINE_SURFACE_WITH_KNOTS('',2,1,((#74346,#74347),(#74348,#74349),
(#74350,#74351)),.UNSPECIFIED.,.F.,.F.,.F.,(3,3),(2,2),(0.,1.),(0.,0.0172800000000002),
 .UNSPECIFIED.);
#608=B_SPLINE_SURFACE_WITH_KNOTS('',2,1,((#74361,#74362),(#74363,#74364),
(#74365,#74366)),.UNSPECIFIED.,.F.,.F.,.F.,(3,3),(2,2),(0.,1.),(0.,0.0172800000000002),
 .UNSPECIFIED.);
#820=B_SPLINE_CURVE_WITH_KNOTS('',2,(#69959,#69960,#69961),
 .UNSPECIFIED.,.F.,.F.,(3,3),(0.,1.),.UNSPECIFIED.);
#821=B_SPLINE_CURVE_WITH_KNOTS('',2,(#69965,#69966,#69967),
 .UNSPECIFIED.,.F.,.F.,(3,3),(0.,1.),.UNSPECIFIED.);
#822=B_SPLINE_CURVE_WITH_KNOTS('',2,(#69976,#69977,#69978),
 .UNSPECIFIED.,.F.,.F.,(3,3),(0.,1.),.UNSPECIFIED.);
#823=B_SPLINE_CURVE_WITH_KNOTS('',2,(#69981,#69982,#69983),
 .UNSPECIFIED.,.F.,.F.,(3,3),(0.,1.),.UNSPECIFIED.);
#824=B_SPLINE_CURVE_WITH_KNOTS('',2,(#69991,#69992,#69993),
 .UNSPECIFIED.,.F.,.F.,(3,3),(0.,1.),.UNSPECIFIED.);
#825=B_SPLINE_CURVE_WITH_KNOTS('',2,(#69996,#69997,#69998),
 .UNSPECIFIED.,.F.,.F.,(3,3),(0.,1.),.UNSPECIFIED.);
#826=B_SPLINE_CURVE_WITH_KNOTS('',2,(#70006,#70007,#70008),
 .UNSPECIFIED.,.F.,.F.,(3,3),(0.,1.),.UNSPECIFIED.);
#827=B_SPLINE_CURVE_WITH_KNOTS('',2,(#70011,#70012,#70013),
 .UNSPECIFIED.,.F.,.F.,(3,3),(0.,1.),.UNSPECIFIED.);
#828=B_SPLINE_CURVE_WITH_KNOTS('',2,(#70021,#70022,#70023),
 .UNSPECIFIED.,.F.,.F.,(3,3),(0.,1.),.UNSPECIFIED.);
#829=B_SPLINE_CURVE_WITH_KNOTS('',2,(#70026,#70027,#70028),
 .UNSPECIFIED.,.F.,.F.,(3,3),(0.,1.),.UNSPECIFIED.);
#830=B_SPLINE_CURVE_WITH_KNOTS('',2,(#70036,#70037,#70038),
 .UNSPECIFIED.,.F.,.F.,(3,3),(0.,1.),.UNSPECIFIED.);
#831=B_SPLINE_CURVE_WITH_KNOTS('',2,(#70041,#70042,#70043),
 .UNSPECIFIED.,.F.,.F.,(3,3),(0.,1.),.UNSPECIFIED.);
#832=B_SPLINE_CURVE_WITH_KNOTS('',2,(#70051,#70052,#70053),
 .UNSPECIFIED.,.F.,.F.,(3,3),(0.,1.),.UNSPECIFIED.);
#833=B_SPLINE_CURVE_WITH_KNOTS('',2,(#70056,#70057,#70058),
 .UNSPECIFIED.,.F.,.F.,(3,3),(0.,1.),.UNSPECIFIED.);
#834=B_SPLINE_CURVE_WITH_KNOTS('',2,(#70065,#70066,#70067),
 .UNSPECIFIED.,.F.,.F.,(3,3),(0.,1.),.UNSPECIFIED.);
#835=B_SPLINE_CURVE_WITH_KNOTS('',2,(#70068,#70069,#70070),
 .UNSPECIFIED.,.F.,.F.,(3,3),(0.,1.),.UNSPECIFIED.);
#836=B_SPLINE_CURVE_WITH_KNOTS('',2,(#70079,#70080,#70081),
 .UNSPECIFIED.,.F.,.F.,(3,3),(0.,1.),.UNSPECIFIED.);
#837=B_SPLINE_CURVE_WITH_KNOTS('',2,(#70085,#70086,#70087),
 .UNSPECIFIED.,.F.,.F.,(3,3),(0.,1.),.UNSPECIFIED.);
#838=B_SPLINE_CURVE_WITH_KNOTS('',2,(#70096,#70097,#70098),
 .UNSPECIFIED.,.F.,.F.,(3,3),(0.,1.),.UNSPECIFIED.);
#839=B_SPLINE_CURVE_WITH_KNOTS('',2,(#70101,#70102,#70103),
 .UNSPECIFIED.,.F.,.F.,(3,3),(0.,1.),.UNSPECIFIED.);
#840=B_SPLINE_CURVE_WITH_KNOTS('',2,(#70111,#70112,#70113),
 .UNSPECIFIED.,.F.,.F.,(3,3),(0.,1.),.UNSPECIFIED.);
#841=B_SPLINE_CURVE_WITH_KNOTS('',2,(#70116,#70117,#70118),
 .UNSPECIFIED.,.F.,.F.,(3,3),(0.,1.),.UNSPECIFIED.);
#842=B_SPLINE_CURVE_WITH_KNOTS('',2,(#70126,#70127,#70128),
 .UNSPECIFIED.,.F.,.F.,(3,3),(0.,1.),.UNSPECIFIED.);
#843=B_SPLINE_CURVE_WITH_KNOTS('',2,(#70131,#70132,#70133),
 .UNSPECIFIED.,.F.,.F.,(3,3),(0.,1.),.UNSPECIFIED.);
#844=B_SPLINE_CURVE_WITH_KNOTS('',2,(#70141,#70142,#70143),
 .UNSPECIFIED.,.F.,.F.,(3,3),(0.,1.),.UNSPECIFIED.);
#845=B_SPLINE_CURVE_WITH_KNOTS('',2,(#70146,#70147,#70148),
 .UNSPECIFIED.,.F.,.F.,(3,3),(0.,1.),.UNSPECIFIED.);
#846=B_SPLINE_CURVE_WITH_KNOTS('',2,(#70156,#70157,#70158),
 .UNSPECIFIED.,.F.,.F.,(3,3),(0.,1.),.UNSPECIFIED.);
#847=B_SPLINE_CURVE_WITH_KNOTS('',2,(#70161,#70162,#70163),
 .UNSPECIFIED.,.F.,.F.,(3,3),(0.,1.),.UNSPECIFIED.);
#848=B_SPLINE_CURVE_WITH_KNOTS('',2,(#70171,#70172,#70173),
 .UNSPECIFIED.,.F.,.F.,(3,3),(0.,1.),.UNSPECIFIED.);
#849=B_SPLINE_CURVE_WITH_KNOTS('',2,(#70176,#70177,#70178),
 .UNSPECIFIED.,.F.,.F.,(3,3),(0.,1.),.UNSPECIFIED.);
#850=B_SPLINE_CURVE_WITH_KNOTS('',2,(#70186,#70187,#70188),
 .UNSPECIFIED.,.F.,.F.,(3,3),(0.,1.),.UNSPECIFIED.);
#851=B_SPLINE_CURVE_WITH_KNOTS('',2,(#70191,#70192,#70193),
 .UNSPECIFIED.,.F.,.F.,(3,3),(0.,1.),.UNSPECIFIED.);
#852=B_SPLINE_CURVE_WITH_KNOTS('',2,(#70201,#70202,#70203),
 .UNSPECIFIED.,.F.,.F.,(3,3),(0.,1.),.UNSPECIFIED.);
#853=B_SPLINE_CURVE_WITH_KNOTS('',2,(#70206,#70207,#70208),
 .UNSPECIFIED.,.F.,.F.,(3,3),(0.,1.),.UNSPECIFIED.);
#854=B_SPLINE_CURVE_WITH_KNOTS('',2,(#70216,#70217,#70218),
 .UNSPECIFIED.,.F.,.F.,(3,3),(0.,1.),.UNSPECIFIED.);
#855=B_SPLINE_CURVE_WITH_KNOTS('',2,(#70221,#70222,#70223),
 .UNSPECIFIED.,.F.,.F.,(3,3),(0.,1.),.UNSPECIFIED.);
#856=B_SPLINE_CURVE_WITH_KNOTS('',2,(#70231,#70232,#70233),
 .UNSPECIFIED.,.F.,.F.,(3,3),(0.,1.),.UNSPECIFIED.);
#857=B_SPLINE_CURVE_WITH_KNOTS('',2,(#70236,#70237,#70238),
 .UNSPECIFIED.,.F.,.F.,(3,3),(0.,1.),.UNSPECIFIED.);
#858=B_SPLINE_CURVE_WITH_KNOTS('',2,(#70245,#70246,#70247),
 .UNSPECIFIED.,.F.,.F.,(3,3),(0.,1.),.UNSPECIFIED.);
#859=B_SPLINE_CURVE_WITH_KNOTS('',2,(#70248,#70249,#70250),
 .UNSPECIFIED.,.F.,.F.,(3,3),(0.,1.),.UNSPECIFIED.);
#860=B_SPLINE_CURVE_WITH_KNOTS('',2,(#70347,#70348,#70349),
 .UNSPECIFIED.,.F.,.F.,(3,3),(0.,1.),.UNSPECIFIED.);
#861=B_SPLINE_CURVE_WITH_KNOTS('',2,(#70353,#70354,#70355),
 .UNSPECIFIED.,.F.,.F.,(3,3),(0.,1.),.UNSPECIFIED.);
#862=B_SPLINE_CURVE_WITH_KNOTS('',2,(#70364,#70365,#70366),
 .UNSPECIFIED.,.F.,.F.,(3,3),(0.,1.),.UNSPECIFIED.);
#863=B_SPLINE_CURVE_WITH_KNOTS('',2,(#70369,#70370,#70371),
 .UNSPECIFIED.,.F.,.F.,(3,3),(0.,1.),.UNSPECIFIED.);
#864=B_SPLINE_CURVE_WITH_KNOTS('',2,(#70379,#70380,#70381),
 .UNSPECIFIED.,.F.,.F.,(3,3),(0.,1.),.UNSPECIFIED.);
#865=B_SPLINE_CURVE_WITH_KNOTS('',2,(#70384,#70385,#70386),
 .UNSPECIFIED.,.F.,.F.,(3,3),(0.,1.),.UNSPECIFIED.);
#866=B_SPLINE_CURVE_WITH_KNOTS('',2,(#70394,#70395,#70396),
 .UNSPECIFIED.,.F.,.F.,(3,3),(0.,1.),.UNSPECIFIED.);
#867=B_SPLINE_CURVE_WITH_KNOTS('',2,(#70399,#70400,#70401),
 .UNSPECIFIED.,.F.,.F.,(3,3),(0.,1.),.UNSPECIFIED.);
#868=B_SPLINE_CURVE_WITH_KNOTS('',2,(#70409,#70410,#70411),
 .UNSPECIFIED.,.F.,.F.,(3,3),(0.,1.),.UNSPECIFIED.);
#869=B_SPLINE_CURVE_WITH_KNOTS('',2,(#70414,#70415,#70416),
 .UNSPECIFIED.,.F.,.F.,(3,3),(0.,1.),.UNSPECIFIED.);
#870=B_SPLINE_CURVE_WITH_KNOTS('',2,(#70424,#70425,#70426),
 .UNSPECIFIED.,.F.,.F.,(3,3),(0.,1.),.UNSPECIFIED.);
#871=B_SPLINE_CURVE_WITH_KNOTS('',2,(#70429,#70430,#70431),
 .UNSPECIFIED.,.F.,.F.,(3,3),(0.,1.),.UNSPECIFIED.);
#872=B_SPLINE_CURVE_WITH_KNOTS('',2,(#70439,#70440,#70441),
 .UNSPECIFIED.,.F.,.F.,(3,3),(0.,1.),.UNSPECIFIED.);
#873=B_SPLINE_CURVE_WITH_KNOTS('',2,(#70444,#70445,#70446),
 .UNSPECIFIED.,.F.,.F.,(3,3),(0.,1.),.UNSPECIFIED.);
#874=B_SPLINE_CURVE_WITH_KNOTS('',2,(#70453,#70454,#70455),
 .UNSPECIFIED.,.F.,.F.,(3,3),(0.,1.),.UNSPECIFIED.);
#875=B_SPLINE_CURVE_WITH_KNOTS('',2,(#70456,#70457,#70458),
 .UNSPECIFIED.,.F.,.F.,(3,3),(0.,1.),.UNSPECIFIED.);
#876=B_SPLINE_CURVE_WITH_KNOTS('',2,(#70467,#70468,#70469),
 .UNSPECIFIED.,.F.,.F.,(3,3),(0.,1.),.UNSPECIFIED.);
#877=B_SPLINE_CURVE_WITH_KNOTS('',2,(#70473,#70474,#70475),
 .UNSPECIFIED.,.F.,.F.,(3,3),(0.,1.),.UNSPECIFIED.);
#878=B_SPLINE_CURVE_WITH_KNOTS('',2,(#70484,#70485,#70486),
 .UNSPECIFIED.,.F.,.F.,(3,3),(0.,1.),.UNSPECIFIED.);
#879=B_SPLINE_CURVE_WITH_KNOTS('',2,(#70489,#70490,#70491),
 .UNSPECIFIED.,.F.,.F.,(3,3),(0.,1.),.UNSPECIFIED.);
#880=B_SPLINE_CURVE_WITH_KNOTS('',2,(#70499,#70500,#70501),
 .UNSPECIFIED.,.F.,.F.,(3,3),(0.,1.),.UNSPECIFIED.);
#881=B_SPLINE_CURVE_WITH_KNOTS('',2,(#70504,#70505,#70506),
 .UNSPECIFIED.,.F.,.F.,(3,3),(0.,1.),.UNSPECIFIED.);
#882=B_SPLINE_CURVE_WITH_KNOTS('',2,(#70514,#70515,#70516),
 .UNSPECIFIED.,.F.,.F.,(3,3),(0.,1.),.UNSPECIFIED.);
#883=B_SPLINE_CURVE_WITH_KNOTS('',2,(#70519,#70520,#70521),
 .UNSPECIFIED.,.F.,.F.,(3,3),(0.,1.),.UNSPECIFIED.);
#884=B_SPLINE_CURVE_WITH_KNOTS('',2,(#70529,#70530,#70531),
 .UNSPECIFIED.,.F.,.F.,(3,3),(0.,1.),.UNSPECIFIED.);
#885=B_SPLINE_CURVE_WITH_KNOTS('',2,(#70534,#70535,#70536),
 .UNSPECIFIED.,.F.,.F.,(3,3),(0.,1.),.UNSPECIFIED.);
#886=B_SPLINE_CURVE_WITH_KNOTS('',2,(#70544,#70545,#70546),
 .UNSPECIFIED.,.F.,.F.,(3,3),(0.,1.),.UNSPECIFIED.);
#887=B_SPLINE_CURVE_WITH_KNOTS('',2,(#70549,#70550,#70551),
 .UNSPECIFIED.,.F.,.F.,(3,3),(0.,1.),.UNSPECIFIED.);
#888=B_SPLINE_CURVE_WITH_KNOTS('',2,(#70559,#70560,#70561),
 .UNSPECIFIED.,.F.,.F.,(3,3),(0.,1.),.UNSPECIFIED.);
#889=B_SPLINE_CURVE_WITH_KNOTS('',2,(#70564,#70565,#70566),
 .UNSPECIFIED.,.F.,.F.,(3,3),(0.,1.),.UNSPECIFIED.);
#890=B_SPLINE_CURVE_WITH_KNOTS('',2,(#70574,#70575,#70576),
 .UNSPECIFIED.,.F.,.F.,(3,3),(0.,1.),.UNSPECIFIED.);
#891=B_SPLINE_CURVE_WITH_KNOTS('',2,(#70579,#70580,#70581),
 .UNSPECIFIED.,.F.,.F.,(3,3),(0.,1.),.UNSPECIFIED.);
#892=B_SPLINE_CURVE_WITH_KNOTS('',2,(#70589,#70590,#70591),
 .UNSPECIFIED.,.F.,.F.,(3,3),(0.,1.),.UNSPECIFIED.);
#893=B_SPLINE_CURVE_WITH_KNOTS('',2,(#70594,#70595,#70596),
 .UNSPECIFIED.,.F.,.F.,(3,3),(0.,1.),.UNSPECIFIED.);
#894=B_SPLINE_CURVE_WITH_KNOTS('',2,(#70604,#70605,#70606),
 .UNSPECIFIED.,.F.,.F.,(3,3),(0.,1.),.UNSPECIFIED.);
#895=B_SPLINE_CURVE_WITH_KNOTS('',2,(#70609,#70610,#70611),
 .UNSPECIFIED.,.F.,.F.,(3,3),(0.,1.),.UNSPECIFIED.);
#896=B_SPLINE_CURVE_WITH_KNOTS('',2,(#70619,#70620,#70621),
 .UNSPECIFIED.,.F.,.F.,(3,3),(0.,1.),.UNSPECIFIED.);
#897=B_SPLINE_CURVE_WITH_KNOTS('',2,(#70624,#70625,#70626),
 .UNSPECIFIED.,.F.,.F.,(3,3),(0.,1.),.UNSPECIFIED.);
#898=B_SPLINE_CURVE_WITH_KNOTS('',2,(#70633,#70634,#70635),
 .UNSPECIFIED.,.F.,.F.,(3,3),(0.,1.),.UNSPECIFIED.);
#899=B_SPLINE_CURVE_WITH_KNOTS('',2,(#70636,#70637,#70638),
 .UNSPECIFIED.,.F.,.F.,(3,3),(0.,1.),.UNSPECIFIED.);
#900=B_SPLINE_CURVE_WITH_KNOTS('',2,(#70648,#70649,#70650),
 .UNSPECIFIED.,.F.,.F.,(3,3),(0.,1.),.UNSPECIFIED.);
#901=B_SPLINE_CURVE_WITH_KNOTS('',2,(#70654,#70655,#70656),
 .UNSPECIFIED.,.F.,.F.,(3,3),(0.,1.),.UNSPECIFIED.);
#902=B_SPLINE_CURVE_WITH_KNOTS('',2,(#70665,#70666,#70667),
 .UNSPECIFIED.,.F.,.F.,(3,3),(0.,1.),.UNSPECIFIED.);
#903=B_SPLINE_CURVE_WITH_KNOTS('',2,(#70670,#70671,#70672),
 .UNSPECIFIED.,.F.,.F.,(3,3),(0.,1.),.UNSPECIFIED.);
#904=B_SPLINE_CURVE_WITH_KNOTS('',2,(#70680,#70681,#70682),
 .UNSPECIFIED.,.F.,.F.,(3,3),(0.,1.),.UNSPECIFIED.);
#905=B_SPLINE_CURVE_WITH_KNOTS('',2,(#70685,#70686,#70687),
 .UNSPECIFIED.,.F.,.F.,(3,3),(0.,1.),.UNSPECIFIED.);
#906=B_SPLINE_CURVE_WITH_KNOTS('',2,(#70695,#70696,#70697),
 .UNSPECIFIED.,.F.,.F.,(3,3),(0.,1.),.UNSPECIFIED.);
#907=B_SPLINE_CURVE_WITH_KNOTS('',2,(#70700,#70701,#70702),
 .UNSPECIFIED.,.F.,.F.,(3,3),(0.,1.),.UNSPECIFIED.);
#908=B_SPLINE_CURVE_WITH_KNOTS('',2,(#70710,#70711,#70712),
 .UNSPECIFIED.,.F.,.F.,(3,3),(0.,1.),.UNSPECIFIED.);
#909=B_SPLINE_CURVE_WITH_KNOTS('',2,(#70715,#70716,#70717),
 .UNSPECIFIED.,.F.,.F.,(3,3),(0.,1.),.UNSPECIFIED.);
#910=B_SPLINE_CURVE_WITH_KNOTS('',2,(#70725,#70726,#70727),
 .UNSPECIFIED.,.F.,.F.,(3,3),(0.,1.),.UNSPECIFIED.);
#911=B_SPLINE_CURVE_WITH_KNOTS('',2,(#70730,#70731,#70732),
 .UNSPECIFIED.,.F.,.F.,(3,3),(0.,1.),.UNSPECIFIED.);
#912=B_SPLINE_CURVE_WITH_KNOTS('',2,(#70740,#70741,#70742),
 .UNSPECIFIED.,.F.,.F.,(3,3),(0.,1.),.UNSPECIFIED.);
#913=B_SPLINE_CURVE_WITH_KNOTS('',2,(#70745,#70746,#70747),
 .UNSPECIFIED.,.F.,.F.,(3,3),(0.,1.),.UNSPECIFIED.);
#914=B_SPLINE_CURVE_WITH_KNOTS('',2,(#70755,#70756,#70757),
 .UNSPECIFIED.,.F.,.F.,(3,3),(0.,1.),.UNSPECIFIED.);
#915=B_SPLINE_CURVE_WITH_KNOTS('',2,(#70760,#70761,#70762),
 .UNSPECIFIED.,.F.,.F.,(3,3),(0.,1.),.UNSPECIFIED.);
#916=B_SPLINE_CURVE_WITH_KNOTS('',2,(#70770,#70771,#70772),
 .UNSPECIFIED.,.F.,.F.,(3,3),(0.,1.),.UNSPECIFIED.);
#917=B_SPLINE_CURVE_WITH_KNOTS('',2,(#70775,#70776,#70777),
 .UNSPECIFIED.,.F.,.F.,(3,3),(0.,1.),.UNSPECIFIED.);
#918=B_SPLINE_CURVE_WITH_KNOTS('',2,(#70785,#70786,#70787),
 .UNSPECIFIED.,.F.,.F.,(3,3),(0.,1.),.UNSPECIFIED.);
#919=B_SPLINE_CURVE_WITH_KNOTS('',2,(#70790,#70791,#70792),
 .UNSPECIFIED.,.F.,.F.,(3,3),(0.,1.),.UNSPECIFIED.);
#920=B_SPLINE_CURVE_WITH_KNOTS('',2,(#70800,#70801,#70802),
 .UNSPECIFIED.,.F.,.F.,(3,3),(0.,1.),.UNSPECIFIED.);
#921=B_SPLINE_CURVE_WITH_KNOTS('',2,(#70805,#70806,#70807),
 .UNSPECIFIED.,.F.,.F.,(3,3),(0.,1.),.UNSPECIFIED.);
#922=B_SPLINE_CURVE_WITH_KNOTS('',2,(#70815,#70816,#70817),
 .UNSPECIFIED.,.F.,.F.,(3,3),(0.,1.),.UNSPECIFIED.);
#923=B_SPLINE_CURVE_WITH_KNOTS('',2,(#70820,#70821,#70822),
 .UNSPECIFIED.,.F.,.F.,(3,3),(0.,1.),.UNSPECIFIED.);
#924=B_SPLINE_CURVE_WITH_KNOTS('',2,(#70836,#70837,#70838),
 .UNSPECIFIED.,.F.,.F.,(3,3),(0.,1.),.UNSPECIFIED.);
#925=B_SPLINE_CURVE_WITH_KNOTS('',2,(#70841,#70842,#70843),
 .UNSPECIFIED.,.F.,.F.,(3,3),(0.,1.),.UNSPECIFIED.);
#926=B_SPLINE_CURVE_WITH_KNOTS('',2,(#70851,#70852,#70853),
 .UNSPECIFIED.,.F.,.F.,(3,3),(0.,1.),.UNSPECIFIED.);
#927=B_SPLINE_CURVE_WITH_KNOTS('',2,(#70856,#70857,#70858),
 .UNSPECIFIED.,.F.,.F.,(3,3),(0.,1.),.UNSPECIFIED.);
#928=B_SPLINE_CURVE_WITH_KNOTS('',2,(#70866,#70867,#70868),
 .UNSPECIFIED.,.F.,.F.,(3,3),(0.,1.),.UNSPECIFIED.);
#929=B_SPLINE_CURVE_WITH_KNOTS('',2,(#70871,#70872,#70873),
 .UNSPECIFIED.,.F.,.F.,(3,3),(0.,1.),.UNSPECIFIED.);
#930=B_SPLINE_CURVE_WITH_KNOTS('',2,(#70881,#70882,#70883),
 .UNSPECIFIED.,.F.,.F.,(3,3),(0.,1.),.UNSPECIFIED.);
#931=B_SPLINE_CURVE_WITH_KNOTS('',2,(#70886,#70887,#70888),
 .UNSPECIFIED.,.F.,.F.,(3,3),(0.,1.),.UNSPECIFIED.);
#932=B_SPLINE_CURVE_WITH_KNOTS('',2,(#70896,#70897,#70898),
 .UNSPECIFIED.,.F.,.F.,(3,3),(0.,1.),.UNSPECIFIED.);
#933=B_SPLINE_CURVE_WITH_KNOTS('',2,(#70901,#70902,#70903),
 .UNSPECIFIED.,.F.,.F.,(3,3),(0.,1.),.UNSPECIFIED.);
#934=B_SPLINE_CURVE_WITH_KNOTS('',2,(#70911,#70912,#70913),
 .UNSPECIFIED.,.F.,.F.,(3,3),(0.,1.),.UNSPECIFIED.);
#935=B_SPLINE_CURVE_WITH_KNOTS('',2,(#70916,#70917,#70918),
 .UNSPECIFIED.,.F.,.F.,(3,3),(0.,1.),.UNSPECIFIED.);
#936=B_SPLINE_CURVE_WITH_KNOTS('',2,(#70926,#70927,#70928),
 .UNSPECIFIED.,.F.,.F.,(3,3),(0.,1.),.UNSPECIFIED.);
#937=B_SPLINE_CURVE_WITH_KNOTS('',2,(#70931,#70932,#70933),
 .UNSPECIFIED.,.F.,.F.,(3,3),(0.,1.),.UNSPECIFIED.);
#938=B_SPLINE_CURVE_WITH_KNOTS('',2,(#70947,#70948,#70949),
 .UNSPECIFIED.,.F.,.F.,(3,3),(0.,1.),.UNSPECIFIED.);
#939=B_SPLINE_CURVE_WITH_KNOTS('',2,(#70952,#70953,#70954),
 .UNSPECIFIED.,.F.,.F.,(3,3),(0.,1.),.UNSPECIFIED.);
#940=B_SPLINE_CURVE_WITH_KNOTS('',2,(#70962,#70963,#70964),
 .UNSPECIFIED.,.F.,.F.,(3,3),(0.,1.),.UNSPECIFIED.);
#941=B_SPLINE_CURVE_WITH_KNOTS('',2,(#70967,#70968,#70969),
 .UNSPECIFIED.,.F.,.F.,(3,3),(0.,1.),.UNSPECIFIED.);
#942=B_SPLINE_CURVE_WITH_KNOTS('',2,(#70977,#70978,#70979),
 .UNSPECIFIED.,.F.,.F.,(3,3),(0.,1.),.UNSPECIFIED.);
#943=B_SPLINE_CURVE_WITH_KNOTS('',2,(#70982,#70983,#70984),
 .UNSPECIFIED.,.F.,.F.,(3,3),(0.,1.),.UNSPECIFIED.);
#944=B_SPLINE_CURVE_WITH_KNOTS('',2,(#70992,#70993,#70994),
 .UNSPECIFIED.,.F.,.F.,(3,3),(0.,1.),.UNSPECIFIED.);
#945=B_SPLINE_CURVE_WITH_KNOTS('',2,(#70997,#70998,#70999),
 .UNSPECIFIED.,.F.,.F.,(3,3),(0.,1.),.UNSPECIFIED.);
#946=B_SPLINE_CURVE_WITH_KNOTS('',2,(#71007,#71008,#71009),
 .UNSPECIFIED.,.F.,.F.,(3,3),(0.,1.),.UNSPECIFIED.);
#947=B_SPLINE_CURVE_WITH_KNOTS('',2,(#71012,#71013,#71014),
 .UNSPECIFIED.,.F.,.F.,(3,3),(0.,1.),.UNSPECIFIED.);
#948=B_SPLINE_CURVE_WITH_KNOTS('',2,(#71022,#71023,#71024),
 .UNSPECIFIED.,.F.,.F.,(3,3),(0.,1.),.UNSPECIFIED.);
#949=B_SPLINE_CURVE_WITH_KNOTS('',2,(#71027,#71028,#71029),
 .UNSPECIFIED.,.F.,.F.,(3,3),(0.,1.),.UNSPECIFIED.);
#950=B_SPLINE_CURVE_WITH_KNOTS('',2,(#71037,#71038,#71039),
 .UNSPECIFIED.,.F.,.F.,(3,3),(0.,1.),.UNSPECIFIED.);
#951=B_SPLINE_CURVE_WITH_KNOTS('',2,(#71042,#71043,#71044),
 .UNSPECIFIED.,.F.,.F.,(3,3),(0.,1.),.UNSPECIFIED.);
#952=B_SPLINE_CURVE_WITH_KNOTS('',2,(#71057,#71058,#71059),
 .UNSPECIFIED.,.F.,.F.,(3,3),(0.,1.),.UNSPECIFIED.);
#953=B_SPLINE_CURVE_WITH_KNOTS('',2,(#71060,#71061,#71062),
 .UNSPECIFIED.,.F.,.F.,(3,3),(0.,1.),.UNSPECIFIED.);
#954=B_SPLINE_CURVE_WITH_KNOTS('',2,(#71073,#71074,#71075),
 .UNSPECIFIED.,.F.,.F.,(3,3),(0.,1.),.UNSPECIFIED.);
#955=B_SPLINE_CURVE_WITH_KNOTS('',2,(#71079,#71080,#71081),
 .UNSPECIFIED.,.F.,.F.,(3,3),(0.,1.),.UNSPECIFIED.);
#956=B_SPLINE_CURVE_WITH_KNOTS('',2,(#71090,#71091,#71092),
 .UNSPECIFIED.,.F.,.F.,(3,3),(0.,1.),.UNSPECIFIED.);
#957=B_SPLINE_CURVE_WITH_KNOTS('',2,(#71095,#71096,#71097),
 .UNSPECIFIED.,.F.,.F.,(3,3),(0.,1.),.UNSPECIFIED.);
#958=B_SPLINE_CURVE_WITH_KNOTS('',2,(#71105,#71106,#71107),
 .UNSPECIFIED.,.F.,.F.,(3,3),(0.,1.),.UNSPECIFIED.);
#959=B_SPLINE_CURVE_WITH_KNOTS('',2,(#71110,#71111,#71112),
 .UNSPECIFIED.,.F.,.F.,(3,3),(0.,1.),.UNSPECIFIED.);
#960=B_SPLINE_CURVE_WITH_KNOTS('',2,(#71120,#71121,#71122),
 .UNSPECIFIED.,.F.,.F.,(3,3),(0.,1.),.UNSPECIFIED.);
#961=B_SPLINE_CURVE_WITH_KNOTS('',2,(#71125,#71126,#71127),
 .UNSPECIFIED.,.F.,.F.,(3,3),(0.,1.),.UNSPECIFIED.);
#962=B_SPLINE_CURVE_WITH_KNOTS('',2,(#71135,#71136,#71137),
 .UNSPECIFIED.,.F.,.F.,(3,3),(0.,1.),.UNSPECIFIED.);
#963=B_SPLINE_CURVE_WITH_KNOTS('',2,(#71140,#71141,#71142),
 .UNSPECIFIED.,.F.,.F.,(3,3),(0.,1.),.UNSPECIFIED.);
#964=B_SPLINE_CURVE_WITH_KNOTS('',2,(#71150,#71151,#71152),
 .UNSPECIFIED.,.F.,.F.,(3,3),(0.,1.),.UNSPECIFIED.);
#965=B_SPLINE_CURVE_WITH_KNOTS('',2,(#71155,#71156,#71157),
 .UNSPECIFIED.,.F.,.F.,(3,3),(0.,1.),.UNSPECIFIED.);
#966=B_SPLINE_CURVE_WITH_KNOTS('',2,(#71165,#71166,#71167),
 .UNSPECIFIED.,.F.,.F.,(3,3),(0.,1.),.UNSPECIFIED.);
#967=B_SPLINE_CURVE_WITH_KNOTS('',2,(#71170,#71171,#71172),
 .UNSPECIFIED.,.F.,.F.,(3,3),(0.,1.),.UNSPECIFIED.);
#968=B_SPLINE_CURVE_WITH_KNOTS('',2,(#71179,#71180,#71181),
 .UNSPECIFIED.,.F.,.F.,(3,3),(0.,1.),.UNSPECIFIED.);
#969=B_SPLINE_CURVE_WITH_KNOTS('',2,(#71182,#71183,#71184),
 .UNSPECIFIED.,.F.,.F.,(3,3),(0.,1.),.UNSPECIFIED.);
#970=B_SPLINE_CURVE_WITH_KNOTS('',2,(#71193,#71194,#71195),
 .UNSPECIFIED.,.F.,.F.,(3,3),(0.,1.),.UNSPECIFIED.);
#971=B_SPLINE_CURVE_WITH_KNOTS('',2,(#71199,#71200,#71201),
 .UNSPECIFIED.,.F.,.F.,(3,3),(0.,1.),.UNSPECIFIED.);
#972=B_SPLINE_CURVE_WITH_KNOTS('',2,(#71210,#71211,#71212),
 .UNSPECIFIED.,.F.,.F.,(3,3),(0.,1.),.UNSPECIFIED.);
#973=B_SPLINE_CURVE_WITH_KNOTS('',2,(#71215,#71216,#71217),
 .UNSPECIFIED.,.F.,.F.,(3,3),(0.,1.),.UNSPECIFIED.);
#974=B_SPLINE_CURVE_WITH_KNOTS('',2,(#71225,#71226,#71227),
 .UNSPECIFIED.,.F.,.F.,(3,3),(0.,1.),.UNSPECIFIED.);
#975=B_SPLINE_CURVE_WITH_KNOTS('',2,(#71230,#71231,#71232),
 .UNSPECIFIED.,.F.,.F.,(3,3),(0.,1.),.UNSPECIFIED.);
#976=B_SPLINE_CURVE_WITH_KNOTS('',2,(#71240,#71241,#71242),
 .UNSPECIFIED.,.F.,.F.,(3,3),(0.,1.),.UNSPECIFIED.);
#977=B_SPLINE_CURVE_WITH_KNOTS('',2,(#71245,#71246,#71247),
 .UNSPECIFIED.,.F.,.F.,(3,3),(0.,1.),.UNSPECIFIED.);
#978=B_SPLINE_CURVE_WITH_KNOTS('',2,(#71255,#71256,#71257),
 .UNSPECIFIED.,.F.,.F.,(3,3),(0.,1.),.UNSPECIFIED.);
#979=B_SPLINE_CURVE_WITH_KNOTS('',2,(#71260,#71261,#71262),
 .UNSPECIFIED.,.F.,.F.,(3,3),(0.,1.),.UNSPECIFIED.);
#980=B_SPLINE_CURVE_WITH_KNOTS('',2,(#71270,#71271,#71272),
 .UNSPECIFIED.,.F.,.F.,(3,3),(0.,1.),.UNSPECIFIED.);
#981=B_SPLINE_CURVE_WITH_KNOTS('',2,(#71275,#71276,#71277),
 .UNSPECIFIED.,.F.,.F.,(3,3),(0.,1.),.UNSPECIFIED.);
#982=B_SPLINE_CURVE_WITH_KNOTS('',2,(#71285,#71286,#71287),
 .UNSPECIFIED.,.F.,.F.,(3,3),(0.,1.),.UNSPECIFIED.);
#983=B_SPLINE_CURVE_WITH_KNOTS('',2,(#71290,#71291,#71292),
 .UNSPECIFIED.,.F.,.F.,(3,3),(0.,1.),.UNSPECIFIED.);
#984=B_SPLINE_CURVE_WITH_KNOTS('',2,(#71300,#71301,#71302),
 .UNSPECIFIED.,.F.,.F.,(3,3),(0.,1.),.UNSPECIFIED.);
#985=B_SPLINE_CURVE_WITH_KNOTS('',2,(#71305,#71306,#71307),
 .UNSPECIFIED.,.F.,.F.,(3,3),(0.,1.),.UNSPECIFIED.);
#986=B_SPLINE_CURVE_WITH_KNOTS('',2,(#71315,#71316,#71317),
 .UNSPECIFIED.,.F.,.F.,(3,3),(0.,1.),.UNSPECIFIED.);
#987=B_SPLINE_CURVE_WITH_KNOTS('',2,(#71320,#71321,#71322),
 .UNSPECIFIED.,.F.,.F.,(3,3),(0.,1.),.UNSPECIFIED.);
#988=B_SPLINE_CURVE_WITH_KNOTS('',2,(#71330,#71331,#71332),
 .UNSPECIFIED.,.F.,.F.,(3,3),(0.,1.),.UNSPECIFIED.);
#989=B_SPLINE_CURVE_WITH_KNOTS('',2,(#71335,#71336,#71337),
 .UNSPECIFIED.,.F.,.F.,(3,3),(0.,1.),.UNSPECIFIED.);
#990=B_SPLINE_CURVE_WITH_KNOTS('',2,(#71345,#71346,#71347),
 .UNSPECIFIED.,.F.,.F.,(3,3),(0.,1.),.UNSPECIFIED.);
#991=B_SPLINE_CURVE_WITH_KNOTS('',2,(#71350,#71351,#71352),
 .UNSPECIFIED.,.F.,.F.,(3,3),(0.,1.),.UNSPECIFIED.);
#992=B_SPLINE_CURVE_WITH_KNOTS('',2,(#71359,#71360,#71361),
 .UNSPECIFIED.,.F.,.F.,(3,3),(0.,1.),.UNSPECIFIED.);
#993=B_SPLINE_CURVE_WITH_KNOTS('',2,(#71362,#71363,#71364),
 .UNSPECIFIED.,.F.,.F.,(3,3),(0.,1.),.UNSPECIFIED.);
#994=B_SPLINE_CURVE_WITH_KNOTS('',2,(#71374,#71375,#71376),
 .UNSPECIFIED.,.F.,.F.,(3,3),(0.,1.),.UNSPECIFIED.);
#995=B_SPLINE_CURVE_WITH_KNOTS('',2,(#71380,#71381,#71382),
 .UNSPECIFIED.,.F.,.F.,(3,3),(0.,1.),.UNSPECIFIED.);
#996=B_SPLINE_CURVE_WITH_KNOTS('',2,(#71391,#71392,#71393),
 .UNSPECIFIED.,.F.,.F.,(3,3),(0.,1.),.UNSPECIFIED.);
#997=B_SPLINE_CURVE_WITH_KNOTS('',2,(#71396,#71397,#71398),
 .UNSPECIFIED.,.F.,.F.,(3,3),(0.,1.),.UNSPECIFIED.);
#998=B_SPLINE_CURVE_WITH_KNOTS('',2,(#71406,#71407,#71408),
 .UNSPECIFIED.,.F.,.F.,(3,3),(0.,1.),.UNSPECIFIED.);
#999=B_SPLINE_CURVE_WITH_KNOTS('',2,(#71411,#71412,#71413),
 .UNSPECIFIED.,.F.,.F.,(3,3),(0.,1.),.UNSPECIFIED.);
#1000=B_SPLINE_CURVE_WITH_KNOTS('',2,(#71421,#71422,#71423),
 .UNSPECIFIED.,.F.,.F.,(3,3),(0.,1.),.UNSPECIFIED.);
#1001=B_SPLINE_CURVE_WITH_KNOTS('',2,(#71426,#71427,#71428),
 .UNSPECIFIED.,.F.,.F.,(3,3),(0.,1.),.UNSPECIFIED.);
#1002=B_SPLINE_CURVE_WITH_KNOTS('',2,(#71436,#71437,#71438),
 .UNSPECIFIED.,.F.,.F.,(3,3),(0.,1.),.UNSPECIFIED.);
#1003=B_SPLINE_CURVE_WITH_KNOTS('',2,(#71441,#71442,#71443),
 .UNSPECIFIED.,.F.,.F.,(3,3),(0.,1.),.UNSPECIFIED.);
#1004=B_SPLINE_CURVE_WITH_KNOTS('',2,(#71451,#71452,#71453),
 .UNSPECIFIED.,.F.,.F.,(3,3),(0.,1.),.UNSPECIFIED.);
#1005=B_SPLINE_CURVE_WITH_KNOTS('',2,(#71456,#71457,#71458),
 .UNSPECIFIED.,.F.,.F.,(3,3),(0.,1.),.UNSPECIFIED.);
#1006=B_SPLINE_CURVE_WITH_KNOTS('',2,(#71466,#71467,#71468),
 .UNSPECIFIED.,.F.,.F.,(3,3),(0.,1.),.UNSPECIFIED.);
#1007=B_SPLINE_CURVE_WITH_KNOTS('',2,(#71471,#71472,#71473),
 .UNSPECIFIED.,.F.,.F.,(3,3),(0.,1.),.UNSPECIFIED.);
#1008=B_SPLINE_CURVE_WITH_KNOTS('',2,(#71481,#71482,#71483),
 .UNSPECIFIED.,.F.,.F.,(3,3),(0.,1.),.UNSPECIFIED.);
#1009=B_SPLINE_CURVE_WITH_KNOTS('',2,(#71486,#71487,#71488),
 .UNSPECIFIED.,.F.,.F.,(3,3),(0.,1.),.UNSPECIFIED.);
#1010=B_SPLINE_CURVE_WITH_KNOTS('',2,(#71496,#71497,#71498),
 .UNSPECIFIED.,.F.,.F.,(3,3),(0.,1.),.UNSPECIFIED.);
#1011=B_SPLINE_CURVE_WITH_KNOTS('',2,(#71501,#71502,#71503),
 .UNSPECIFIED.,.F.,.F.,(3,3),(0.,1.),.UNSPECIFIED.);
#1012=B_SPLINE_CURVE_WITH_KNOTS('',2,(#71517,#71518,#71519),
 .UNSPECIFIED.,.F.,.F.,(3,3),(0.,1.),.UNSPECIFIED.);
#1013=B_SPLINE_CURVE_WITH_KNOTS('',2,(#71522,#71523,#71524),
 .UNSPECIFIED.,.F.,.F.,(3,3),(0.,1.),.UNSPECIFIED.);
#1014=B_SPLINE_CURVE_WITH_KNOTS('',2,(#71532,#71533,#71534),
 .UNSPECIFIED.,.F.,.F.,(3,3),(0.,1.),.UNSPECIFIED.);
#1015=B_SPLINE_CURVE_WITH_KNOTS('',2,(#71537,#71538,#71539),
 .UNSPECIFIED.,.F.,.F.,(3,3),(0.,1.),.UNSPECIFIED.);
#1016=B_SPLINE_CURVE_WITH_KNOTS('',2,(#71547,#71548,#71549),
 .UNSPECIFIED.,.F.,.F.,(3,3),(0.,1.),.UNSPECIFIED.);
#1017=B_SPLINE_CURVE_WITH_KNOTS('',2,(#71552,#71553,#71554),
 .UNSPECIFIED.,.F.,.F.,(3,3),(0.,1.),.UNSPECIFIED.);
#1018=B_SPLINE_CURVE_WITH_KNOTS('',2,(#71562,#71563,#71564),
 .UNSPECIFIED.,.F.,.F.,(3,3),(0.,1.),.UNSPECIFIED.);
#1019=B_SPLINE_CURVE_WITH_KNOTS('',2,(#71567,#71568,#71569),
 .UNSPECIFIED.,.F.,.F.,(3,3),(0.,1.),.UNSPECIFIED.);
#1020=B_SPLINE_CURVE_WITH_KNOTS('',2,(#71577,#71578,#71579),
 .UNSPECIFIED.,.F.,.F.,(3,3),(0.,1.),.UNSPECIFIED.);
#1021=B_SPLINE_CURVE_WITH_KNOTS('',2,(#71582,#71583,#71584),
 .UNSPECIFIED.,.F.,.F.,(3,3),(0.,1.),.UNSPECIFIED.);
#1022=B_SPLINE_CURVE_WITH_KNOTS('',2,(#71592,#71593,#71594),
 .UNSPECIFIED.,.F.,.F.,(3,3),(0.,1.),.UNSPECIFIED.);
#1023=B_SPLINE_CURVE_WITH_KNOTS('',2,(#71597,#71598,#71599),
 .UNSPECIFIED.,.F.,.F.,(3,3),(0.,1.),.UNSPECIFIED.);
#1024=B_SPLINE_CURVE_WITH_KNOTS('',2,(#71607,#71608,#71609),
 .UNSPECIFIED.,.F.,.F.,(3,3),(0.,1.),.UNSPECIFIED.);
#1025=B_SPLINE_CURVE_WITH_KNOTS('',2,(#71612,#71613,#71614),
 .UNSPECIFIED.,.F.,.F.,(3,3),(0.,1.),.UNSPECIFIED.);
#1026=B_SPLINE_CURVE_WITH_KNOTS('',2,(#71622,#71623,#71624),
 .UNSPECIFIED.,.F.,.F.,(3,3),(0.,1.),.UNSPECIFIED.);
#1027=B_SPLINE_CURVE_WITH_KNOTS('',2,(#71627,#71628,#71629),
 .UNSPECIFIED.,.F.,.F.,(3,3),(0.,1.),.UNSPECIFIED.);
#1028=B_SPLINE_CURVE_WITH_KNOTS('',2,(#71637,#71638,#71639),
 .UNSPECIFIED.,.F.,.F.,(3,3),(0.,1.),.UNSPECIFIED.);
#1029=B_SPLINE_CURVE_WITH_KNOTS('',2,(#71642,#71643,#71644),
 .UNSPECIFIED.,.F.,.F.,(3,3),(0.,1.),.UNSPECIFIED.);
#1030=B_SPLINE_CURVE_WITH_KNOTS('',2,(#71670,#71671,#71672),
 .UNSPECIFIED.,.F.,.F.,(3,3),(0.,1.),.UNSPECIFIED.);
#1031=B_SPLINE_CURVE_WITH_KNOTS('',2,(#71676,#71677,#71678),
 .UNSPECIFIED.,.F.,.F.,(3,3),(0.,1.),.UNSPECIFIED.);
#1032=B_SPLINE_CURVE_WITH_KNOTS('',2,(#71687,#71688,#71689),
 .UNSPECIFIED.,.F.,.F.,(3,3),(0.,1.),.UNSPECIFIED.);
#1033=B_SPLINE_CURVE_WITH_KNOTS('',2,(#71692,#71693,#71694),
 .UNSPECIFIED.,.F.,.F.,(3,3),(0.,1.),.UNSPECIFIED.);
#1034=B_SPLINE_CURVE_WITH_KNOTS('',2,(#71702,#71703,#71704),
 .UNSPECIFIED.,.F.,.F.,(3,3),(0.,1.),.UNSPECIFIED.);
#1035=B_SPLINE_CURVE_WITH_KNOTS('',2,(#71707,#71708,#71709),
 .UNSPECIFIED.,.F.,.F.,(3,3),(0.,1.),.UNSPECIFIED.);
#1036=B_SPLINE_CURVE_WITH_KNOTS('',2,(#71717,#71718,#71719),
 .UNSPECIFIED.,.F.,.F.,(3,3),(0.,1.),.UNSPECIFIED.);
#1037=B_SPLINE_CURVE_WITH_KNOTS('',2,(#71722,#71723,#71724),
 .UNSPECIFIED.,.F.,.F.,(3,3),(0.,1.),.UNSPECIFIED.);
#1038=B_SPLINE_CURVE_WITH_KNOTS('',2,(#71732,#71733,#71734),
 .UNSPECIFIED.,.F.,.F.,(3,3),(0.,1.),.UNSPECIFIED.);
#1039=B_SPLINE_CURVE_WITH_KNOTS('',2,(#71737,#71738,#71739),
 .UNSPECIFIED.,.F.,.F.,(3,3),(0.,1.),.UNSPECIFIED.);
#1040=B_SPLINE_CURVE_WITH_KNOTS('',2,(#71747,#71748,#71749),
 .UNSPECIFIED.,.F.,.F.,(3,3),(0.,1.),.UNSPECIFIED.);
#1041=B_SPLINE_CURVE_WITH_KNOTS('',2,(#71752,#71753,#71754),
 .UNSPECIFIED.,.F.,.F.,(3,3),(0.,1.),.UNSPECIFIED.);
#1042=B_SPLINE_CURVE_WITH_KNOTS('',2,(#71762,#71763,#71764),
 .UNSPECIFIED.,.F.,.F.,(3,3),(0.,1.),.UNSPECIFIED.);
#1043=B_SPLINE_CURVE_WITH_KNOTS('',2,(#71767,#71768,#71769),
 .UNSPECIFIED.,.F.,.F.,(3,3),(0.,1.),.UNSPECIFIED.);
#1044=B_SPLINE_CURVE_WITH_KNOTS('',2,(#71776,#71777,#71778),
 .UNSPECIFIED.,.F.,.F.,(3,3),(0.,1.),.UNSPECIFIED.);
#1045=B_SPLINE_CURVE_WITH_KNOTS('',2,(#71779,#71780,#71781),
 .UNSPECIFIED.,.F.,.F.,(3,3),(0.,1.),.UNSPECIFIED.);
#1046=B_SPLINE_CURVE_WITH_KNOTS('',2,(#71790,#71791,#71792),
 .UNSPECIFIED.,.F.,.F.,(3,3),(0.,1.),.UNSPECIFIED.);
#1047=B_SPLINE_CURVE_WITH_KNOTS('',2,(#71796,#71797,#71798),
 .UNSPECIFIED.,.F.,.F.,(3,3),(0.,1.),.UNSPECIFIED.);
#1048=B_SPLINE_CURVE_WITH_KNOTS('',2,(#71807,#71808,#71809),
 .UNSPECIFIED.,.F.,.F.,(3,3),(0.,1.),.UNSPECIFIED.);
#1049=B_SPLINE_CURVE_WITH_KNOTS('',2,(#71812,#71813,#71814),
 .UNSPECIFIED.,.F.,.F.,(3,3),(0.,1.),.UNSPECIFIED.);
#1050=B_SPLINE_CURVE_WITH_KNOTS('',2,(#71822,#71823,#71824),
 .UNSPECIFIED.,.F.,.F.,(3,3),(0.,1.),.UNSPECIFIED.);
#1051=B_SPLINE_CURVE_WITH_KNOTS('',2,(#71827,#71828,#71829),
 .UNSPECIFIED.,.F.,.F.,(3,3),(0.,1.),.UNSPECIFIED.);
#1052=B_SPLINE_CURVE_WITH_KNOTS('',2,(#71837,#71838,#71839),
 .UNSPECIFIED.,.F.,.F.,(3,3),(0.,1.),.UNSPECIFIED.);
#1053=B_SPLINE_CURVE_WITH_KNOTS('',2,(#71842,#71843,#71844),
 .UNSPECIFIED.,.F.,.F.,(3,3),(0.,1.),.UNSPECIFIED.);
#1054=B_SPLINE_CURVE_WITH_KNOTS('',2,(#71852,#71853,#71854),
 .UNSPECIFIED.,.F.,.F.,(3,3),(0.,1.),.UNSPECIFIED.);
#1055=B_SPLINE_CURVE_WITH_KNOTS('',2,(#71857,#71858,#71859),
 .UNSPECIFIED.,.F.,.F.,(3,3),(0.,1.),.UNSPECIFIED.);
#1056=B_SPLINE_CURVE_WITH_KNOTS('',2,(#71867,#71868,#71869),
 .UNSPECIFIED.,.F.,.F.,(3,3),(0.,1.),.UNSPECIFIED.);
#1057=B_SPLINE_CURVE_WITH_KNOTS('',2,(#71872,#71873,#71874),
 .UNSPECIFIED.,.F.,.F.,(3,3),(0.,1.),.UNSPECIFIED.);
#1058=B_SPLINE_CURVE_WITH_KNOTS('',2,(#71882,#71883,#71884),
 .UNSPECIFIED.,.F.,.F.,(3,3),(0.,1.),.UNSPECIFIED.);
#1059=B_SPLINE_CURVE_WITH_KNOTS('',2,(#71887,#71888,#71889),
 .UNSPECIFIED.,.F.,.F.,(3,3),(0.,1.),.UNSPECIFIED.);
#1060=B_SPLINE_CURVE_WITH_KNOTS('',2,(#71897,#71898,#71899),
 .UNSPECIFIED.,.F.,.F.,(3,3),(0.,1.),.UNSPECIFIED.);
#1061=B_SPLINE_CURVE_WITH_KNOTS('',2,(#71902,#71903,#71904),
 .UNSPECIFIED.,.F.,.F.,(3,3),(0.,1.),.UNSPECIFIED.);
#1062=B_SPLINE_CURVE_WITH_KNOTS('',2,(#71912,#71913,#71914),
 .UNSPECIFIED.,.F.,.F.,(3,3),(0.,1.),.UNSPECIFIED.);
#1063=B_SPLINE_CURVE_WITH_KNOTS('',2,(#71917,#71918,#71919),
 .UNSPECIFIED.,.F.,.F.,(3,3),(0.,1.),.UNSPECIFIED.);
#1064=B_SPLINE_CURVE_WITH_KNOTS('',2,(#71927,#71928,#71929),
 .UNSPECIFIED.,.F.,.F.,(3,3),(0.,1.),.UNSPECIFIED.);
#1065=B_SPLINE_CURVE_WITH_KNOTS('',2,(#71932,#71933,#71934),
 .UNSPECIFIED.,.F.,.F.,(3,3),(0.,1.),.UNSPECIFIED.);
#1066=B_SPLINE_CURVE_WITH_KNOTS('',2,(#71942,#71943,#71944),
 .UNSPECIFIED.,.F.,.F.,(3,3),(0.,1.),.UNSPECIFIED.);
#1067=B_SPLINE_CURVE_WITH_KNOTS('',2,(#71947,#71948,#71949),
 .UNSPECIFIED.,.F.,.F.,(3,3),(0.,1.),.UNSPECIFIED.);
#1068=B_SPLINE_CURVE_WITH_KNOTS('',2,(#71956,#71957,#71958),
 .UNSPECIFIED.,.F.,.F.,(3,3),(0.,1.),.UNSPECIFIED.);
#1069=B_SPLINE_CURVE_WITH_KNOTS('',2,(#71959,#71960,#71961),
 .UNSPECIFIED.,.F.,.F.,(3,3),(0.,1.),.UNSPECIFIED.);
#1070=B_SPLINE_CURVE_WITH_KNOTS('',2,(#71979,#71980,#71981),
 .UNSPECIFIED.,.F.,.F.,(3,3),(0.,1.),.UNSPECIFIED.);
#1071=B_SPLINE_CURVE_WITH_KNOTS('',2,(#71984,#71985,#71986),
 .UNSPECIFIED.,.F.,.F.,(3,3),(0.,1.),.UNSPECIFIED.);
#1072=B_SPLINE_CURVE_WITH_KNOTS('',2,(#71994,#71995,#71996),
 .UNSPECIFIED.,.F.,.F.,(3,3),(0.,1.),.UNSPECIFIED.);
#1073=B_SPLINE_CURVE_WITH_KNOTS('',2,(#71999,#72000,#72001),
 .UNSPECIFIED.,.F.,.F.,(3,3),(0.,1.),.UNSPECIFIED.);
#1074=B_SPLINE_CURVE_WITH_KNOTS('',2,(#72015,#72016,#72017),
 .UNSPECIFIED.,.F.,.F.,(3,3),(0.,1.),.UNSPECIFIED.);
#1075=B_SPLINE_CURVE_WITH_KNOTS('',2,(#72020,#72021,#72022),
 .UNSPECIFIED.,.F.,.F.,(3,3),(0.,1.),.UNSPECIFIED.);
#1076=B_SPLINE_CURVE_WITH_KNOTS('',2,(#72030,#72031,#72032),
 .UNSPECIFIED.,.F.,.F.,(3,3),(0.,1.),.UNSPECIFIED.);
#1077=B_SPLINE_CURVE_WITH_KNOTS('',2,(#72035,#72036,#72037),
 .UNSPECIFIED.,.F.,.F.,(3,3),(0.,1.),.UNSPECIFIED.);
#1078=B_SPLINE_CURVE_WITH_KNOTS('',2,(#72063,#72064,#72065),
 .UNSPECIFIED.,.F.,.F.,(3,3),(0.,1.),.UNSPECIFIED.);
#1079=B_SPLINE_CURVE_WITH_KNOTS('',2,(#72069,#72070,#72071),
 .UNSPECIFIED.,.F.,.F.,(3,3),(0.,1.),.UNSPECIFIED.);
#1080=B_SPLINE_CURVE_WITH_KNOTS('',2,(#72080,#72081,#72082),
 .UNSPECIFIED.,.F.,.F.,(3,3),(0.,1.),.UNSPECIFIED.);
#1081=B_SPLINE_CURVE_WITH_KNOTS('',2,(#72085,#72086,#72087),
 .UNSPECIFIED.,.F.,.F.,(3,3),(0.,1.),.UNSPECIFIED.);
#1082=B_SPLINE_CURVE_WITH_KNOTS('',2,(#72095,#72096,#72097),
 .UNSPECIFIED.,.F.,.F.,(3,3),(0.,1.),.UNSPECIFIED.);
#1083=B_SPLINE_CURVE_WITH_KNOTS('',2,(#72100,#72101,#72102),
 .UNSPECIFIED.,.F.,.F.,(3,3),(0.,1.),.UNSPECIFIED.);
#1084=B_SPLINE_CURVE_WITH_KNOTS('',2,(#72110,#72111,#72112),
 .UNSPECIFIED.,.F.,.F.,(3,3),(0.,1.),.UNSPECIFIED.);
#1085=B_SPLINE_CURVE_WITH_KNOTS('',2,(#72115,#72116,#72117),
 .UNSPECIFIED.,.F.,.F.,(3,3),(0.,1.),.UNSPECIFIED.);
#1086=B_SPLINE_CURVE_WITH_KNOTS('',2,(#72125,#72126,#72127),
 .UNSPECIFIED.,.F.,.F.,(3,3),(0.,1.),.UNSPECIFIED.);
#1087=B_SPLINE_CURVE_WITH_KNOTS('',2,(#72130,#72131,#72132),
 .UNSPECIFIED.,.F.,.F.,(3,3),(0.,1.),.UNSPECIFIED.);
#1088=B_SPLINE_CURVE_WITH_KNOTS('',2,(#72140,#72141,#72142),
 .UNSPECIFIED.,.F.,.F.,(3,3),(0.,1.),.UNSPECIFIED.);
#1089=B_SPLINE_CURVE_WITH_KNOTS('',2,(#72145,#72146,#72147),
 .UNSPECIFIED.,.F.,.F.,(3,3),(0.,1.),.UNSPECIFIED.);
#1090=B_SPLINE_CURVE_WITH_KNOTS('',2,(#72155,#72156,#72157),
 .UNSPECIFIED.,.F.,.F.,(3,3),(0.,1.),.UNSPECIFIED.);
#1091=B_SPLINE_CURVE_WITH_KNOTS('',2,(#72160,#72161,#72162),
 .UNSPECIFIED.,.F.,.F.,(3,3),(0.,1.),.UNSPECIFIED.);
#1092=B_SPLINE_CURVE_WITH_KNOTS('',2,(#72169,#72170,#72171),
 .UNSPECIFIED.,.F.,.F.,(3,3),(0.,1.),.UNSPECIFIED.);
#1093=B_SPLINE_CURVE_WITH_KNOTS('',2,(#72172,#72173,#72174),
 .UNSPECIFIED.,.F.,.F.,(3,3),(0.,1.),.UNSPECIFIED.);
#1094=B_SPLINE_CURVE_WITH_KNOTS('',2,(#72183,#72184,#72185),
 .UNSPECIFIED.,.F.,.F.,(3,3),(0.,1.),.UNSPECIFIED.);
#1095=B_SPLINE_CURVE_WITH_KNOTS('',2,(#72189,#72190,#72191),
 .UNSPECIFIED.,.F.,.F.,(3,3),(0.,1.),.UNSPECIFIED.);
#1096=B_SPLINE_CURVE_WITH_KNOTS('',2,(#72200,#72201,#72202),
 .UNSPECIFIED.,.F.,.F.,(3,3),(0.,1.),.UNSPECIFIED.);
#1097=B_SPLINE_CURVE_WITH_KNOTS('',2,(#72205,#72206,#72207),
 .UNSPECIFIED.,.F.,.F.,(3,3),(0.,1.),.UNSPECIFIED.);
#1098=B_SPLINE_CURVE_WITH_KNOTS('',2,(#72215,#72216,#72217),
 .UNSPECIFIED.,.F.,.F.,(3,3),(0.,1.),.UNSPECIFIED.);
#1099=B_SPLINE_CURVE_WITH_KNOTS('',2,(#72220,#72221,#72222),
 .UNSPECIFIED.,.F.,.F.,(3,3),(0.,1.),.UNSPECIFIED.);
#1100=B_SPLINE_CURVE_WITH_KNOTS('',2,(#72230,#72231,#72232),
 .UNSPECIFIED.,.F.,.F.,(3,3),(0.,1.),.UNSPECIFIED.);
#1101=B_SPLINE_CURVE_WITH_KNOTS('',2,(#72235,#72236,#72237),
 .UNSPECIFIED.,.F.,.F.,(3,3),(0.,1.),.UNSPECIFIED.);
#1102=B_SPLINE_CURVE_WITH_KNOTS('',2,(#72245,#72246,#72247),
 .UNSPECIFIED.,.F.,.F.,(3,3),(0.,1.),.UNSPECIFIED.);
#1103=B_SPLINE_CURVE_WITH_KNOTS('',2,(#72250,#72251,#72252),
 .UNSPECIFIED.,.F.,.F.,(3,3),(0.,1.),.UNSPECIFIED.);
#1104=B_SPLINE_CURVE_WITH_KNOTS('',2,(#72260,#72261,#72262),
 .UNSPECIFIED.,.F.,.F.,(3,3),(0.,1.),.UNSPECIFIED.);
#1105=B_SPLINE_CURVE_WITH_KNOTS('',2,(#72265,#72266,#72267),
 .UNSPECIFIED.,.F.,.F.,(3,3),(0.,1.),.UNSPECIFIED.);
#1106=B_SPLINE_CURVE_WITH_KNOTS('',2,(#72275,#72276,#72277),
 .UNSPECIFIED.,.F.,.F.,(3,3),(0.,1.),.UNSPECIFIED.);
#1107=B_SPLINE_CURVE_WITH_KNOTS('',2,(#72280,#72281,#72282),
 .UNSPECIFIED.,.F.,.F.,(3,3),(0.,1.),.UNSPECIFIED.);
#1108=B_SPLINE_CURVE_WITH_KNOTS('',2,(#72290,#72291,#72292),
 .UNSPECIFIED.,.F.,.F.,(3,3),(0.,1.),.UNSPECIFIED.);
#1109=B_SPLINE_CURVE_WITH_KNOTS('',2,(#72295,#72296,#72297),
 .UNSPECIFIED.,.F.,.F.,(3,3),(0.,1.),.UNSPECIFIED.);
#1110=B_SPLINE_CURVE_WITH_KNOTS('',2,(#72305,#72306,#72307),
 .UNSPECIFIED.,.F.,.F.,(3,3),(0.,1.),.UNSPECIFIED.);
#1111=B_SPLINE_CURVE_WITH_KNOTS('',2,(#72310,#72311,#72312),
 .UNSPECIFIED.,.F.,.F.,(3,3),(0.,1.),.UNSPECIFIED.);
#1112=B_SPLINE_CURVE_WITH_KNOTS('',2,(#72320,#72321,#72322),
 .UNSPECIFIED.,.F.,.F.,(3,3),(0.,1.),.UNSPECIFIED.);
#1113=B_SPLINE_CURVE_WITH_KNOTS('',2,(#72325,#72326,#72327),
 .UNSPECIFIED.,.F.,.F.,(3,3),(0.,1.),.UNSPECIFIED.);
#1114=B_SPLINE_CURVE_WITH_KNOTS('',2,(#72335,#72336,#72337),
 .UNSPECIFIED.,.F.,.F.,(3,3),(0.,1.),.UNSPECIFIED.);
#1115=B_SPLINE_CURVE_WITH_KNOTS('',2,(#72340,#72341,#72342),
 .UNSPECIFIED.,.F.,.F.,(3,3),(0.,1.),.UNSPECIFIED.);
#1116=B_SPLINE_CURVE_WITH_KNOTS('',2,(#72349,#72350,#72351),
 .UNSPECIFIED.,.F.,.F.,(3,3),(0.,1.),.UNSPECIFIED.);
#1117=B_SPLINE_CURVE_WITH_KNOTS('',2,(#72352,#72353,#72354),
 .UNSPECIFIED.,.F.,.F.,(3,3),(0.,1.),.UNSPECIFIED.);
#1118=B_SPLINE_CURVE_WITH_KNOTS('',2,(#72365,#72366,#72367),
 .UNSPECIFIED.,.F.,.F.,(3,3),(0.,1.),.UNSPECIFIED.);
#1119=B_SPLINE_CURVE_WITH_KNOTS('',2,(#72371,#72372,#72373),
 .UNSPECIFIED.,.F.,.F.,(3,3),(0.,1.),.UNSPECIFIED.);
#1120=B_SPLINE_CURVE_WITH_KNOTS('',2,(#72382,#72383,#72384),
 .UNSPECIFIED.,.F.,.F.,(3,3),(0.,1.),.UNSPECIFIED.);
#1121=B_SPLINE_CURVE_WITH_KNOTS('',2,(#72387,#72388,#72389),
 .UNSPECIFIED.,.F.,.F.,(3,3),(0.,1.),.UNSPECIFIED.);
#1122=B_SPLINE_CURVE_WITH_KNOTS('',2,(#72397,#72398,#72399),
 .UNSPECIFIED.,.F.,.F.,(3,3),(0.,1.),.UNSPECIFIED.);
#1123=B_SPLINE_CURVE_WITH_KNOTS('',2,(#72402,#72403,#72404),
 .UNSPECIFIED.,.F.,.F.,(3,3),(0.,1.),.UNSPECIFIED.);
#1124=B_SPLINE_CURVE_WITH_KNOTS('',2,(#72412,#72413,#72414),
 .UNSPECIFIED.,.F.,.F.,(3,3),(0.,1.),.UNSPECIFIED.);
#1125=B_SPLINE_CURVE_WITH_KNOTS('',2,(#72417,#72418,#72419),
 .UNSPECIFIED.,.F.,.F.,(3,3),(0.,1.),.UNSPECIFIED.);
#1126=B_SPLINE_CURVE_WITH_KNOTS('',2,(#72427,#72428,#72429),
 .UNSPECIFIED.,.F.,.F.,(3,3),(0.,1.),.UNSPECIFIED.);
#1127=B_SPLINE_CURVE_WITH_KNOTS('',2,(#72432,#72433,#72434),
 .UNSPECIFIED.,.F.,.F.,(3,3),(0.,1.),.UNSPECIFIED.);
#1128=B_SPLINE_CURVE_WITH_KNOTS('',2,(#72442,#72443,#72444),
 .UNSPECIFIED.,.F.,.F.,(3,3),(0.,1.),.UNSPECIFIED.);
#1129=B_SPLINE_CURVE_WITH_KNOTS('',2,(#72447,#72448,#72449),
 .UNSPECIFIED.,.F.,.F.,(3,3),(0.,1.),.UNSPECIFIED.);
#1130=B_SPLINE_CURVE_WITH_KNOTS('',2,(#72457,#72458,#72459),
 .UNSPECIFIED.,.F.,.F.,(3,3),(0.,1.),.UNSPECIFIED.);
#1131=B_SPLINE_CURVE_WITH_KNOTS('',2,(#72462,#72463,#72464),
 .UNSPECIFIED.,.F.,.F.,(3,3),(0.,1.),.UNSPECIFIED.);
#1132=B_SPLINE_CURVE_WITH_KNOTS('',2,(#72471,#72472,#72473),
 .UNSPECIFIED.,.F.,.F.,(3,3),(0.,1.),.UNSPECIFIED.);
#1133=B_SPLINE_CURVE_WITH_KNOTS('',2,(#72474,#72475,#72476),
 .UNSPECIFIED.,.F.,.F.,(3,3),(0.,1.),.UNSPECIFIED.);
#1134=B_SPLINE_CURVE_WITH_KNOTS('',2,(#72485,#72486,#72487),
 .UNSPECIFIED.,.F.,.F.,(3,3),(0.,1.),.UNSPECIFIED.);
#1135=B_SPLINE_CURVE_WITH_KNOTS('',2,(#72491,#72492,#72493),
 .UNSPECIFIED.,.F.,.F.,(3,3),(0.,1.),.UNSPECIFIED.);
#1136=B_SPLINE_CURVE_WITH_KNOTS('',2,(#72502,#72503,#72504),
 .UNSPECIFIED.,.F.,.F.,(3,3),(0.,1.),.UNSPECIFIED.);
#1137=B_SPLINE_CURVE_WITH_KNOTS('',2,(#72507,#72508,#72509),
 .UNSPECIFIED.,.F.,.F.,(3,3),(0.,1.),.UNSPECIFIED.);
#1138=B_SPLINE_CURVE_WITH_KNOTS('',2,(#72517,#72518,#72519),
 .UNSPECIFIED.,.F.,.F.,(3,3),(0.,1.),.UNSPECIFIED.);
#1139=B_SPLINE_CURVE_WITH_KNOTS('',2,(#72522,#72523,#72524),
 .UNSPECIFIED.,.F.,.F.,(3,3),(0.,1.),.UNSPECIFIED.);
#1140=B_SPLINE_CURVE_WITH_KNOTS('',2,(#72532,#72533,#72534),
 .UNSPECIFIED.,.F.,.F.,(3,3),(0.,1.),.UNSPECIFIED.);
#1141=B_SPLINE_CURVE_WITH_KNOTS('',2,(#72537,#72538,#72539),
 .UNSPECIFIED.,.F.,.F.,(3,3),(0.,1.),.UNSPECIFIED.);
#1142=B_SPLINE_CURVE_WITH_KNOTS('',2,(#72547,#72548,#72549),
 .UNSPECIFIED.,.F.,.F.,(3,3),(0.,1.),.UNSPECIFIED.);
#1143=B_SPLINE_CURVE_WITH_KNOTS('',2,(#72552,#72553,#72554),
 .UNSPECIFIED.,.F.,.F.,(3,3),(0.,1.),.UNSPECIFIED.);
#1144=B_SPLINE_CURVE_WITH_KNOTS('',2,(#72562,#72563,#72564),
 .UNSPECIFIED.,.F.,.F.,(3,3),(0.,1.),.UNSPECIFIED.);
#1145=B_SPLINE_CURVE_WITH_KNOTS('',2,(#72567,#72568,#72569),
 .UNSPECIFIED.,.F.,.F.,(3,3),(0.,1.),.UNSPECIFIED.);
#1146=B_SPLINE_CURVE_WITH_KNOTS('',2,(#72577,#72578,#72579),
 .UNSPECIFIED.,.F.,.F.,(3,3),(0.,1.),.UNSPECIFIED.);
#1147=B_SPLINE_CURVE_WITH_KNOTS('',2,(#72582,#72583,#72584),
 .UNSPECIFIED.,.F.,.F.,(3,3),(0.,1.),.UNSPECIFIED.);
#1148=B_SPLINE_CURVE_WITH_KNOTS('',2,(#72592,#72593,#72594),
 .UNSPECIFIED.,.F.,.F.,(3,3),(0.,1.),.UNSPECIFIED.);
#1149=B_SPLINE_CURVE_WITH_KNOTS('',2,(#72597,#72598,#72599),
 .UNSPECIFIED.,.F.,.F.,(3,3),(0.,1.),.UNSPECIFIED.);
#1150=B_SPLINE_CURVE_WITH_KNOTS('',2,(#72607,#72608,#72609),
 .UNSPECIFIED.,.F.,.F.,(3,3),(0.,1.),.UNSPECIFIED.);
#1151=B_SPLINE_CURVE_WITH_KNOTS('',2,(#72612,#72613,#72614),
 .UNSPECIFIED.,.F.,.F.,(3,3),(0.,1.),.UNSPECIFIED.);
#1152=B_SPLINE_CURVE_WITH_KNOTS('',2,(#72622,#72623,#72624),
 .UNSPECIFIED.,.F.,.F.,(3,3),(0.,1.),.UNSPECIFIED.);
#1153=B_SPLINE_CURVE_WITH_KNOTS('',2,(#72627,#72628,#72629),
 .UNSPECIFIED.,.F.,.F.,(3,3),(0.,1.),.UNSPECIFIED.);
#1154=B_SPLINE_CURVE_WITH_KNOTS('',2,(#72637,#72638,#72639),
 .UNSPECIFIED.,.F.,.F.,(3,3),(0.,1.),.UNSPECIFIED.);
#1155=B_SPLINE_CURVE_WITH_KNOTS('',2,(#72642,#72643,#72644),
 .UNSPECIFIED.,.F.,.F.,(3,3),(0.,1.),.UNSPECIFIED.);
#1156=B_SPLINE_CURVE_WITH_KNOTS('',2,(#72651,#72652,#72653),
 .UNSPECIFIED.,.F.,.F.,(3,3),(0.,1.),.UNSPECIFIED.);
#1157=B_SPLINE_CURVE_WITH_KNOTS('',2,(#72654,#72655,#72656),
 .UNSPECIFIED.,.F.,.F.,(3,3),(0.,1.),.UNSPECIFIED.);
#1158=B_SPLINE_CURVE_WITH_KNOTS('',2,(#72674,#72675,#72676),
 .UNSPECIFIED.,.F.,.F.,(3,3),(0.,1.),.UNSPECIFIED.);
#1159=B_SPLINE_CURVE_WITH_KNOTS('',2,(#72679,#72680,#72681),
 .UNSPECIFIED.,.F.,.F.,(3,3),(0.,1.),.UNSPECIFIED.);
#1160=B_SPLINE_CURVE_WITH_KNOTS('',2,(#72689,#72690,#72691),
 .UNSPECIFIED.,.F.,.F.,(3,3),(0.,1.),.UNSPECIFIED.);
#1161=B_SPLINE_CURVE_WITH_KNOTS('',2,(#72694,#72695,#72696),
 .UNSPECIFIED.,.F.,.F.,(3,3),(0.,1.),.UNSPECIFIED.);
#1162=B_SPLINE_CURVE_WITH_KNOTS('',2,(#72710,#72711,#72712),
 .UNSPECIFIED.,.F.,.F.,(3,3),(0.,1.),.UNSPECIFIED.);
#1163=B_SPLINE_CURVE_WITH_KNOTS('',2,(#72715,#72716,#72717),
 .UNSPECIFIED.,.F.,.F.,(3,3),(0.,1.),.UNSPECIFIED.);
#1164=B_SPLINE_CURVE_WITH_KNOTS('',2,(#72725,#72726,#72727),
 .UNSPECIFIED.,.F.,.F.,(3,3),(0.,1.),.UNSPECIFIED.);
#1165=B_SPLINE_CURVE_WITH_KNOTS('',2,(#72730,#72731,#72732),
 .UNSPECIFIED.,.F.,.F.,(3,3),(0.,1.),.UNSPECIFIED.);
#1166=B_SPLINE_CURVE_WITH_KNOTS('',2,(#72758,#72759,#72760),
 .UNSPECIFIED.,.F.,.F.,(3,3),(0.,1.),.UNSPECIFIED.);
#1167=B_SPLINE_CURVE_WITH_KNOTS('',2,(#72764,#72765,#72766),
 .UNSPECIFIED.,.F.,.F.,(3,3),(0.,1.),.UNSPECIFIED.);
#1168=B_SPLINE_CURVE_WITH_KNOTS('',2,(#72775,#72776,#72777),
 .UNSPECIFIED.,.F.,.F.,(3,3),(0.,1.),.UNSPECIFIED.);
#1169=B_SPLINE_CURVE_WITH_KNOTS('',2,(#72780,#72781,#72782),
 .UNSPECIFIED.,.F.,.F.,(3,3),(0.,1.),.UNSPECIFIED.);
#1170=B_SPLINE_CURVE_WITH_KNOTS('',2,(#72790,#72791,#72792),
 .UNSPECIFIED.,.F.,.F.,(3,3),(0.,1.),.UNSPECIFIED.);
#1171=B_SPLINE_CURVE_WITH_KNOTS('',2,(#72795,#72796,#72797),
 .UNSPECIFIED.,.F.,.F.,(3,3),(0.,1.),.UNSPECIFIED.);
#1172=B_SPLINE_CURVE_WITH_KNOTS('',2,(#72805,#72806,#72807),
 .UNSPECIFIED.,.F.,.F.,(3,3),(0.,1.),.UNSPECIFIED.);
#1173=B_SPLINE_CURVE_WITH_KNOTS('',2,(#72810,#72811,#72812),
 .UNSPECIFIED.,.F.,.F.,(3,3),(0.,1.),.UNSPECIFIED.);
#1174=B_SPLINE_CURVE_WITH_KNOTS('',2,(#72820,#72821,#72822),
 .UNSPECIFIED.,.F.,.F.,(3,3),(0.,1.),.UNSPECIFIED.);
#1175=B_SPLINE_CURVE_WITH_KNOTS('',2,(#72825,#72826,#72827),
 .UNSPECIFIED.,.F.,.F.,(3,3),(0.,1.),.UNSPECIFIED.);
#1176=B_SPLINE_CURVE_WITH_KNOTS('',2,(#72835,#72836,#72837),
 .UNSPECIFIED.,.F.,.F.,(3,3),(0.,1.),.UNSPECIFIED.);
#1177=B_SPLINE_CURVE_WITH_KNOTS('',2,(#72840,#72841,#72842),
 .UNSPECIFIED.,.F.,.F.,(3,3),(0.,1.),.UNSPECIFIED.);
#1178=B_SPLINE_CURVE_WITH_KNOTS('',2,(#72850,#72851,#72852),
 .UNSPECIFIED.,.F.,.F.,(3,3),(0.,1.),.UNSPECIFIED.);
#1179=B_SPLINE_CURVE_WITH_KNOTS('',2,(#72855,#72856,#72857),
 .UNSPECIFIED.,.F.,.F.,(3,3),(0.,1.),.UNSPECIFIED.);
#1180=B_SPLINE_CURVE_WITH_KNOTS('',2,(#72864,#72865,#72866),
 .UNSPECIFIED.,.F.,.F.,(3,3),(0.,1.),.UNSPECIFIED.);
#1181=B_SPLINE_CURVE_WITH_KNOTS('',2,(#72867,#72868,#72869),
 .UNSPECIFIED.,.F.,.F.,(3,3),(0.,1.),.UNSPECIFIED.);
#1182=B_SPLINE_CURVE_WITH_KNOTS('',2,(#72878,#72879,#72880),
 .UNSPECIFIED.,.F.,.F.,(3,3),(0.,1.),.UNSPECIFIED.);
#1183=B_SPLINE_CURVE_WITH_KNOTS('',2,(#72884,#72885,#72886),
 .UNSPECIFIED.,.F.,.F.,(3,3),(0.,1.),.UNSPECIFIED.);
#1184=B_SPLINE_CURVE_WITH_KNOTS('',2,(#72895,#72896,#72897),
 .UNSPECIFIED.,.F.,.F.,(3,3),(0.,1.),.UNSPECIFIED.);
#1185=B_SPLINE_CURVE_WITH_KNOTS('',2,(#72900,#72901,#72902),
 .UNSPECIFIED.,.F.,.F.,(3,3),(0.,1.),.UNSPECIFIED.);
#1186=B_SPLINE_CURVE_WITH_KNOTS('',2,(#72910,#72911,#72912),
 .UNSPECIFIED.,.F.,.F.,(3,3),(0.,1.),.UNSPECIFIED.);
#1187=B_SPLINE_CURVE_WITH_KNOTS('',2,(#72915,#72916,#72917),
 .UNSPECIFIED.,.F.,.F.,(3,3),(0.,1.),.UNSPECIFIED.);
#1188=B_SPLINE_CURVE_WITH_KNOTS('',2,(#72925,#72926,#72927),
 .UNSPECIFIED.,.F.,.F.,(3,3),(0.,1.),.UNSPECIFIED.);
#1189=B_SPLINE_CURVE_WITH_KNOTS('',2,(#72930,#72931,#72932),
 .UNSPECIFIED.,.F.,.F.,(3,3),(0.,1.),.UNSPECIFIED.);
#1190=B_SPLINE_CURVE_WITH_KNOTS('',2,(#72940,#72941,#72942),
 .UNSPECIFIED.,.F.,.F.,(3,3),(0.,1.),.UNSPECIFIED.);
#1191=B_SPLINE_CURVE_WITH_KNOTS('',2,(#72945,#72946,#72947),
 .UNSPECIFIED.,.F.,.F.,(3,3),(0.,1.),.UNSPECIFIED.);
#1192=B_SPLINE_CURVE_WITH_KNOTS('',2,(#72955,#72956,#72957),
 .UNSPECIFIED.,.F.,.F.,(3,3),(0.,1.),.UNSPECIFIED.);
#1193=B_SPLINE_CURVE_WITH_KNOTS('',2,(#72960,#72961,#72962),
 .UNSPECIFIED.,.F.,.F.,(3,3),(0.,1.),.UNSPECIFIED.);
#1194=B_SPLINE_CURVE_WITH_KNOTS('',2,(#72970,#72971,#72972),
 .UNSPECIFIED.,.F.,.F.,(3,3),(0.,1.),.UNSPECIFIED.);
#1195=B_SPLINE_CURVE_WITH_KNOTS('',2,(#72975,#72976,#72977),
 .UNSPECIFIED.,.F.,.F.,(3,3),(0.,1.),.UNSPECIFIED.);
#1196=B_SPLINE_CURVE_WITH_KNOTS('',2,(#72985,#72986,#72987),
 .UNSPECIFIED.,.F.,.F.,(3,3),(0.,1.),.UNSPECIFIED.);
#1197=B_SPLINE_CURVE_WITH_KNOTS('',2,(#72990,#72991,#72992),
 .UNSPECIFIED.,.F.,.F.,(3,3),(0.,1.),.UNSPECIFIED.);
#1198=B_SPLINE_CURVE_WITH_KNOTS('',2,(#73000,#73001,#73002),
 .UNSPECIFIED.,.F.,.F.,(3,3),(0.,1.),.UNSPECIFIED.);
#1199=B_SPLINE_CURVE_WITH_KNOTS('',2,(#73005,#73006,#73007),
 .UNSPECIFIED.,.F.,.F.,(3,3),(0.,1.),.UNSPECIFIED.);
#1200=B_SPLINE_CURVE_WITH_KNOTS('',2,(#73015,#73016,#73017),
 .UNSPECIFIED.,.F.,.F.,(3,3),(0.,1.),.UNSPECIFIED.);
#1201=B_SPLINE_CURVE_WITH_KNOTS('',2,(#73020,#73021,#73022),
 .UNSPECIFIED.,.F.,.F.,(3,3),(0.,1.),.UNSPECIFIED.);
#1202=B_SPLINE_CURVE_WITH_KNOTS('',2,(#73030,#73031,#73032),
 .UNSPECIFIED.,.F.,.F.,(3,3),(0.,1.),.UNSPECIFIED.);
#1203=B_SPLINE_CURVE_WITH_KNOTS('',2,(#73035,#73036,#73037),
 .UNSPECIFIED.,.F.,.F.,(3,3),(0.,1.),.UNSPECIFIED.);
#1204=B_SPLINE_CURVE_WITH_KNOTS('',2,(#73044,#73045,#73046),
 .UNSPECIFIED.,.F.,.F.,(3,3),(0.,1.),.UNSPECIFIED.);
#1205=B_SPLINE_CURVE_WITH_KNOTS('',2,(#73047,#73048,#73049),
 .UNSPECIFIED.,.F.,.F.,(3,3),(0.,1.),.UNSPECIFIED.);
#1206=B_SPLINE_CURVE_WITH_KNOTS('',2,(#73059,#73060,#73061),
 .UNSPECIFIED.,.F.,.F.,(3,3),(0.,1.),.UNSPECIFIED.);
#1207=B_SPLINE_CURVE_WITH_KNOTS('',2,(#73065,#73066,#73067),
 .UNSPECIFIED.,.F.,.F.,(3,3),(0.,1.),.UNSPECIFIED.);
#1208=B_SPLINE_CURVE_WITH_KNOTS('',2,(#73076,#73077,#73078),
 .UNSPECIFIED.,.F.,.F.,(3,3),(0.,1.),.UNSPECIFIED.);
#1209=B_SPLINE_CURVE_WITH_KNOTS('',2,(#73081,#73082,#73083),
 .UNSPECIFIED.,.F.,.F.,(3,3),(0.,1.),.UNSPECIFIED.);
#1210=B_SPLINE_CURVE_WITH_KNOTS('',2,(#73091,#73092,#73093),
 .UNSPECIFIED.,.F.,.F.,(3,3),(0.,1.),.UNSPECIFIED.);
#1211=B_SPLINE_CURVE_WITH_KNOTS('',2,(#73096,#73097,#73098),
 .UNSPECIFIED.,.F.,.F.,(3,3),(0.,1.),.UNSPECIFIED.);
#1212=B_SPLINE_CURVE_WITH_KNOTS('',2,(#73106,#73107,#73108),
 .UNSPECIFIED.,.F.,.F.,(3,3),(0.,1.),.UNSPECIFIED.);
#1213=B_SPLINE_CURVE_WITH_KNOTS('',2,(#73111,#73112,#73113),
 .UNSPECIFIED.,.F.,.F.,(3,3),(0.,1.),.UNSPECIFIED.);
#1214=B_SPLINE_CURVE_WITH_KNOTS('',2,(#73121,#73122,#73123),
 .UNSPECIFIED.,.F.,.F.,(3,3),(0.,1.),.UNSPECIFIED.);
#1215=B_SPLINE_CURVE_WITH_KNOTS('',2,(#73126,#73127,#73128),
 .UNSPECIFIED.,.F.,.F.,(3,3),(0.,1.),.UNSPECIFIED.);
#1216=B_SPLINE_CURVE_WITH_KNOTS('',2,(#73136,#73137,#73138),
 .UNSPECIFIED.,.F.,.F.,(3,3),(0.,1.),.UNSPECIFIED.);
#1217=B_SPLINE_CURVE_WITH_KNOTS('',2,(#73141,#73142,#73143),
 .UNSPECIFIED.,.F.,.F.,(3,3),(0.,1.),.UNSPECIFIED.);
#1218=B_SPLINE_CURVE_WITH_KNOTS('',2,(#73151,#73152,#73153),
 .UNSPECIFIED.,.F.,.F.,(3,3),(0.,1.),.UNSPECIFIED.);
#1219=B_SPLINE_CURVE_WITH_KNOTS('',2,(#73156,#73157,#73158),
 .UNSPECIFIED.,.F.,.F.,(3,3),(0.,1.),.UNSPECIFIED.);
#1220=B_SPLINE_CURVE_WITH_KNOTS('',2,(#73166,#73167,#73168),
 .UNSPECIFIED.,.F.,.F.,(3,3),(0.,1.),.UNSPECIFIED.);
#1221=B_SPLINE_CURVE_WITH_KNOTS('',2,(#73171,#73172,#73173),
 .UNSPECIFIED.,.F.,.F.,(3,3),(0.,1.),.UNSPECIFIED.);
#1222=B_SPLINE_CURVE_WITH_KNOTS('',2,(#73181,#73182,#73183),
 .UNSPECIFIED.,.F.,.F.,(3,3),(0.,1.),.UNSPECIFIED.);
#1223=B_SPLINE_CURVE_WITH_KNOTS('',2,(#73186,#73187,#73188),
 .UNSPECIFIED.,.F.,.F.,(3,3),(0.,1.),.UNSPECIFIED.);
#1224=B_SPLINE_CURVE_WITH_KNOTS('',2,(#73202,#73203,#73204),
 .UNSPECIFIED.,.F.,.F.,(3,3),(0.,1.),.UNSPECIFIED.);
#1225=B_SPLINE_CURVE_WITH_KNOTS('',2,(#73207,#73208,#73209),
 .UNSPECIFIED.,.F.,.F.,(3,3),(0.,1.),.UNSPECIFIED.);
#1226=B_SPLINE_CURVE_WITH_KNOTS('',2,(#73217,#73218,#73219),
 .UNSPECIFIED.,.F.,.F.,(3,3),(0.,1.),.UNSPECIFIED.);
#1227=B_SPLINE_CURVE_WITH_KNOTS('',2,(#73222,#73223,#73224),
 .UNSPECIFIED.,.F.,.F.,(3,3),(0.,1.),.UNSPECIFIED.);
#1228=B_SPLINE_CURVE_WITH_KNOTS('',2,(#73232,#73233,#73234),
 .UNSPECIFIED.,.F.,.F.,(3,3),(0.,1.),.UNSPECIFIED.);
#1229=B_SPLINE_CURVE_WITH_KNOTS('',2,(#73237,#73238,#73239),
 .UNSPECIFIED.,.F.,.F.,(3,3),(0.,1.),.UNSPECIFIED.);
#1230=B_SPLINE_CURVE_WITH_KNOTS('',2,(#73247,#73248,#73249),
 .UNSPECIFIED.,.F.,.F.,(3,3),(0.,1.),.UNSPECIFIED.);
#1231=B_SPLINE_CURVE_WITH_KNOTS('',2,(#73252,#73253,#73254),
 .UNSPECIFIED.,.F.,.F.,(3,3),(0.,1.),.UNSPECIFIED.);
#1232=B_SPLINE_CURVE_WITH_KNOTS('',2,(#73262,#73263,#73264),
 .UNSPECIFIED.,.F.,.F.,(3,3),(0.,1.),.UNSPECIFIED.);
#1233=B_SPLINE_CURVE_WITH_KNOTS('',2,(#73267,#73268,#73269),
 .UNSPECIFIED.,.F.,.F.,(3,3),(0.,1.),.UNSPECIFIED.);
#1234=B_SPLINE_CURVE_WITH_KNOTS('',2,(#73277,#73278,#73279),
 .UNSPECIFIED.,.F.,.F.,(3,3),(0.,1.),.UNSPECIFIED.);
#1235=B_SPLINE_CURVE_WITH_KNOTS('',2,(#73282,#73283,#73284),
 .UNSPECIFIED.,.F.,.F.,(3,3),(0.,1.),.UNSPECIFIED.);
#1236=B_SPLINE_CURVE_WITH_KNOTS('',2,(#73292,#73293,#73294),
 .UNSPECIFIED.,.F.,.F.,(3,3),(0.,1.),.UNSPECIFIED.);
#1237=B_SPLINE_CURVE_WITH_KNOTS('',2,(#73297,#73298,#73299),
 .UNSPECIFIED.,.F.,.F.,(3,3),(0.,1.),.UNSPECIFIED.);
#1238=B_SPLINE_CURVE_WITH_KNOTS('',2,(#73307,#73308,#73309),
 .UNSPECIFIED.,.F.,.F.,(3,3),(0.,1.),.UNSPECIFIED.);
#1239=B_SPLINE_CURVE_WITH_KNOTS('',2,(#73312,#73313,#73314),
 .UNSPECIFIED.,.F.,.F.,(3,3),(0.,1.),.UNSPECIFIED.);
#1240=B_SPLINE_CURVE_WITH_KNOTS('',2,(#73322,#73323,#73324),
 .UNSPECIFIED.,.F.,.F.,(3,3),(0.,1.),.UNSPECIFIED.);
#1241=B_SPLINE_CURVE_WITH_KNOTS('',2,(#73327,#73328,#73329),
 .UNSPECIFIED.,.F.,.F.,(3,3),(0.,1.),.UNSPECIFIED.);
#1242=B_SPLINE_CURVE_WITH_KNOTS('',2,(#73355,#73356,#73357),
 .UNSPECIFIED.,.F.,.F.,(3,3),(0.,1.),.UNSPECIFIED.);
#1243=B_SPLINE_CURVE_WITH_KNOTS('',2,(#73361,#73362,#73363),
 .UNSPECIFIED.,.F.,.F.,(3,3),(0.,1.),.UNSPECIFIED.);
#1244=B_SPLINE_CURVE_WITH_KNOTS('',2,(#73372,#73373,#73374),
 .UNSPECIFIED.,.F.,.F.,(3,3),(0.,1.),.UNSPECIFIED.);
#1245=B_SPLINE_CURVE_WITH_KNOTS('',2,(#73377,#73378,#73379),
 .UNSPECIFIED.,.F.,.F.,(3,3),(0.,1.),.UNSPECIFIED.);
#1246=B_SPLINE_CURVE_WITH_KNOTS('',2,(#73387,#73388,#73389),
 .UNSPECIFIED.,.F.,.F.,(3,3),(0.,1.),.UNSPECIFIED.);
#1247=B_SPLINE_CURVE_WITH_KNOTS('',2,(#73392,#73393,#73394),
 .UNSPECIFIED.,.F.,.F.,(3,3),(0.,1.),.UNSPECIFIED.);
#1248=B_SPLINE_CURVE_WITH_KNOTS('',2,(#73402,#73403,#73404),
 .UNSPECIFIED.,.F.,.F.,(3,3),(0.,1.),.UNSPECIFIED.);
#1249=B_SPLINE_CURVE_WITH_KNOTS('',2,(#73407,#73408,#73409),
 .UNSPECIFIED.,.F.,.F.,(3,3),(0.,1.),.UNSPECIFIED.);
#1250=B_SPLINE_CURVE_WITH_KNOTS('',2,(#73417,#73418,#73419),
 .UNSPECIFIED.,.F.,.F.,(3,3),(0.,1.),.UNSPECIFIED.);
#1251=B_SPLINE_CURVE_WITH_KNOTS('',2,(#73422,#73423,#73424),
 .UNSPECIFIED.,.F.,.F.,(3,3),(0.,1.),.UNSPECIFIED.);
#1252=B_SPLINE_CURVE_WITH_KNOTS('',2,(#73432,#73433,#73434),
 .UNSPECIFIED.,.F.,.F.,(3,3),(0.,1.),.UNSPECIFIED.);
#1253=B_SPLINE_CURVE_WITH_KNOTS('',2,(#73437,#73438,#73439),
 .UNSPECIFIED.,.F.,.F.,(3,3),(0.,1.),.UNSPECIFIED.);
#1254=B_SPLINE_CURVE_WITH_KNOTS('',2,(#73447,#73448,#73449),
 .UNSPECIFIED.,.F.,.F.,(3,3),(0.,1.),.UNSPECIFIED.);
#1255=B_SPLINE_CURVE_WITH_KNOTS('',2,(#73452,#73453,#73454),
 .UNSPECIFIED.,.F.,.F.,(3,3),(0.,1.),.UNSPECIFIED.);
#1256=B_SPLINE_CURVE_WITH_KNOTS('',2,(#73461,#73462,#73463),
 .UNSPECIFIED.,.F.,.F.,(3,3),(0.,1.),.UNSPECIFIED.);
#1257=B_SPLINE_CURVE_WITH_KNOTS('',2,(#73464,#73465,#73466),
 .UNSPECIFIED.,.F.,.F.,(3,3),(0.,1.),.UNSPECIFIED.);
#1258=B_SPLINE_CURVE_WITH_KNOTS('',2,(#73475,#73476,#73477),
 .UNSPECIFIED.,.F.,.F.,(3,3),(0.,1.),.UNSPECIFIED.);
#1259=B_SPLINE_CURVE_WITH_KNOTS('',2,(#73481,#73482,#73483),
 .UNSPECIFIED.,.F.,.F.,(3,3),(0.,1.),.UNSPECIFIED.);
#1260=B_SPLINE_CURVE_WITH_KNOTS('',2,(#73492,#73493,#73494),
 .UNSPECIFIED.,.F.,.F.,(3,3),(0.,1.),.UNSPECIFIED.);
#1261=B_SPLINE_CURVE_WITH_KNOTS('',2,(#73497,#73498,#73499),
 .UNSPECIFIED.,.F.,.F.,(3,3),(0.,1.),.UNSPECIFIED.);
#1262=B_SPLINE_CURVE_WITH_KNOTS('',2,(#73507,#73508,#73509),
 .UNSPECIFIED.,.F.,.F.,(3,3),(0.,1.),.UNSPECIFIED.);
#1263=B_SPLINE_CURVE_WITH_KNOTS('',2,(#73512,#73513,#73514),
 .UNSPECIFIED.,.F.,.F.,(3,3),(0.,1.),.UNSPECIFIED.);
#1264=B_SPLINE_CURVE_WITH_KNOTS('',2,(#73522,#73523,#73524),
 .UNSPECIFIED.,.F.,.F.,(3,3),(0.,1.),.UNSPECIFIED.);
#1265=B_SPLINE_CURVE_WITH_KNOTS('',2,(#73527,#73528,#73529),
 .UNSPECIFIED.,.F.,.F.,(3,3),(0.,1.),.UNSPECIFIED.);
#1266=B_SPLINE_CURVE_WITH_KNOTS('',2,(#73537,#73538,#73539),
 .UNSPECIFIED.,.F.,.F.,(3,3),(0.,1.),.UNSPECIFIED.);
#1267=B_SPLINE_CURVE_WITH_KNOTS('',2,(#73542,#73543,#73544),
 .UNSPECIFIED.,.F.,.F.,(3,3),(0.,1.),.UNSPECIFIED.);
#1268=B_SPLINE_CURVE_WITH_KNOTS('',2,(#73552,#73553,#73554),
 .UNSPECIFIED.,.F.,.F.,(3,3),(0.,1.),.UNSPECIFIED.);
#1269=B_SPLINE_CURVE_WITH_KNOTS('',2,(#73557,#73558,#73559),
 .UNSPECIFIED.,.F.,.F.,(3,3),(0.,1.),.UNSPECIFIED.);
#1270=B_SPLINE_CURVE_WITH_KNOTS('',2,(#73567,#73568,#73569),
 .UNSPECIFIED.,.F.,.F.,(3,3),(0.,1.),.UNSPECIFIED.);
#1271=B_SPLINE_CURVE_WITH_KNOTS('',2,(#73572,#73573,#73574),
 .UNSPECIFIED.,.F.,.F.,(3,3),(0.,1.),.UNSPECIFIED.);
#1272=B_SPLINE_CURVE_WITH_KNOTS('',2,(#73582,#73583,#73584),
 .UNSPECIFIED.,.F.,.F.,(3,3),(0.,1.),.UNSPECIFIED.);
#1273=B_SPLINE_CURVE_WITH_KNOTS('',2,(#73587,#73588,#73589),
 .UNSPECIFIED.,.F.,.F.,(3,3),(0.,1.),.UNSPECIFIED.);
#1274=B_SPLINE_CURVE_WITH_KNOTS('',2,(#73597,#73598,#73599),
 .UNSPECIFIED.,.F.,.F.,(3,3),(0.,1.),.UNSPECIFIED.);
#1275=B_SPLINE_CURVE_WITH_KNOTS('',2,(#73602,#73603,#73604),
 .UNSPECIFIED.,.F.,.F.,(3,3),(0.,1.),.UNSPECIFIED.);
#1276=B_SPLINE_CURVE_WITH_KNOTS('',2,(#73612,#73613,#73614),
 .UNSPECIFIED.,.F.,.F.,(3,3),(0.,1.),.UNSPECIFIED.);
#1277=B_SPLINE_CURVE_WITH_KNOTS('',2,(#73617,#73618,#73619),
 .UNSPECIFIED.,.F.,.F.,(3,3),(0.,1.),.UNSPECIFIED.);
#1278=B_SPLINE_CURVE_WITH_KNOTS('',2,(#73627,#73628,#73629),
 .UNSPECIFIED.,.F.,.F.,(3,3),(0.,1.),.UNSPECIFIED.);
#1279=B_SPLINE_CURVE_WITH_KNOTS('',2,(#73632,#73633,#73634),
 .UNSPECIFIED.,.F.,.F.,(3,3),(0.,1.),.UNSPECIFIED.);
#1280=B_SPLINE_CURVE_WITH_KNOTS('',2,(#73641,#73642,#73643),
 .UNSPECIFIED.,.F.,.F.,(3,3),(0.,1.),.UNSPECIFIED.);
#1281=B_SPLINE_CURVE_WITH_KNOTS('',2,(#73644,#73645,#73646),
 .UNSPECIFIED.,.F.,.F.,(3,3),(0.,1.),.UNSPECIFIED.);
#1282=B_SPLINE_CURVE_WITH_KNOTS('',2,(#73656,#73657,#73658),
 .UNSPECIFIED.,.F.,.F.,(3,3),(0.,1.),.UNSPECIFIED.);
#1283=B_SPLINE_CURVE_WITH_KNOTS('',2,(#73662,#73663,#73664),
 .UNSPECIFIED.,.F.,.F.,(3,3),(0.,1.),.UNSPECIFIED.);
#1284=B_SPLINE_CURVE_WITH_KNOTS('',2,(#73673,#73674,#73675),
 .UNSPECIFIED.,.F.,.F.,(3,3),(0.,1.),.UNSPECIFIED.);
#1285=B_SPLINE_CURVE_WITH_KNOTS('',2,(#73678,#73679,#73680),
 .UNSPECIFIED.,.F.,.F.,(3,3),(0.,1.),.UNSPECIFIED.);
#1286=B_SPLINE_CURVE_WITH_KNOTS('',2,(#73688,#73689,#73690),
 .UNSPECIFIED.,.F.,.F.,(3,3),(0.,1.),.UNSPECIFIED.);
#1287=B_SPLINE_CURVE_WITH_KNOTS('',2,(#73693,#73694,#73695),
 .UNSPECIFIED.,.F.,.F.,(3,3),(0.,1.),.UNSPECIFIED.);
#1288=B_SPLINE_CURVE_WITH_KNOTS('',2,(#73703,#73704,#73705),
 .UNSPECIFIED.,.F.,.F.,(3,3),(0.,1.),.UNSPECIFIED.);
#1289=B_SPLINE_CURVE_WITH_KNOTS('',2,(#73708,#73709,#73710),
 .UNSPECIFIED.,.F.,.F.,(3,3),(0.,1.),.UNSPECIFIED.);
#1290=B_SPLINE_CURVE_WITH_KNOTS('',2,(#73718,#73719,#73720),
 .UNSPECIFIED.,.F.,.F.,(3,3),(0.,1.),.UNSPECIFIED.);
#1291=B_SPLINE_CURVE_WITH_KNOTS('',2,(#73723,#73724,#73725),
 .UNSPECIFIED.,.F.,.F.,(3,3),(0.,1.),.UNSPECIFIED.);
#1292=B_SPLINE_CURVE_WITH_KNOTS('',2,(#73733,#73734,#73735),
 .UNSPECIFIED.,.F.,.F.,(3,3),(0.,1.),.UNSPECIFIED.);
#1293=B_SPLINE_CURVE_WITH_KNOTS('',2,(#73738,#73739,#73740),
 .UNSPECIFIED.,.F.,.F.,(3,3),(0.,1.),.UNSPECIFIED.);
#1294=B_SPLINE_CURVE_WITH_KNOTS('',2,(#73748,#73749,#73750),
 .UNSPECIFIED.,.F.,.F.,(3,3),(0.,1.),.UNSPECIFIED.);
#1295=B_SPLINE_CURVE_WITH_KNOTS('',2,(#73753,#73754,#73755),
 .UNSPECIFIED.,.F.,.F.,(3,3),(0.,1.),.UNSPECIFIED.);
#1296=B_SPLINE_CURVE_WITH_KNOTS('',2,(#73763,#73764,#73765),
 .UNSPECIFIED.,.F.,.F.,(3,3),(0.,1.),.UNSPECIFIED.);
#1297=B_SPLINE_CURVE_WITH_KNOTS('',2,(#73768,#73769,#73770),
 .UNSPECIFIED.,.F.,.F.,(3,3),(0.,1.),.UNSPECIFIED.);
#1298=B_SPLINE_CURVE_WITH_KNOTS('',2,(#73778,#73779,#73780),
 .UNSPECIFIED.,.F.,.F.,(3,3),(0.,1.),.UNSPECIFIED.);
#1299=B_SPLINE_CURVE_WITH_KNOTS('',2,(#73783,#73784,#73785),
 .UNSPECIFIED.,.F.,.F.,(3,3),(0.,1.),.UNSPECIFIED.);
#1300=B_SPLINE_CURVE_WITH_KNOTS('',2,(#73793,#73794,#73795),
 .UNSPECIFIED.,.F.,.F.,(3,3),(0.,1.),.UNSPECIFIED.);
#1301=B_SPLINE_CURVE_WITH_KNOTS('',2,(#73798,#73799,#73800),
 .UNSPECIFIED.,.F.,.F.,(3,3),(0.,1.),.UNSPECIFIED.);
#1302=B_SPLINE_CURVE_WITH_KNOTS('',2,(#73808,#73809,#73810),
 .UNSPECIFIED.,.F.,.F.,(3,3),(0.,1.),.UNSPECIFIED.);
#1303=B_SPLINE_CURVE_WITH_KNOTS('',2,(#73813,#73814,#73815),
 .UNSPECIFIED.,.F.,.F.,(3,3),(0.,1.),.UNSPECIFIED.);
#1304=B_SPLINE_CURVE_WITH_KNOTS('',2,(#73823,#73824,#73825),
 .UNSPECIFIED.,.F.,.F.,(3,3),(0.,1.),.UNSPECIFIED.);
#1305=B_SPLINE_CURVE_WITH_KNOTS('',2,(#73828,#73829,#73830),
 .UNSPECIFIED.,.F.,.F.,(3,3),(0.,1.),.UNSPECIFIED.);
#1306=B_SPLINE_CURVE_WITH_KNOTS('',2,(#73844,#73845,#73846),
 .UNSPECIFIED.,.F.,.F.,(3,3),(0.,1.),.UNSPECIFIED.);
#1307=B_SPLINE_CURVE_WITH_KNOTS('',2,(#73849,#73850,#73851),
 .UNSPECIFIED.,.F.,.F.,(3,3),(0.,1.),.UNSPECIFIED.);
#1308=B_SPLINE_CURVE_WITH_KNOTS('',2,(#73859,#73860,#73861),
 .UNSPECIFIED.,.F.,.F.,(3,3),(0.,1.),.UNSPECIFIED.);
#1309=B_SPLINE_CURVE_WITH_KNOTS('',2,(#73864,#73865,#73866),
 .UNSPECIFIED.,.F.,.F.,(3,3),(0.,1.),.UNSPECIFIED.);
#1310=B_SPLINE_CURVE_WITH_KNOTS('',2,(#73874,#73875,#73876),
 .UNSPECIFIED.,.F.,.F.,(3,3),(0.,1.),.UNSPECIFIED.);
#1311=B_SPLINE_CURVE_WITH_KNOTS('',2,(#73879,#73880,#73881),
 .UNSPECIFIED.,.F.,.F.,(3,3),(0.,1.),.UNSPECIFIED.);
#1312=B_SPLINE_CURVE_WITH_KNOTS('',2,(#73889,#73890,#73891),
 .UNSPECIFIED.,.F.,.F.,(3,3),(0.,1.),.UNSPECIFIED.);
#1313=B_SPLINE_CURVE_WITH_KNOTS('',2,(#73894,#73895,#73896),
 .UNSPECIFIED.,.F.,.F.,(3,3),(0.,1.),.UNSPECIFIED.);
#1314=B_SPLINE_CURVE_WITH_KNOTS('',2,(#73904,#73905,#73906),
 .UNSPECIFIED.,.F.,.F.,(3,3),(0.,1.),.UNSPECIFIED.);
#1315=B_SPLINE_CURVE_WITH_KNOTS('',2,(#73909,#73910,#73911),
 .UNSPECIFIED.,.F.,.F.,(3,3),(0.,1.),.UNSPECIFIED.);
#1316=B_SPLINE_CURVE_WITH_KNOTS('',2,(#73919,#73920,#73921),
 .UNSPECIFIED.,.F.,.F.,(3,3),(0.,1.),.UNSPECIFIED.);
#1317=B_SPLINE_CURVE_WITH_KNOTS('',2,(#73924,#73925,#73926),
 .UNSPECIFIED.,.F.,.F.,(3,3),(0.,1.),.UNSPECIFIED.);
#1318=B_SPLINE_CURVE_WITH_KNOTS('',2,(#73934,#73935,#73936),
 .UNSPECIFIED.,.F.,.F.,(3,3),(0.,1.),.UNSPECIFIED.);
#1319=B_SPLINE_CURVE_WITH_KNOTS('',2,(#73939,#73940,#73941),
 .UNSPECIFIED.,.F.,.F.,(3,3),(0.,1.),.UNSPECIFIED.);
#1320=B_SPLINE_CURVE_WITH_KNOTS('',2,(#73955,#73956,#73957),
 .UNSPECIFIED.,.F.,.F.,(3,3),(0.,1.),.UNSPECIFIED.);
#1321=B_SPLINE_CURVE_WITH_KNOTS('',2,(#73960,#73961,#73962),
 .UNSPECIFIED.,.F.,.F.,(3,3),(0.,1.),.UNSPECIFIED.);
#1322=B_SPLINE_CURVE_WITH_KNOTS('',2,(#73970,#73971,#73972),
 .UNSPECIFIED.,.F.,.F.,(3,3),(0.,1.),.UNSPECIFIED.);
#1323=B_SPLINE_CURVE_WITH_KNOTS('',2,(#73975,#73976,#73977),
 .UNSPECIFIED.,.F.,.F.,(3,3),(0.,1.),.UNSPECIFIED.);
#1324=B_SPLINE_CURVE_WITH_KNOTS('',2,(#73985,#73986,#73987),
 .UNSPECIFIED.,.F.,.F.,(3,3),(0.,1.),.UNSPECIFIED.);
#1325=B_SPLINE_CURVE_WITH_KNOTS('',2,(#73990,#73991,#73992),
 .UNSPECIFIED.,.F.,.F.,(3,3),(0.,1.),.UNSPECIFIED.);
#1326=B_SPLINE_CURVE_WITH_KNOTS('',2,(#74000,#74001,#74002),
 .UNSPECIFIED.,.F.,.F.,(3,3),(0.,1.),.UNSPECIFIED.);
#1327=B_SPLINE_CURVE_WITH_KNOTS('',2,(#74005,#74006,#74007),
 .UNSPECIFIED.,.F.,.F.,(3,3),(0.,1.),.UNSPECIFIED.);
#1328=B_SPLINE_CURVE_WITH_KNOTS('',2,(#74015,#74016,#74017),
 .UNSPECIFIED.,.F.,.F.,(3,3),(0.,1.),.UNSPECIFIED.);
#1329=B_SPLINE_CURVE_WITH_KNOTS('',2,(#74020,#74021,#74022),
 .UNSPECIFIED.,.F.,.F.,(3,3),(0.,1.),.UNSPECIFIED.);
#1330=B_SPLINE_CURVE_WITH_KNOTS('',2,(#74030,#74031,#74032),
 .UNSPECIFIED.,.F.,.F.,(3,3),(0.,1.),.UNSPECIFIED.);
#1331=B_SPLINE_CURVE_WITH_KNOTS('',2,(#74035,#74036,#74037),
 .UNSPECIFIED.,.F.,.F.,(3,3),(0.,1.),.UNSPECIFIED.);
#1332=B_SPLINE_CURVE_WITH_KNOTS('',2,(#74045,#74046,#74047),
 .UNSPECIFIED.,.F.,.F.,(3,3),(0.,1.),.UNSPECIFIED.);
#1333=B_SPLINE_CURVE_WITH_KNOTS('',2,(#74050,#74051,#74052),
 .UNSPECIFIED.,.F.,.F.,(3,3),(0.,1.),.UNSPECIFIED.);
#1334=B_SPLINE_CURVE_WITH_KNOTS('',2,(#74065,#74066,#74067),
 .UNSPECIFIED.,.F.,.F.,(3,3),(0.,1.),.UNSPECIFIED.);
#1335=B_SPLINE_CURVE_WITH_KNOTS('',2,(#74068,#74069,#74070),
 .UNSPECIFIED.,.F.,.F.,(3,3),(0.,1.),.UNSPECIFIED.);
#1336=B_SPLINE_CURVE_WITH_KNOTS('',2,(#74081,#74082,#74083),
 .UNSPECIFIED.,.F.,.F.,(3,3),(0.,1.),.UNSPECIFIED.);
#1337=B_SPLINE_CURVE_WITH_KNOTS('',2,(#74087,#74088,#74089),
 .UNSPECIFIED.,.F.,.F.,(3,3),(0.,1.),.UNSPECIFIED.);
#1338=B_SPLINE_CURVE_WITH_KNOTS('',2,(#74098,#74099,#74100),
 .UNSPECIFIED.,.F.,.F.,(3,3),(0.,1.),.UNSPECIFIED.);
#1339=B_SPLINE_CURVE_WITH_KNOTS('',2,(#74103,#74104,#74105),
 .UNSPECIFIED.,.F.,.F.,(3,3),(0.,1.),.UNSPECIFIED.);
#1340=B_SPLINE_CURVE_WITH_KNOTS('',2,(#74113,#74114,#74115),
 .UNSPECIFIED.,.F.,.F.,(3,3),(0.,1.),.UNSPECIFIED.);
#1341=B_SPLINE_CURVE_WITH_KNOTS('',2,(#74118,#74119,#74120),
 .UNSPECIFIED.,.F.,.F.,(3,3),(0.,1.),.UNSPECIFIED.);
#1342=B_SPLINE_CURVE_WITH_KNOTS('',2,(#74128,#74129,#74130),
 .UNSPECIFIED.,.F.,.F.,(3,3),(0.,1.),.UNSPECIFIED.);
#1343=B_SPLINE_CURVE_WITH_KNOTS('',2,(#74133,#74134,#74135),
 .UNSPECIFIED.,.F.,.F.,(3,3),(0.,1.),.UNSPECIFIED.);
#1344=B_SPLINE_CURVE_WITH_KNOTS('',2,(#74143,#74144,#74145),
 .UNSPECIFIED.,.F.,.F.,(3,3),(0.,1.),.UNSPECIFIED.);
#1345=B_SPLINE_CURVE_WITH_KNOTS('',2,(#74148,#74149,#74150),
 .UNSPECIFIED.,.F.,.F.,(3,3),(0.,1.),.UNSPECIFIED.);
#1346=B_SPLINE_CURVE_WITH_KNOTS('',2,(#74158,#74159,#74160),
 .UNSPECIFIED.,.F.,.F.,(3,3),(0.,1.),.UNSPECIFIED.);
#1347=B_SPLINE_CURVE_WITH_KNOTS('',2,(#74163,#74164,#74165),
 .UNSPECIFIED.,.F.,.F.,(3,3),(0.,1.),.UNSPECIFIED.);
#1348=B_SPLINE_CURVE_WITH_KNOTS('',2,(#74173,#74174,#74175),
 .UNSPECIFIED.,.F.,.F.,(3,3),(0.,1.),.UNSPECIFIED.);
#1349=B_SPLINE_CURVE_WITH_KNOTS('',2,(#74178,#74179,#74180),
 .UNSPECIFIED.,.F.,.F.,(3,3),(0.,1.),.UNSPECIFIED.);
#1350=B_SPLINE_CURVE_WITH_KNOTS('',2,(#74187,#74188,#74189),
 .UNSPECIFIED.,.F.,.F.,(3,3),(0.,1.),.UNSPECIFIED.);
#1351=B_SPLINE_CURVE_WITH_KNOTS('',2,(#74190,#74191,#74192),
 .UNSPECIFIED.,.F.,.F.,(3,3),(0.,1.),.UNSPECIFIED.);
#1352=B_SPLINE_CURVE_WITH_KNOTS('',2,(#74201,#74202,#74203),
 .UNSPECIFIED.,.F.,.F.,(3,3),(0.,1.),.UNSPECIFIED.);
#1353=B_SPLINE_CURVE_WITH_KNOTS('',2,(#74207,#74208,#74209),
 .UNSPECIFIED.,.F.,.F.,(3,3),(0.,1.),.UNSPECIFIED.);
#1354=B_SPLINE_CURVE_WITH_KNOTS('',2,(#74218,#74219,#74220),
 .UNSPECIFIED.,.F.,.F.,(3,3),(0.,1.),.UNSPECIFIED.);
#1355=B_SPLINE_CURVE_WITH_KNOTS('',2,(#74223,#74224,#74225),
 .UNSPECIFIED.,.F.,.F.,(3,3),(0.,1.),.UNSPECIFIED.);
#1356=B_SPLINE_CURVE_WITH_KNOTS('',2,(#74233,#74234,#74235),
 .UNSPECIFIED.,.F.,.F.,(3,3),(0.,1.),.UNSPECIFIED.);
#1357=B_SPLINE_CURVE_WITH_KNOTS('',2,(#74238,#74239,#74240),
 .UNSPECIFIED.,.F.,.F.,(3,3),(0.,1.),.UNSPECIFIED.);
#1358=B_SPLINE_CURVE_WITH_KNOTS('',2,(#74248,#74249,#74250),
 .UNSPECIFIED.,.F.,.F.,(3,3),(0.,1.),.UNSPECIFIED.);
#1359=B_SPLINE_CURVE_WITH_KNOTS('',2,(#74253,#74254,#74255),
 .UNSPECIFIED.,.F.,.F.,(3,3),(0.,1.),.UNSPECIFIED.);
#1360=B_SPLINE_CURVE_WITH_KNOTS('',2,(#74263,#74264,#74265),
 .UNSPECIFIED.,.F.,.F.,(3,3),(0.,1.),.UNSPECIFIED.);
#1361=B_SPLINE_CURVE_WITH_KNOTS('',2,(#74268,#74269,#74270),
 .UNSPECIFIED.,.F.,.F.,(3,3),(0.,1.),.UNSPECIFIED.);
#1362=B_SPLINE_CURVE_WITH_KNOTS('',2,(#74278,#74279,#74280),
 .UNSPECIFIED.,.F.,.F.,(3,3),(0.,1.),.UNSPECIFIED.);
#1363=B_SPLINE_CURVE_WITH_KNOTS('',2,(#74283,#74284,#74285),
 .UNSPECIFIED.,.F.,.F.,(3,3),(0.,1.),.UNSPECIFIED.);
#1364=B_SPLINE_CURVE_WITH_KNOTS('',2,(#74293,#74294,#74295),
 .UNSPECIFIED.,.F.,.F.,(3,3),(0.,1.),.UNSPECIFIED.);
#1365=B_SPLINE_CURVE_WITH_KNOTS('',2,(#74298,#74299,#74300),
 .UNSPECIFIED.,.F.,.F.,(3,3),(0.,1.),.UNSPECIFIED.);
#1366=B_SPLINE_CURVE_WITH_KNOTS('',2,(#74308,#74309,#74310),
 .UNSPECIFIED.,.F.,.F.,(3,3),(0.,1.),.UNSPECIFIED.);
#1367=B_SPLINE_CURVE_WITH_KNOTS('',2,(#74313,#74314,#74315),
 .UNSPECIFIED.,.F.,.F.,(3,3),(0.,1.),.UNSPECIFIED.);
#1368=B_SPLINE_CURVE_WITH_KNOTS('',2,(#74323,#74324,#74325),
 .UNSPECIFIED.,.F.,.F.,(3,3),(0.,1.),.UNSPECIFIED.);
#1369=B_SPLINE_CURVE_WITH_KNOTS('',2,(#74328,#74329,#74330),
 .UNSPECIFIED.,.F.,.F.,(3,3),(0.,1.),.UNSPECIFIED.);
#1370=B_SPLINE_CURVE_WITH_KNOTS('',2,(#74338,#74339,#74340),
 .UNSPECIFIED.,.F.,.F.,(3,3),(0.,1.),.UNSPECIFIED.);
#1371=B_SPLINE_CURVE_WITH_KNOTS('',2,(#74343,#74344,#74345),
 .UNSPECIFIED.,.F.,.F.,(3,3),(0.,1.),.UNSPECIFIED.);
#1372=B_SPLINE_CURVE_WITH_KNOTS('',2,(#74353,#74354,#74355),
 .UNSPECIFIED.,.F.,.F.,(3,3),(0.,1.),.UNSPECIFIED.);
#1373=B_SPLINE_CURVE_WITH_KNOTS('',2,(#74358,#74359,#74360),
 .UNSPECIFIED.,.F.,.F.,(3,3),(0.,1.),.UNSPECIFIED.);
#1374=B_SPLINE_CURVE_WITH_KNOTS('',2,(#74367,#74368,#74369),
 .UNSPECIFIED.,.F.,.F.,(3,3),(0.,1.),.UNSPECIFIED.);
#1375=B_SPLINE_CURVE_WITH_KNOTS('',2,(#74370,#74371,#74372),
 .UNSPECIFIED.,.F.,.F.,(3,3),(0.,1.),.UNSPECIFIED.);
#1718=SHAPE_REPRESENTATION_RELATIONSHIP('SRR','None',#135342,#1731);
#1731=ADVANCED_BREP_SHAPE_REPRESENTATION('',(#1757),#135274);
#1744=STYLED_ITEM('',(#135416),#1757);
#1757=MANIFOLD_SOLID_BREP('Body1',#32080);
#1840=CYLINDRICAL_SURFACE('',#33263,1.1);
#1841=CYLINDRICAL_SURFACE('',#33266,1.1);
#1842=CYLINDRICAL_SURFACE('',#33270,0.799999999999998);
#1843=CYLINDRICAL_SURFACE('',#33274,0.800000000000018);
#1844=CYLINDRICAL_SURFACE('',#33278,0.800000000000025);
#1845=CYLINDRICAL_SURFACE('',#33282,0.799999999999996);
#2078=FACE_BOUND('',#5545,.T.);
#2079=FACE_BOUND('',#5561,.T.);
#2080=FACE_BOUND('',#5585,.T.);
#2081=FACE_BOUND('',#5639,.T.);
#2082=FACE_BOUND('',#5685,.T.);
#2083=FACE_BOUND('',#5718,.T.);
#2084=FACE_BOUND('',#5741,.T.);
#2085=FACE_BOUND('',#5774,.T.);
#2086=FACE_BOUND('',#5820,.T.);
#2087=FACE_BOUND('',#5874,.T.);
#2088=FACE_BOUND('',#5890,.T.);
#2089=FACE_BOUND('',#6329,.T.);
#2090=FACE_BOUND('',#6330,.T.);
#2091=FACE_BOUND('',#6331,.T.);
#2092=FACE_BOUND('',#6332,.T.);
#2093=FACE_BOUND('',#6333,.T.);
#2094=FACE_BOUND('',#6334,.T.);
#2095=FACE_BOUND('',#6335,.T.);
#2096=FACE_BOUND('',#6336,.T.);
#2097=FACE_BOUND('',#6337,.T.);
#2098=FACE_BOUND('',#6338,.T.);
#2099=FACE_BOUND('',#6339,.T.);
#2100=FACE_BOUND('',#6340,.T.);
#2101=FACE_BOUND('',#6341,.T.);
#2102=FACE_BOUND('',#6342,.T.);
#2103=FACE_BOUND('',#6343,.T.);
#2104=FACE_BOUND('',#6344,.T.);
#2105=FACE_BOUND('',#6345,.T.);
#2106=FACE_BOUND('',#6346,.T.);
#2107=FACE_BOUND('',#6347,.T.);
#2108=FACE_BOUND('',#6348,.T.);
#2109=FACE_BOUND('',#6349,.T.);
#2110=FACE_BOUND('',#6350,.T.);
#2111=FACE_BOUND('',#6351,.T.);
#2112=FACE_BOUND('',#6352,.T.);
#2113=FACE_BOUND('',#6353,.T.);
#2114=FACE_BOUND('',#6354,.T.);
#2115=FACE_BOUND('',#6355,.T.);
#2116=FACE_BOUND('',#6356,.T.);
#2117=FACE_BOUND('',#6357,.T.);
#2118=FACE_BOUND('',#6358,.T.);
#2119=FACE_BOUND('',#6359,.T.);
#2120=FACE_BOUND('',#6360,.T.);
#2121=FACE_BOUND('',#6361,.T.);
#2122=FACE_BOUND('',#6362,.T.);
#2123=FACE_BOUND('',#6363,.T.);
#2124=FACE_BOUND('',#6364,.T.);
#2125=FACE_BOUND('',#6365,.T.);
#2126=FACE_BOUND('',#6366,.T.);
#2127=FACE_BOUND('',#6367,.T.);
#2128=FACE_BOUND('',#6368,.T.);
#2129=FACE_BOUND('',#6369,.T.);
#2130=FACE_BOUND('',#6370,.T.);
#2131=FACE_BOUND('',#6371,.T.);
#2132=FACE_BOUND('',#6372,.T.);
#2133=FACE_BOUND('',#6373,.T.);
#2134=FACE_BOUND('',#6374,.T.);
#2135=FACE_BOUND('',#6375,.T.);
#2136=FACE_BOUND('',#6376,.T.);
#2137=FACE_BOUND('',#6377,.T.);
#2138=FACE_BOUND('',#6378,.T.);
#2139=FACE_BOUND('',#6379,.T.);
#2140=FACE_BOUND('',#6380,.T.);
#2141=FACE_BOUND('',#6381,.T.);
#2142=FACE_BOUND('',#6382,.T.);
#2143=FACE_BOUND('',#6383,.T.);
#2144=FACE_BOUND('',#6384,.T.);
#2145=FACE_BOUND('',#6385,.T.);
#2146=FACE_BOUND('',#6386,.T.);
#2147=FACE_BOUND('',#6387,.T.);
#2148=FACE_BOUND('',#6388,.T.);
#2149=FACE_BOUND('',#6389,.T.);
#2150=FACE_BOUND('',#6390,.T.);
#2151=FACE_BOUND('',#6391,.T.);
#2152=FACE_BOUND('',#6392,.T.);
#2153=FACE_BOUND('',#6393,.T.);
#2154=FACE_BOUND('',#6394,.T.);
#2155=FACE_BOUND('',#6395,.T.);
#2156=FACE_BOUND('',#6396,.T.);
#2157=FACE_BOUND('',#6397,.T.);
#2158=FACE_BOUND('',#6398,.T.);
#2159=FACE_BOUND('',#6399,.T.);
#2160=FACE_BOUND('',#6400,.T.);
#2161=FACE_BOUND('',#6401,.T.);
#2162=FACE_BOUND('',#6402,.T.);
#2163=FACE_BOUND('',#6403,.T.);
#2164=FACE_BOUND('',#6404,.T.);
#2165=FACE_BOUND('',#6405,.T.);
#2166=FACE_BOUND('',#6406,.T.);
#2167=FACE_BOUND('',#6407,.T.);
#2168=FACE_BOUND('',#6408,.T.);
#2169=FACE_BOUND('',#6409,.T.);
#2170=FACE_BOUND('',#6410,.T.);
#2171=FACE_BOUND('',#6411,.T.);
#2172=FACE_BOUND('',#6412,.T.);
#2173=FACE_BOUND('',#6413,.T.);
#2174=FACE_BOUND('',#6414,.T.);
#2175=FACE_BOUND('',#6415,.T.);
#2176=FACE_BOUND('',#6416,.T.);
#2177=FACE_BOUND('',#6417,.T.);
#2178=FACE_BOUND('',#6418,.T.);
#2179=FACE_BOUND('',#6419,.T.);
#2180=FACE_BOUND('',#6420,.T.);
#2181=FACE_BOUND('',#6421,.T.);
#2182=FACE_BOUND('',#6422,.T.);
#2183=FACE_BOUND('',#6423,.T.);
#2184=FACE_BOUND('',#6424,.T.);
#2185=FACE_BOUND('',#6425,.T.);
#2186=FACE_BOUND('',#6426,.T.);
#2187=FACE_BOUND('',#6427,.T.);
#2188=FACE_BOUND('',#6428,.T.);
#2189=FACE_BOUND('',#6429,.T.);
#2190=FACE_BOUND('',#6430,.T.);
#2191=FACE_BOUND('',#6431,.T.);
#2192=FACE_BOUND('',#6432,.T.);
#2193=FACE_BOUND('',#6434,.T.);
#2194=FACE_BOUND('',#6435,.T.);
#2450=PLANE('',#32758);
#2451=PLANE('',#32759);
#2452=PLANE('',#32760);
#2453=PLANE('',#32761);
#2454=PLANE('',#32762);
#2455=PLANE('',#32763);
#2456=PLANE('',#32764);
#2457=PLANE('',#32765);
#2458=PLANE('',#32766);
#2459=PLANE('',#32767);
#2460=PLANE('',#32768);
#2461=PLANE('',#32769);
#2462=PLANE('',#32770);
#2463=PLANE('',#32771);
#2464=PLANE('',#32772);
#2465=PLANE('',#32773);
#2466=PLANE('',#32774);
#2467=PLANE('',#32775);
#2468=PLANE('',#32776);
#2469=PLANE('',#32777);
#2470=PLANE('',#32778);
#2471=PLANE('',#32779);
#2472=PLANE('',#32780);
#2473=PLANE('',#32781);
#2474=PLANE('',#32782);
#2475=PLANE('',#32783);
#2476=PLANE('',#32784);
#2477=PLANE('',#32785);
#2478=PLANE('',#32786);
#2479=PLANE('',#32787);
#2480=PLANE('',#32788);
#2481=PLANE('',#32789);
#2482=PLANE('',#32790);
#2483=PLANE('',#32791);
#2484=PLANE('',#32792);
#2485=PLANE('',#32793);
#2486=PLANE('',#32794);
#2487=PLANE('',#32795);
#2488=PLANE('',#32796);
#2489=PLANE('',#32797);
#2490=PLANE('',#32798);
#2491=PLANE('',#32799);
#2492=PLANE('',#32800);
#2493=PLANE('',#32801);
#2494=PLANE('',#32802);
#2495=PLANE('',#32803);
#2496=PLANE('',#32804);
#2497=PLANE('',#32805);
#2498=PLANE('',#32806);
#2499=PLANE('',#32807);
#2500=PLANE('',#32808);
#2501=PLANE('',#32809);
#2502=PLANE('',#32810);
#2503=PLANE('',#32811);
#2504=PLANE('',#32812);
#2505=PLANE('',#32813);
#2506=PLANE('',#32814);
#2507=PLANE('',#32815);
#2508=PLANE('',#32816);
#2509=PLANE('',#32817);
#2510=PLANE('',#32818);
#2511=PLANE('',#32819);
#2512=PLANE('',#32820);
#2513=PLANE('',#32821);
#2514=PLANE('',#32822);
#2515=PLANE('',#32823);
#2516=PLANE('',#32824);
#2517=PLANE('',#32825);
#2518=PLANE('',#32826);
#2519=PLANE('',#32827);
#2520=PLANE('',#32828);
#2521=PLANE('',#32829);
#2522=PLANE('',#32830);
#2523=PLANE('',#32831);
#2524=PLANE('',#32832);
#2525=PLANE('',#32833);
#2526=PLANE('',#32834);
#2527=PLANE('',#32835);
#2528=PLANE('',#32836);
#2529=PLANE('',#32837);
#2530=PLANE('',#32838);
#2531=PLANE('',#32839);
#2532=PLANE('',#32840);
#2533=PLANE('',#32841);
#2534=PLANE('',#32842);
#2535=PLANE('',#32843);
#2536=PLANE('',#32844);
#2537=PLANE('',#32845);
#2538=PLANE('',#32846);
#2539=PLANE('',#32847);
#2540=PLANE('',#32848);
#2541=PLANE('',#32849);
#2542=PLANE('',#32850);
#2543=PLANE('',#32851);
#2544=PLANE('',#32852);
#2545=PLANE('',#32853);
#2546=PLANE('',#32854);
#2547=PLANE('',#32855);
#2548=PLANE('',#32856);
#2549=PLANE('',#32857);
#2550=PLANE('',#32858);
#2551=PLANE('',#32859);
#2552=PLANE('',#32860);
#2553=PLANE('',#32861);
#2554=PLANE('',#32862);
#2555=PLANE('',#32863);
#2556=PLANE('',#32864);
#2557=PLANE('',#32865);
#2558=PLANE('',#32866);
#2559=PLANE('',#32867);
#2560=PLANE('',#32868);
#2561=PLANE('',#32869);
#2562=PLANE('',#32870);
#2563=PLANE('',#32871);
#2564=PLANE('',#32872);
#2565=PLANE('',#32873);
#2566=PLANE('',#32874);
#2567=PLANE('',#32875);
#2568=PLANE('',#32876);
#2569=PLANE('',#32877);
#2570=PLANE('',#32878);
#2571=PLANE('',#32879);
#2572=PLANE('',#32880);
#2573=PLANE('',#32881);
#2574=PLANE('',#32882);
#2575=PLANE('',#32883);
#2576=PLANE('',#32884);
#2577=PLANE('',#32885);
#2578=PLANE('',#32886);
#2579=PLANE('',#32887);
#2580=PLANE('',#32888);
#2581=PLANE('',#32889);
#2582=PLANE('',#32890);
#2583=PLANE('',#32891);
#2584=PLANE('',#32892);
#2585=PLANE('',#32893);
#2586=PLANE('',#32894);
#2587=PLANE('',#32895);
#2588=PLANE('',#32896);
#2589=PLANE('',#32897);
#2590=PLANE('',#32898);
#2591=PLANE('',#32899);
#2592=PLANE('',#32900);
#2593=PLANE('',#32901);
#2594=PLANE('',#32902);
#2595=PLANE('',#32903);
#2596=PLANE('',#32904);
#2597=PLANE('',#32905);
#2598=PLANE('',#32906);
#2599=PLANE('',#32907);
#2600=PLANE('',#32908);
#2601=PLANE('',#32909);
#2602=PLANE('',#32910);
#2603=PLANE('',#32911);
#2604=PLANE('',#32912);
#2605=PLANE('',#32913);
#2606=PLANE('',#32914);
#2607=PLANE('',#32915);
#2608=PLANE('',#32916);
#2609=PLANE('',#32917);
#2610=PLANE('',#32918);
#2611=PLANE('',#32919);
#2612=PLANE('',#32920);
#2613=PLANE('',#32921);
#2614=PLANE('',#32922);
#2615=PLANE('',#32923);
#2616=PLANE('',#32924);
#2617=PLANE('',#32925);
#2618=PLANE('',#32926);
#2619=PLANE('',#32927);
#2620=PLANE('',#32928);
#2621=PLANE('',#32929);
#2622=PLANE('',#32930);
#2623=PLANE('',#32931);
#2624=PLANE('',#32932);
#2625=PLANE('',#32933);
#2626=PLANE('',#32934);
#2627=PLANE('',#32935);
#2628=PLANE('',#32936);
#2629=PLANE('',#32937);
#2630=PLANE('',#32938);
#2631=PLANE('',#32939);
#2632=PLANE('',#32940);
#2633=PLANE('',#32941);
#2634=PLANE('',#32942);
#2635=PLANE('',#32943);
#2636=PLANE('',#32944);
#2637=PLANE('',#32945);
#2638=PLANE('',#32946);
#2639=PLANE('',#32947);
#2640=PLANE('',#32948);
#2641=PLANE('',#32949);
#2642=PLANE('',#32950);
#2643=PLANE('',#32951);
#2644=PLANE('',#32952);
#2645=PLANE('',#32953);
#2646=PLANE('',#32954);
#2647=PLANE('',#32955);
#2648=PLANE('',#32956);
#2649=PLANE('',#32957);
#2650=PLANE('',#32958);
#2651=PLANE('',#32959);
#2652=PLANE('',#32960);
#2653=PLANE('',#32961);
#2654=PLANE('',#32962);
#2655=PLANE('',#32963);
#2656=PLANE('',#32964);
#2657=PLANE('',#32965);
#2658=PLANE('',#32966);
#2659=PLANE('',#32967);
#2660=PLANE('',#32968);
#2661=PLANE('',#32969);
#2662=PLANE('',#32970);
#2663=PLANE('',#32971);
#2664=PLANE('',#32972);
#2665=PLANE('',#32973);
#2666=PLANE('',#32974);
#2667=PLANE('',#32975);
#2668=PLANE('',#32976);
#2669=PLANE('',#32977);
#2670=PLANE('',#32978);
#2671=PLANE('',#32979);
#2672=PLANE('',#32980);
#2673=PLANE('',#32981);
#2674=PLANE('',#32982);
#2675=PLANE('',#32983);
#2676=PLANE('',#32984);
#2677=PLANE('',#32985);
#2678=PLANE('',#32986);
#2679=PLANE('',#32987);
#2680=PLANE('',#32988);
#2681=PLANE('',#32989);
#2682=PLANE('',#32990);
#2683=PLANE('',#32991);
#2684=PLANE('',#32992);
#2685=PLANE('',#32993);
#2686=PLANE('',#32994);
#2687=PLANE('',#32995);
#2688=PLANE('',#32996);
#2689=PLANE('',#32997);
#2690=PLANE('',#32998);
#2691=PLANE('',#32999);
#2692=PLANE('',#33000);
#2693=PLANE('',#33001);
#2694=PLANE('',#33002);
#2695=PLANE('',#33003);
#2696=PLANE('',#33004);
#2697=PLANE('',#33005);
#2698=PLANE('',#33006);
#2699=PLANE('',#33007);
#2700=PLANE('',#33008);
#2701=PLANE('',#33009);
#2702=PLANE('',#33010);
#2703=PLANE('',#33011);
#2704=PLANE('',#33012);
#2705=PLANE('',#33013);
#2706=PLANE('',#33014);
#2707=PLANE('',#33015);
#2708=PLANE('',#33016);
#2709=PLANE('',#33017);
#2710=PLANE('',#33018);
#2711=PLANE('',#33019);
#2712=PLANE('',#33020);
#2713=PLANE('',#33021);
#2714=PLANE('',#33022);
#2715=PLANE('',#33023);
#2716=PLANE('',#33024);
#2717=PLANE('',#33025);
#2718=PLANE('',#33026);
#2719=PLANE('',#33027);
#2720=PLANE('',#33028);
#2721=PLANE('',#33029);
#2722=PLANE('',#33030);
#2723=PLANE('',#33031);
#2724=PLANE('',#33032);
#2725=PLANE('',#33033);
#2726=PLANE('',#33034);
#2727=PLANE('',#33035);
#2728=PLANE('',#33036);
#2729=PLANE('',#33037);
#2730=PLANE('',#33038);
#2731=PLANE('',#33039);
#2732=PLANE('',#33040);
#2733=PLANE('',#33041);
#2734=PLANE('',#33042);
#2735=PLANE('',#33043);
#2736=PLANE('',#33044);
#2737=PLANE('',#33045);
#2738=PLANE('',#33046);
#2739=PLANE('',#33047);
#2740=PLANE('',#33048);
#2741=PLANE('',#33049);
#2742=PLANE('',#33050);
#2743=PLANE('',#33051);
#2744=PLANE('',#33052);
#2745=PLANE('',#33053);
#2746=PLANE('',#33054);
#2747=PLANE('',#33055);
#2748=PLANE('',#33056);
#2749=PLANE('',#33057);
#2750=PLANE('',#33058);
#2751=PLANE('',#33059);
#2752=PLANE('',#33060);
#2753=PLANE('',#33061);
#2754=PLANE('',#33062);
#2755=PLANE('',#33063);
#2756=PLANE('',#33064);
#2757=PLANE('',#33065);
#2758=PLANE('',#33066);
#2759=PLANE('',#33067);
#2760=PLANE('',#33068);
#2761=PLANE('',#33069);
#2762=PLANE('',#33070);
#2763=PLANE('',#33071);
#2764=PLANE('',#33072);
#2765=PLANE('',#33073);
#2766=PLANE('',#33074);
#2767=PLANE('',#33075);
#2768=PLANE('',#33076);
#2769=PLANE('',#33077);
#2770=PLANE('',#33078);
#2771=PLANE('',#33079);
#2772=PLANE('',#33080);
#2773=PLANE('',#33081);
#2774=PLANE('',#33082);
#2775=PLANE('',#33083);
#2776=PLANE('',#33084);
#2777=PLANE('',#33085);
#2778=PLANE('',#33086);
#2779=PLANE('',#33087);
#2780=PLANE('',#33088);
#2781=PLANE('',#33089);
#2782=PLANE('',#33090);
#2783=PLANE('',#33091);
#2784=PLANE('',#33092);
#2785=PLANE('',#33093);
#2786=PLANE('',#33094);
#2787=PLANE('',#33095);
#2788=PLANE('',#33096);
#2789=PLANE('',#33097);
#2790=PLANE('',#33098);
#2791=PLANE('',#33099);
#2792=PLANE('',#33100);
#2793=PLANE('',#33101);
#2794=PLANE('',#33102);
#2795=PLANE('',#33103);
#2796=PLANE('',#33104);
#2797=PLANE('',#33105);
#2798=PLANE('',#33106);
#2799=PLANE('',#33107);
#2800=PLANE('',#33108);
#2801=PLANE('',#33109);
#2802=PLANE('',#33110);
#2803=PLANE('',#33111);
#2804=PLANE('',#33112);
#2805=PLANE('',#33113);
#2806=PLANE('',#33114);
#2807=PLANE('',#33115);
#2808=PLANE('',#33116);
#2809=PLANE('',#33117);
#2810=PLANE('',#33118);
#2811=PLANE('',#33119);
#2812=PLANE('',#33120);
#2813=PLANE('',#33121);
#2814=PLANE('',#33122);
#2815=PLANE('',#33123);
#2816=PLANE('',#33124);
#2817=PLANE('',#33125);
#2818=PLANE('',#33126);
#2819=PLANE('',#33127);
#2820=PLANE('',#33128);
#2821=PLANE('',#33129);
#2822=PLANE('',#33130);
#2823=PLANE('',#33131);
#2824=PLANE('',#33132);
#2825=PLANE('',#33133);
#2826=PLANE('',#33134);
#2827=PLANE('',#33135);
#2828=PLANE('',#33136);
#2829=PLANE('',#33137);
#2830=PLANE('',#33138);
#2831=PLANE('',#33139);
#2832=PLANE('',#33140);
#2833=PLANE('',#33141);
#2834=PLANE('',#33142);
#2835=PLANE('',#33143);
#2836=PLANE('',#33144);
#2837=PLANE('',#33145);
#2838=PLANE('',#33146);
#2839=PLANE('',#33147);
#2840=PLANE('',#33148);
#2841=PLANE('',#33149);
#2842=PLANE('',#33150);
#2843=PLANE('',#33151);
#2844=PLANE('',#33152);
#2845=PLANE('',#33153);
#2846=PLANE('',#33154);
#2847=PLANE('',#33155);
#2848=PLANE('',#33156);
#2849=PLANE('',#33157);
#2850=PLANE('',#33158);
#2851=PLANE('',#33159);
#2852=PLANE('',#33160);
#2853=PLANE('',#33161);
#2854=PLANE('',#33162);
#2855=PLANE('',#33163);
#2856=PLANE('',#33164);
#2857=PLANE('',#33165);
#2858=PLANE('',#33166);
#2859=PLANE('',#33167);
#2860=PLANE('',#33168);
#2861=PLANE('',#33169);
#2862=PLANE('',#33170);
#2863=PLANE('',#33171);
#2864=PLANE('',#33172);
#2865=PLANE('',#33173);
#2866=PLANE('',#33174);
#2867=PLANE('',#33175);
#2868=PLANE('',#33176);
#2869=PLANE('',#33177);
#2870=PLANE('',#33178);
#2871=PLANE('',#33179);
#2872=PLANE('',#33180);
#2873=PLANE('',#33181);
#2874=PLANE('',#33182);
#2875=PLANE('',#33183);
#2876=PLANE('',#33184);
#2877=PLANE('',#33185);
#2878=PLANE('',#33186);
#2879=PLANE('',#33187);
#2880=PLANE('',#33188);
#2881=PLANE('',#33189);
#2882=PLANE('',#33190);
#2883=PLANE('',#33191);
#2884=PLANE('',#33192);
#2885=PLANE('',#33193);
#2886=PLANE('',#33194);
#2887=PLANE('',#33195);
#2888=PLANE('',#33196);
#2889=PLANE('',#33197);
#2890=PLANE('',#33198);
#2891=PLANE('',#33199);
#2892=PLANE('',#33200);
#2893=PLANE('',#33201);
#2894=PLANE('',#33202);
#2895=PLANE('',#33203);
#2896=PLANE('',#33204);
#2897=PLANE('',#33205);
#2898=PLANE('',#33206);
#2899=PLANE('',#33207);
#2900=PLANE('',#33208);
#2901=PLANE('',#33209);
#2902=PLANE('',#33210);
#2903=PLANE('',#33211);
#2904=PLANE('',#33212);
#2905=PLANE('',#33213);
#2906=PLANE('',#33214);
#2907=PLANE('',#33215);
#2908=PLANE('',#33216);
#2909=PLANE('',#33217);
#2910=PLANE('',#33218);
#2911=PLANE('',#33219);
#2912=PLANE('',#33220);
#2913=PLANE('',#33221);
#2914=PLANE('',#33222);
#2915=PLANE('',#33223);
#2916=PLANE('',#33224);
#2917=PLANE('',#33225);
#2918=PLANE('',#33226);
#2919=PLANE('',#33227);
#2920=PLANE('',#33228);
#2921=PLANE('',#33229);
#2922=PLANE('',#33230);
#2923=PLANE('',#33231);
#2924=PLANE('',#33232);
#2925=PLANE('',#33233);
#2926=PLANE('',#33234);
#2927=PLANE('',#33235);
#2928=PLANE('',#33236);
#2929=PLANE('',#33237);
#2930=PLANE('',#33238);
#2931=PLANE('',#33239);
#2932=PLANE('',#33240);
#2933=PLANE('',#33241);
#2934=PLANE('',#33242);
#2935=PLANE('',#33243);
#2936=PLANE('',#33244);
#2937=PLANE('',#33245);
#2938=PLANE('',#33246);
#2939=PLANE('',#33247);
#2940=PLANE('',#33248);
#2941=PLANE('',#33249);
#2942=PLANE('',#33250);
#2943=PLANE('',#33251);
#2944=PLANE('',#33252);
#2945=PLANE('',#33253);
#2946=PLANE('',#33254);
#2947=PLANE('',#33255);
#2948=PLANE('',#33256);
#2949=PLANE('',#33257);
#2950=PLANE('',#33258);
#2951=PLANE('',#33259);
#2952=PLANE('',#33260);
#2953=PLANE('',#33261);
#2954=PLANE('',#33262);
#2955=PLANE('',#33269);
#2956=PLANE('',#33273);
#2957=PLANE('',#33277);
#2958=PLANE('',#33281);
#2959=PLANE('',#33285);
#2960=PLANE('',#33286);
#3708=FACE_OUTER_BOUND('',#5524,.T.);
#3709=FACE_OUTER_BOUND('',#5525,.T.);
#3710=FACE_OUTER_BOUND('',#5526,.T.);
#3711=FACE_OUTER_BOUND('',#5527,.T.);
#3712=FACE_OUTER_BOUND('',#5528,.T.);
#3713=FACE_OUTER_BOUND('',#5529,.T.);
#3714=FACE_OUTER_BOUND('',#5530,.T.);
#3715=FACE_OUTER_BOUND('',#5531,.T.);
#3716=FACE_OUTER_BOUND('',#5532,.T.);
#3717=FACE_OUTER_BOUND('',#5533,.T.);
#3718=FACE_OUTER_BOUND('',#5534,.T.);
#3719=FACE_OUTER_BOUND('',#5535,.T.);
#3720=FACE_OUTER_BOUND('',#5536,.T.);
#3721=FACE_OUTER_BOUND('',#5537,.T.);
#3722=FACE_OUTER_BOUND('',#5538,.T.);
#3723=FACE_OUTER_BOUND('',#5539,.T.);
#3724=FACE_OUTER_BOUND('',#5540,.T.);
#3725=FACE_OUTER_BOUND('',#5541,.T.);
#3726=FACE_OUTER_BOUND('',#5542,.T.);
#3727=FACE_OUTER_BOUND('',#5543,.T.);
#3728=FACE_OUTER_BOUND('',#5544,.T.);
#3729=FACE_OUTER_BOUND('',#5546,.T.);
#3730=FACE_OUTER_BOUND('',#5547,.T.);
#3731=FACE_OUTER_BOUND('',#5548,.T.);
#3732=FACE_OUTER_BOUND('',#5549,.T.);
#3733=FACE_OUTER_BOUND('',#5550,.T.);
#3734=FACE_OUTER_BOUND('',#5551,.T.);
#3735=FACE_OUTER_BOUND('',#5552,.T.);
#3736=FACE_OUTER_BOUND('',#5553,.T.);
#3737=FACE_OUTER_BOUND('',#5554,.T.);
#3738=FACE_OUTER_BOUND('',#5555,.T.);
#3739=FACE_OUTER_BOUND('',#5556,.T.);
#3740=FACE_OUTER_BOUND('',#5557,.T.);
#3741=FACE_OUTER_BOUND('',#5558,.T.);
#3742=FACE_OUTER_BOUND('',#5559,.T.);
#3743=FACE_OUTER_BOUND('',#5560,.T.);
#3744=FACE_OUTER_BOUND('',#5562,.T.);
#3745=FACE_OUTER_BOUND('',#5563,.T.);
#3746=FACE_OUTER_BOUND('',#5564,.T.);
#3747=FACE_OUTER_BOUND('',#5565,.T.);
#3748=FACE_OUTER_BOUND('',#5566,.T.);
#3749=FACE_OUTER_BOUND('',#5567,.T.);
#3750=FACE_OUTER_BOUND('',#5568,.T.);
#3751=FACE_OUTER_BOUND('',#5569,.T.);
#3752=FACE_OUTER_BOUND('',#5570,.T.);
#3753=FACE_OUTER_BOUND('',#5571,.T.);
#3754=FACE_OUTER_BOUND('',#5572,.T.);
#3755=FACE_OUTER_BOUND('',#5573,.T.);
#3756=FACE_OUTER_BOUND('',#5574,.T.);
#3757=FACE_OUTER_BOUND('',#5575,.T.);
#3758=FACE_OUTER_BOUND('',#5576,.T.);
#3759=FACE_OUTER_BOUND('',#5577,.T.);
#3760=FACE_OUTER_BOUND('',#5578,.T.);
#3761=FACE_OUTER_BOUND('',#5579,.T.);
#3762=FACE_OUTER_BOUND('',#5580,.T.);
#3763=FACE_OUTER_BOUND('',#5581,.T.);
#3764=FACE_OUTER_BOUND('',#5582,.T.);
#3765=FACE_OUTER_BOUND('',#5583,.T.);
#3766=FACE_OUTER_BOUND('',#5584,.T.);
#3767=FACE_OUTER_BOUND('',#5586,.T.);
#3768=FACE_OUTER_BOUND('',#5587,.T.);
#3769=FACE_OUTER_BOUND('',#5588,.T.);
#3770=FACE_OUTER_BOUND('',#5589,.T.);
#3771=FACE_OUTER_BOUND('',#5590,.T.);
#3772=FACE_OUTER_BOUND('',#5591,.T.);
#3773=FACE_OUTER_BOUND('',#5592,.T.);
#3774=FACE_OUTER_BOUND('',#5593,.T.);
#3775=FACE_OUTER_BOUND('',#5594,.T.);
#3776=FACE_OUTER_BOUND('',#5595,.T.);
#3777=FACE_OUTER_BOUND('',#5596,.T.);
#3778=FACE_OUTER_BOUND('',#5597,.T.);
#3779=FACE_OUTER_BOUND('',#5598,.T.);
#3780=FACE_OUTER_BOUND('',#5599,.T.);
#3781=FACE_OUTER_BOUND('',#5600,.T.);
#3782=FACE_OUTER_BOUND('',#5601,.T.);
#3783=FACE_OUTER_BOUND('',#5602,.T.);
#3784=FACE_OUTER_BOUND('',#5603,.T.);
#3785=FACE_OUTER_BOUND('',#5604,.T.);
#3786=FACE_OUTER_BOUND('',#5605,.T.);
#3787=FACE_OUTER_BOUND('',#5606,.T.);
#3788=FACE_OUTER_BOUND('',#5607,.T.);
#3789=FACE_OUTER_BOUND('',#5608,.T.);
#3790=FACE_OUTER_BOUND('',#5609,.T.);
#3791=FACE_OUTER_BOUND('',#5610,.T.);
#3792=FACE_OUTER_BOUND('',#5611,.T.);
#3793=FACE_OUTER_BOUND('',#5612,.T.);
#3794=FACE_OUTER_BOUND('',#5613,.T.);
#3795=FACE_OUTER_BOUND('',#5614,.T.);
#3796=FACE_OUTER_BOUND('',#5615,.T.);
#3797=FACE_OUTER_BOUND('',#5616,.T.);
#3798=FACE_OUTER_BOUND('',#5617,.T.);
#3799=FACE_OUTER_BOUND('',#5618,.T.);
#3800=FACE_OUTER_BOUND('',#5619,.T.);
#3801=FACE_OUTER_BOUND('',#5620,.T.);
#3802=FACE_OUTER_BOUND('',#5621,.T.);
#3803=FACE_OUTER_BOUND('',#5622,.T.);
#3804=FACE_OUTER_BOUND('',#5623,.T.);
#3805=FACE_OUTER_BOUND('',#5624,.T.);
#3806=FACE_OUTER_BOUND('',#5625,.T.);
#3807=FACE_OUTER_BOUND('',#5626,.T.);
#3808=FACE_OUTER_BOUND('',#5627,.T.);
#3809=FACE_OUTER_BOUND('',#5628,.T.);
#3810=FACE_OUTER_BOUND('',#5629,.T.);
#3811=FACE_OUTER_BOUND('',#5630,.T.);
#3812=FACE_OUTER_BOUND('',#5631,.T.);
#3813=FACE_OUTER_BOUND('',#5632,.T.);
#3814=FACE_OUTER_BOUND('',#5633,.T.);
#3815=FACE_OUTER_BOUND('',#5634,.T.);
#3816=FACE_OUTER_BOUND('',#5635,.T.);
#3817=FACE_OUTER_BOUND('',#5636,.T.);
#3818=FACE_OUTER_BOUND('',#5637,.T.);
#3819=FACE_OUTER_BOUND('',#5638,.T.);
#3820=FACE_OUTER_BOUND('',#5640,.T.);
#3821=FACE_OUTER_BOUND('',#5641,.T.);
#3822=FACE_OUTER_BOUND('',#5642,.T.);
#3823=FACE_OUTER_BOUND('',#5643,.T.);
#3824=FACE_OUTER_BOUND('',#5644,.T.);
#3825=FACE_OUTER_BOUND('',#5645,.T.);
#3826=FACE_OUTER_BOUND('',#5646,.T.);
#3827=FACE_OUTER_BOUND('',#5647,.T.);
#3828=FACE_OUTER_BOUND('',#5648,.T.);
#3829=FACE_OUTER_BOUND('',#5649,.T.);
#3830=FACE_OUTER_BOUND('',#5650,.T.);
#3831=FACE_OUTER_BOUND('',#5651,.T.);
#3832=FACE_OUTER_BOUND('',#5652,.T.);
#3833=FACE_OUTER_BOUND('',#5653,.T.);
#3834=FACE_OUTER_BOUND('',#5654,.T.);
#3835=FACE_OUTER_BOUND('',#5655,.T.);
#3836=FACE_OUTER_BOUND('',#5656,.T.);
#3837=FACE_OUTER_BOUND('',#5657,.T.);
#3838=FACE_OUTER_BOUND('',#5658,.T.);
#3839=FACE_OUTER_BOUND('',#5659,.T.);
#3840=FACE_OUTER_BOUND('',#5660,.T.);
#3841=FACE_OUTER_BOUND('',#5661,.T.);
#3842=FACE_OUTER_BOUND('',#5662,.T.);
#3843=FACE_OUTER_BOUND('',#5663,.T.);
#3844=FACE_OUTER_BOUND('',#5664,.T.);
#3845=FACE_OUTER_BOUND('',#5665,.T.);
#3846=FACE_OUTER_BOUND('',#5666,.T.);
#3847=FACE_OUTER_BOUND('',#5667,.T.);
#3848=FACE_OUTER_BOUND('',#5668,.T.);
#3849=FACE_OUTER_BOUND('',#5669,.T.);
#3850=FACE_OUTER_BOUND('',#5670,.T.);
#3851=FACE_OUTER_BOUND('',#5671,.T.);
#3852=FACE_OUTER_BOUND('',#5672,.T.);
#3853=FACE_OUTER_BOUND('',#5673,.T.);
#3854=FACE_OUTER_BOUND('',#5674,.T.);
#3855=FACE_OUTER_BOUND('',#5675,.T.);
#3856=FACE_OUTER_BOUND('',#5676,.T.);
#3857=FACE_OUTER_BOUND('',#5677,.T.);
#3858=FACE_OUTER_BOUND('',#5678,.T.);
#3859=FACE_OUTER_BOUND('',#5679,.T.);
#3860=FACE_OUTER_BOUND('',#5680,.T.);
#3861=FACE_OUTER_BOUND('',#5681,.T.);
#3862=FACE_OUTER_BOUND('',#5682,.T.);
#3863=FACE_OUTER_BOUND('',#5683,.T.);
#3864=FACE_OUTER_BOUND('',#5684,.T.);
#3865=FACE_OUTER_BOUND('',#5686,.T.);
#3866=FACE_OUTER_BOUND('',#5687,.T.);
#3867=FACE_OUTER_BOUND('',#5688,.T.);
#3868=FACE_OUTER_BOUND('',#5689,.T.);
#3869=FACE_OUTER_BOUND('',#5690,.T.);
#3870=FACE_OUTER_BOUND('',#5691,.T.);
#3871=FACE_OUTER_BOUND('',#5692,.T.);
#3872=FACE_OUTER_BOUND('',#5693,.T.);
#3873=FACE_OUTER_BOUND('',#5694,.T.);
#3874=FACE_OUTER_BOUND('',#5695,.T.);
#3875=FACE_OUTER_BOUND('',#5696,.T.);
#3876=FACE_OUTER_BOUND('',#5697,.T.);
#3877=FACE_OUTER_BOUND('',#5698,.T.);
#3878=FACE_OUTER_BOUND('',#5699,.T.);
#3879=FACE_OUTER_BOUND('',#5700,.T.);
#3880=FACE_OUTER_BOUND('',#5701,.T.);
#3881=FACE_OUTER_BOUND('',#5702,.T.);
#3882=FACE_OUTER_BOUND('',#5703,.T.);
#3883=FACE_OUTER_BOUND('',#5704,.T.);
#3884=FACE_OUTER_BOUND('',#5705,.T.);
#3885=FACE_OUTER_BOUND('',#5706,.T.);
#3886=FACE_OUTER_BOUND('',#5707,.T.);
#3887=FACE_OUTER_BOUND('',#5708,.T.);
#3888=FACE_OUTER_BOUND('',#5709,.T.);
#3889=FACE_OUTER_BOUND('',#5710,.T.);
#3890=FACE_OUTER_BOUND('',#5711,.T.);
#3891=FACE_OUTER_BOUND('',#5712,.T.);
#3892=FACE_OUTER_BOUND('',#5713,.T.);
#3893=FACE_OUTER_BOUND('',#5714,.T.);
#3894=FACE_OUTER_BOUND('',#5715,.T.);
#3895=FACE_OUTER_BOUND('',#5716,.T.);
#3896=FACE_OUTER_BOUND('',#5717,.T.);
#3897=FACE_OUTER_BOUND('',#5719,.T.);
#3898=FACE_OUTER_BOUND('',#5720,.T.);
#3899=FACE_OUTER_BOUND('',#5721,.T.);
#3900=FACE_OUTER_BOUND('',#5722,.T.);
#3901=FACE_OUTER_BOUND('',#5723,.T.);
#3902=FACE_OUTER_BOUND('',#5724,.T.);
#3903=FACE_OUTER_BOUND('',#5725,.T.);
#3904=FACE_OUTER_BOUND('',#5726,.T.);
#3905=FACE_OUTER_BOUND('',#5727,.T.);
#3906=FACE_OUTER_BOUND('',#5728,.T.);
#3907=FACE_OUTER_BOUND('',#5729,.T.);
#3908=FACE_OUTER_BOUND('',#5730,.T.);
#3909=FACE_OUTER_BOUND('',#5731,.T.);
#3910=FACE_OUTER_BOUND('',#5732,.T.);
#3911=FACE_OUTER_BOUND('',#5733,.T.);
#3912=FACE_OUTER_BOUND('',#5734,.T.);
#3913=FACE_OUTER_BOUND('',#5735,.T.);
#3914=FACE_OUTER_BOUND('',#5736,.T.);
#3915=FACE_OUTER_BOUND('',#5737,.T.);
#3916=FACE_OUTER_BOUND('',#5738,.T.);
#3917=FACE_OUTER_BOUND('',#5739,.T.);
#3918=FACE_OUTER_BOUND('',#5740,.T.);
#3919=FACE_OUTER_BOUND('',#5742,.T.);
#3920=FACE_OUTER_BOUND('',#5743,.T.);
#3921=FACE_OUTER_BOUND('',#5744,.T.);
#3922=FACE_OUTER_BOUND('',#5745,.T.);
#3923=FACE_OUTER_BOUND('',#5746,.T.);
#3924=FACE_OUTER_BOUND('',#5747,.T.);
#3925=FACE_OUTER_BOUND('',#5748,.T.);
#3926=FACE_OUTER_BOUND('',#5749,.T.);
#3927=FACE_OUTER_BOUND('',#5750,.T.);
#3928=FACE_OUTER_BOUND('',#5751,.T.);
#3929=FACE_OUTER_BOUND('',#5752,.T.);
#3930=FACE_OUTER_BOUND('',#5753,.T.);
#3931=FACE_OUTER_BOUND('',#5754,.T.);
#3932=FACE_OUTER_BOUND('',#5755,.T.);
#3933=FACE_OUTER_BOUND('',#5756,.T.);
#3934=FACE_OUTER_BOUND('',#5757,.T.);
#3935=FACE_OUTER_BOUND('',#5758,.T.);
#3936=FACE_OUTER_BOUND('',#5759,.T.);
#3937=FACE_OUTER_BOUND('',#5760,.T.);
#3938=FACE_OUTER_BOUND('',#5761,.T.);
#3939=FACE_OUTER_BOUND('',#5762,.T.);
#3940=FACE_OUTER_BOUND('',#5763,.T.);
#3941=FACE_OUTER_BOUND('',#5764,.T.);
#3942=FACE_OUTER_BOUND('',#5765,.T.);
#3943=FACE_OUTER_BOUND('',#5766,.T.);
#3944=FACE_OUTER_BOUND('',#5767,.T.);
#3945=FACE_OUTER_BOUND('',#5768,.T.);
#3946=FACE_OUTER_BOUND('',#5769,.T.);
#3947=FACE_OUTER_BOUND('',#5770,.T.);
#3948=FACE_OUTER_BOUND('',#5771,.T.);
#3949=FACE_OUTER_BOUND('',#5772,.T.);
#3950=FACE_OUTER_BOUND('',#5773,.T.);
#3951=FACE_OUTER_BOUND('',#5775,.T.);
#3952=FACE_OUTER_BOUND('',#5776,.T.);
#3953=FACE_OUTER_BOUND('',#5777,.T.);
#3954=FACE_OUTER_BOUND('',#5778,.T.);
#3955=FACE_OUTER_BOUND('',#5779,.T.);
#3956=FACE_OUTER_BOUND('',#5780,.T.);
#3957=FACE_OUTER_BOUND('',#5781,.T.);
#3958=FACE_OUTER_BOUND('',#5782,.T.);
#3959=FACE_OUTER_BOUND('',#5783,.T.);
#3960=FACE_OUTER_BOUND('',#5784,.T.);
#3961=FACE_OUTER_BOUND('',#5785,.T.);
#3962=FACE_OUTER_BOUND('',#5786,.T.);
#3963=FACE_OUTER_BOUND('',#5787,.T.);
#3964=FACE_OUTER_BOUND('',#5788,.T.);
#3965=FACE_OUTER_BOUND('',#5789,.T.);
#3966=FACE_OUTER_BOUND('',#5790,.T.);
#3967=FACE_OUTER_BOUND('',#5791,.T.);
#3968=FACE_OUTER_BOUND('',#5792,.T.);
#3969=FACE_OUTER_BOUND('',#5793,.T.);
#3970=FACE_OUTER_BOUND('',#5794,.T.);
#3971=FACE_OUTER_BOUND('',#5795,.T.);
#3972=FACE_OUTER_BOUND('',#5796,.T.);
#3973=FACE_OUTER_BOUND('',#5797,.T.);
#3974=FACE_OUTER_BOUND('',#5798,.T.);
#3975=FACE_OUTER_BOUND('',#5799,.T.);
#3976=FACE_OUTER_BOUND('',#5800,.T.);
#3977=FACE_OUTER_BOUND('',#5801,.T.);
#3978=FACE_OUTER_BOUND('',#5802,.T.);
#3979=FACE_OUTER_BOUND('',#5803,.T.);
#3980=FACE_OUTER_BOUND('',#5804,.T.);
#3981=FACE_OUTER_BOUND('',#5805,.T.);
#3982=FACE_OUTER_BOUND('',#5806,.T.);
#3983=FACE_OUTER_BOUND('',#5807,.T.);
#3984=FACE_OUTER_BOUND('',#5808,.T.);
#3985=FACE_OUTER_BOUND('',#5809,.T.);
#3986=FACE_OUTER_BOUND('',#5810,.T.);
#3987=FACE_OUTER_BOUND('',#5811,.T.);
#3988=FACE_OUTER_BOUND('',#5812,.T.);
#3989=FACE_OUTER_BOUND('',#5813,.T.);
#3990=FACE_OUTER_BOUND('',#5814,.T.);
#3991=FACE_OUTER_BOUND('',#5815,.T.);
#3992=FACE_OUTER_BOUND('',#5816,.T.);
#3993=FACE_OUTER_BOUND('',#5817,.T.);
#3994=FACE_OUTER_BOUND('',#5818,.T.);
#3995=FACE_OUTER_BOUND('',#5819,.T.);
#3996=FACE_OUTER_BOUND('',#5821,.T.);
#3997=FACE_OUTER_BOUND('',#5822,.T.);
#3998=FACE_OUTER_BOUND('',#5823,.T.);
#3999=FACE_OUTER_BOUND('',#5824,.T.);
#4000=FACE_OUTER_BOUND('',#5825,.T.);
#4001=FACE_OUTER_BOUND('',#5826,.T.);
#4002=FACE_OUTER_BOUND('',#5827,.T.);
#4003=FACE_OUTER_BOUND('',#5828,.T.);
#4004=FACE_OUTER_BOUND('',#5829,.T.);
#4005=FACE_OUTER_BOUND('',#5830,.T.);
#4006=FACE_OUTER_BOUND('',#5831,.T.);
#4007=FACE_OUTER_BOUND('',#5832,.T.);
#4008=FACE_OUTER_BOUND('',#5833,.T.);
#4009=FACE_OUTER_BOUND('',#5834,.T.);
#4010=FACE_OUTER_BOUND('',#5835,.T.);
#4011=FACE_OUTER_BOUND('',#5836,.T.);
#4012=FACE_OUTER_BOUND('',#5837,.T.);
#4013=FACE_OUTER_BOUND('',#5838,.T.);
#4014=FACE_OUTER_BOUND('',#5839,.T.);
#4015=FACE_OUTER_BOUND('',#5840,.T.);
#4016=FACE_OUTER_BOUND('',#5841,.T.);
#4017=FACE_OUTER_BOUND('',#5842,.T.);
#4018=FACE_OUTER_BOUND('',#5843,.T.);
#4019=FACE_OUTER_BOUND('',#5844,.T.);
#4020=FACE_OUTER_BOUND('',#5845,.T.);
#4021=FACE_OUTER_BOUND('',#5846,.T.);
#4022=FACE_OUTER_BOUND('',#5847,.T.);
#4023=FACE_OUTER_BOUND('',#5848,.T.);
#4024=FACE_OUTER_BOUND('',#5849,.T.);
#4025=FACE_OUTER_BOUND('',#5850,.T.);
#4026=FACE_OUTER_BOUND('',#5851,.T.);
#4027=FACE_OUTER_BOUND('',#5852,.T.);
#4028=FACE_OUTER_BOUND('',#5853,.T.);
#4029=FACE_OUTER_BOUND('',#5854,.T.);
#4030=FACE_OUTER_BOUND('',#5855,.T.);
#4031=FACE_OUTER_BOUND('',#5856,.T.);
#4032=FACE_OUTER_BOUND('',#5857,.T.);
#4033=FACE_OUTER_BOUND('',#5858,.T.);
#4034=FACE_OUTER_BOUND('',#5859,.T.);
#4035=FACE_OUTER_BOUND('',#5860,.T.);
#4036=FACE_OUTER_BOUND('',#5861,.T.);
#4037=FACE_OUTER_BOUND('',#5862,.T.);
#4038=FACE_OUTER_BOUND('',#5863,.T.);
#4039=FACE_OUTER_BOUND('',#5864,.T.);
#4040=FACE_OUTER_BOUND('',#5865,.T.);
#4041=FACE_OUTER_BOUND('',#5866,.T.);
#4042=FACE_OUTER_BOUND('',#5867,.T.);
#4043=FACE_OUTER_BOUND('',#5868,.T.);
#4044=FACE_OUTER_BOUND('',#5869,.T.);
#4045=FACE_OUTER_BOUND('',#5870,.T.);
#4046=FACE_OUTER_BOUND('',#5871,.T.);
#4047=FACE_OUTER_BOUND('',#5872,.T.);
#4048=FACE_OUTER_BOUND('',#5873,.T.);
#4049=FACE_OUTER_BOUND('',#5875,.T.);
#4050=FACE_OUTER_BOUND('',#5876,.T.);
#4051=FACE_OUTER_BOUND('',#5877,.T.);
#4052=FACE_OUTER_BOUND('',#5878,.T.);
#4053=FACE_OUTER_BOUND('',#5879,.T.);
#4054=FACE_OUTER_BOUND('',#5880,.T.);
#4055=FACE_OUTER_BOUND('',#5881,.T.);
#4056=FACE_OUTER_BOUND('',#5882,.T.);
#4057=FACE_OUTER_BOUND('',#5883,.T.);
#4058=FACE_OUTER_BOUND('',#5884,.T.);
#4059=FACE_OUTER_BOUND('',#5885,.T.);
#4060=FACE_OUTER_BOUND('',#5886,.T.);
#4061=FACE_OUTER_BOUND('',#5887,.T.);
#4062=FACE_OUTER_BOUND('',#5888,.T.);
#4063=FACE_OUTER_BOUND('',#5889,.T.);
#4064=FACE_OUTER_BOUND('',#5891,.T.);
#4065=FACE_OUTER_BOUND('',#5892,.T.);
#4066=FACE_OUTER_BOUND('',#5893,.T.);
#4067=FACE_OUTER_BOUND('',#5894,.T.);
#4068=FACE_OUTER_BOUND('',#5895,.T.);
#4069=FACE_OUTER_BOUND('',#5896,.T.);
#4070=FACE_OUTER_BOUND('',#5897,.T.);
#4071=FACE_OUTER_BOUND('',#5898,.T.);
#4072=FACE_OUTER_BOUND('',#5899,.T.);
#4073=FACE_OUTER_BOUND('',#5900,.T.);
#4074=FACE_OUTER_BOUND('',#5901,.T.);
#4075=FACE_OUTER_BOUND('',#5902,.T.);
#4076=FACE_OUTER_BOUND('',#5903,.T.);
#4077=FACE_OUTER_BOUND('',#5904,.T.);
#4078=FACE_OUTER_BOUND('',#5905,.T.);
#4079=FACE_OUTER_BOUND('',#5906,.T.);
#4080=FACE_OUTER_BOUND('',#5907,.T.);
#4081=FACE_OUTER_BOUND('',#5908,.T.);
#4082=FACE_OUTER_BOUND('',#5909,.T.);
#4083=FACE_OUTER_BOUND('',#5910,.T.);
#4084=FACE_OUTER_BOUND('',#5911,.T.);
#4085=FACE_OUTER_BOUND('',#5912,.T.);
#4086=FACE_OUTER_BOUND('',#5913,.T.);
#4087=FACE_OUTER_BOUND('',#5914,.T.);
#4088=FACE_OUTER_BOUND('',#5915,.T.);
#4089=FACE_OUTER_BOUND('',#5916,.T.);
#4090=FACE_OUTER_BOUND('',#5917,.T.);
#4091=FACE_OUTER_BOUND('',#5918,.T.);
#4092=FACE_OUTER_BOUND('',#5919,.T.);
#4093=FACE_OUTER_BOUND('',#5920,.T.);
#4094=FACE_OUTER_BOUND('',#5921,.T.);
#4095=FACE_OUTER_BOUND('',#5922,.T.);
#4096=FACE_OUTER_BOUND('',#5923,.T.);
#4097=FACE_OUTER_BOUND('',#5924,.T.);
#4098=FACE_OUTER_BOUND('',#5925,.T.);
#4099=FACE_OUTER_BOUND('',#5926,.T.);
#4100=FACE_OUTER_BOUND('',#5927,.T.);
#4101=FACE_OUTER_BOUND('',#5928,.T.);
#4102=FACE_OUTER_BOUND('',#5929,.T.);
#4103=FACE_OUTER_BOUND('',#5930,.T.);
#4104=FACE_OUTER_BOUND('',#5931,.T.);
#4105=FACE_OUTER_BOUND('',#5932,.T.);
#4106=FACE_OUTER_BOUND('',#5933,.T.);
#4107=FACE_OUTER_BOUND('',#5934,.T.);
#4108=FACE_OUTER_BOUND('',#5935,.T.);
#4109=FACE_OUTER_BOUND('',#5936,.T.);
#4110=FACE_OUTER_BOUND('',#5937,.T.);
#4111=FACE_OUTER_BOUND('',#5938,.T.);
#4112=FACE_OUTER_BOUND('',#5939,.T.);
#4113=FACE_OUTER_BOUND('',#5940,.T.);
#4114=FACE_OUTER_BOUND('',#5941,.T.);
#4115=FACE_OUTER_BOUND('',#5942,.T.);
#4116=FACE_OUTER_BOUND('',#5943,.T.);
#4117=FACE_OUTER_BOUND('',#5944,.T.);
#4118=FACE_OUTER_BOUND('',#5945,.T.);
#4119=FACE_OUTER_BOUND('',#5946,.T.);
#4120=FACE_OUTER_BOUND('',#5947,.T.);
#4121=FACE_OUTER_BOUND('',#5948,.T.);
#4122=FACE_OUTER_BOUND('',#5949,.T.);
#4123=FACE_OUTER_BOUND('',#5950,.T.);
#4124=FACE_OUTER_BOUND('',#5951,.T.);
#4125=FACE_OUTER_BOUND('',#5952,.T.);
#4126=FACE_OUTER_BOUND('',#5953,.T.);
#4127=FACE_OUTER_BOUND('',#5954,.T.);
#4128=FACE_OUTER_BOUND('',#5955,.T.);
#4129=FACE_OUTER_BOUND('',#5956,.T.);
#4130=FACE_OUTER_BOUND('',#5957,.T.);
#4131=FACE_OUTER_BOUND('',#5958,.T.);
#4132=FACE_OUTER_BOUND('',#5959,.T.);
#4133=FACE_OUTER_BOUND('',#5960,.T.);
#4134=FACE_OUTER_BOUND('',#5961,.T.);
#4135=FACE_OUTER_BOUND('',#5962,.T.);
#4136=FACE_OUTER_BOUND('',#5963,.T.);
#4137=FACE_OUTER_BOUND('',#5964,.T.);
#4138=FACE_OUTER_BOUND('',#5965,.T.);
#4139=FACE_OUTER_BOUND('',#5966,.T.);
#4140=FACE_OUTER_BOUND('',#5967,.T.);
#4141=FACE_OUTER_BOUND('',#5968,.T.);
#4142=FACE_OUTER_BOUND('',#5969,.T.);
#4143=FACE_OUTER_BOUND('',#5970,.T.);
#4144=FACE_OUTER_BOUND('',#5971,.T.);
#4145=FACE_OUTER_BOUND('',#5972,.T.);
#4146=FACE_OUTER_BOUND('',#5973,.T.);
#4147=FACE_OUTER_BOUND('',#5974,.T.);
#4148=FACE_OUTER_BOUND('',#5975,.T.);
#4149=FACE_OUTER_BOUND('',#5976,.T.);
#4150=FACE_OUTER_BOUND('',#5977,.T.);
#4151=FACE_OUTER_BOUND('',#5978,.T.);
#4152=FACE_OUTER_BOUND('',#5979,.T.);
#4153=FACE_OUTER_BOUND('',#5980,.T.);
#4154=FACE_OUTER_BOUND('',#5981,.T.);
#4155=FACE_OUTER_BOUND('',#5982,.T.);
#4156=FACE_OUTER_BOUND('',#5983,.T.);
#4157=FACE_OUTER_BOUND('',#5984,.T.);
#4158=FACE_OUTER_BOUND('',#5985,.T.);
#4159=FACE_OUTER_BOUND('',#5986,.T.);
#4160=FACE_OUTER_BOUND('',#5987,.T.);
#4161=FACE_OUTER_BOUND('',#5988,.T.);
#4162=FACE_OUTER_BOUND('',#5989,.T.);
#4163=FACE_OUTER_BOUND('',#5990,.T.);
#4164=FACE_OUTER_BOUND('',#5991,.T.);
#4165=FACE_OUTER_BOUND('',#5992,.T.);
#4166=FACE_OUTER_BOUND('',#5993,.T.);
#4167=FACE_OUTER_BOUND('',#5994,.T.);
#4168=FACE_OUTER_BOUND('',#5995,.T.);
#4169=FACE_OUTER_BOUND('',#5996,.T.);
#4170=FACE_OUTER_BOUND('',#5997,.T.);
#4171=FACE_OUTER_BOUND('',#5998,.T.);
#4172=FACE_OUTER_BOUND('',#5999,.T.);
#4173=FACE_OUTER_BOUND('',#6000,.T.);
#4174=FACE_OUTER_BOUND('',#6001,.T.);
#4175=FACE_OUTER_BOUND('',#6002,.T.);
#4176=FACE_OUTER_BOUND('',#6003,.T.);
#4177=FACE_OUTER_BOUND('',#6004,.T.);
#4178=FACE_OUTER_BOUND('',#6005,.T.);
#4179=FACE_OUTER_BOUND('',#6006,.T.);
#4180=FACE_OUTER_BOUND('',#6007,.T.);
#4181=FACE_OUTER_BOUND('',#6008,.T.);
#4182=FACE_OUTER_BOUND('',#6009,.T.);
#4183=FACE_OUTER_BOUND('',#6010,.T.);
#4184=FACE_OUTER_BOUND('',#6011,.T.);
#4185=FACE_OUTER_BOUND('',#6012,.T.);
#4186=FACE_OUTER_BOUND('',#6013,.T.);
#4187=FACE_OUTER_BOUND('',#6014,.T.);
#4188=FACE_OUTER_BOUND('',#6015,.T.);
#4189=FACE_OUTER_BOUND('',#6016,.T.);
#4190=FACE_OUTER_BOUND('',#6017,.T.);
#4191=FACE_OUTER_BOUND('',#6018,.T.);
#4192=FACE_OUTER_BOUND('',#6019,.T.);
#4193=FACE_OUTER_BOUND('',#6020,.T.);
#4194=FACE_OUTER_BOUND('',#6021,.T.);
#4195=FACE_OUTER_BOUND('',#6022,.T.);
#4196=FACE_OUTER_BOUND('',#6023,.T.);
#4197=FACE_OUTER_BOUND('',#6024,.T.);
#4198=FACE_OUTER_BOUND('',#6025,.T.);
#4199=FACE_OUTER_BOUND('',#6026,.T.);
#4200=FACE_OUTER_BOUND('',#6027,.T.);
#4201=FACE_OUTER_BOUND('',#6028,.T.);
#4202=FACE_OUTER_BOUND('',#6029,.T.);
#4203=FACE_OUTER_BOUND('',#6030,.T.);
#4204=FACE_OUTER_BOUND('',#6031,.T.);
#4205=FACE_OUTER_BOUND('',#6032,.T.);
#4206=FACE_OUTER_BOUND('',#6033,.T.);
#4207=FACE_OUTER_BOUND('',#6034,.T.);
#4208=FACE_OUTER_BOUND('',#6035,.T.);
#4209=FACE_OUTER_BOUND('',#6036,.T.);
#4210=FACE_OUTER_BOUND('',#6037,.T.);
#4211=FACE_OUTER_BOUND('',#6038,.T.);
#4212=FACE_OUTER_BOUND('',#6039,.T.);
#4213=FACE_OUTER_BOUND('',#6040,.T.);
#4214=FACE_OUTER_BOUND('',#6041,.T.);
#4215=FACE_OUTER_BOUND('',#6042,.T.);
#4216=FACE_OUTER_BOUND('',#6043,.T.);
#4217=FACE_OUTER_BOUND('',#6044,.T.);
#4218=FACE_OUTER_BOUND('',#6045,.T.);
#4219=FACE_OUTER_BOUND('',#6046,.T.);
#4220=FACE_OUTER_BOUND('',#6047,.T.);
#4221=FACE_OUTER_BOUND('',#6048,.T.);
#4222=FACE_OUTER_BOUND('',#6049,.T.);
#4223=FACE_OUTER_BOUND('',#6050,.T.);
#4224=FACE_OUTER_BOUND('',#6051,.T.);
#4225=FACE_OUTER_BOUND('',#6052,.T.);
#4226=FACE_OUTER_BOUND('',#6053,.T.);
#4227=FACE_OUTER_BOUND('',#6054,.T.);
#4228=FACE_OUTER_BOUND('',#6055,.T.);
#4229=FACE_OUTER_BOUND('',#6056,.T.);
#4230=FACE_OUTER_BOUND('',#6057,.T.);
#4231=FACE_OUTER_BOUND('',#6058,.T.);
#4232=FACE_OUTER_BOUND('',#6059,.T.);
#4233=FACE_OUTER_BOUND('',#6060,.T.);
#4234=FACE_OUTER_BOUND('',#6061,.T.);
#4235=FACE_OUTER_BOUND('',#6062,.T.);
#4236=FACE_OUTER_BOUND('',#6063,.T.);
#4237=FACE_OUTER_BOUND('',#6064,.T.);
#4238=FACE_OUTER_BOUND('',#6065,.T.);
#4239=FACE_OUTER_BOUND('',#6066,.T.);
#4240=FACE_OUTER_BOUND('',#6067,.T.);
#4241=FACE_OUTER_BOUND('',#6068,.T.);
#4242=FACE_OUTER_BOUND('',#6069,.T.);
#4243=FACE_OUTER_BOUND('',#6070,.T.);
#4244=FACE_OUTER_BOUND('',#6071,.T.);
#4245=FACE_OUTER_BOUND('',#6072,.T.);
#4246=FACE_OUTER_BOUND('',#6073,.T.);
#4247=FACE_OUTER_BOUND('',#6074,.T.);
#4248=FACE_OUTER_BOUND('',#6075,.T.);
#4249=FACE_OUTER_BOUND('',#6076,.T.);
#4250=FACE_OUTER_BOUND('',#6077,.T.);
#4251=FACE_OUTER_BOUND('',#6078,.T.);
#4252=FACE_OUTER_BOUND('',#6079,.T.);
#4253=FACE_OUTER_BOUND('',#6080,.T.);
#4254=FACE_OUTER_BOUND('',#6081,.T.);
#4255=FACE_OUTER_BOUND('',#6082,.T.);
#4256=FACE_OUTER_BOUND('',#6083,.T.);
#4257=FACE_OUTER_BOUND('',#6084,.T.);
#4258=FACE_OUTER_BOUND('',#6085,.T.);
#4259=FACE_OUTER_BOUND('',#6086,.T.);
#4260=FACE_OUTER_BOUND('',#6087,.T.);
#4261=FACE_OUTER_BOUND('',#6088,.T.);
#4262=FACE_OUTER_BOUND('',#6089,.T.);
#4263=FACE_OUTER_BOUND('',#6090,.T.);
#4264=FACE_OUTER_BOUND('',#6091,.T.);
#4265=FACE_OUTER_BOUND('',#6092,.T.);
#4266=FACE_OUTER_BOUND('',#6093,.T.);
#4267=FACE_OUTER_BOUND('',#6094,.T.);
#4268=FACE_OUTER_BOUND('',#6095,.T.);
#4269=FACE_OUTER_BOUND('',#6096,.T.);
#4270=FACE_OUTER_BOUND('',#6097,.T.);
#4271=FACE_OUTER_BOUND('',#6098,.T.);
#4272=FACE_OUTER_BOUND('',#6099,.T.);
#4273=FACE_OUTER_BOUND('',#6100,.T.);
#4274=FACE_OUTER_BOUND('',#6101,.T.);
#4275=FACE_OUTER_BOUND('',#6102,.T.);
#4276=FACE_OUTER_BOUND('',#6103,.T.);
#4277=FACE_OUTER_BOUND('',#6104,.T.);
#4278=FACE_OUTER_BOUND('',#6105,.T.);
#4279=FACE_OUTER_BOUND('',#6106,.T.);
#4280=FACE_OUTER_BOUND('',#6107,.T.);
#4281=FACE_OUTER_BOUND('',#6108,.T.);
#4282=FACE_OUTER_BOUND('',#6109,.T.);
#4283=FACE_OUTER_BOUND('',#6110,.T.);
#4284=FACE_OUTER_BOUND('',#6111,.T.);
#4285=FACE_OUTER_BOUND('',#6112,.T.);
#4286=FACE_OUTER_BOUND('',#6113,.T.);
#4287=FACE_OUTER_BOUND('',#6114,.T.);
#4288=FACE_OUTER_BOUND('',#6115,.T.);
#4289=FACE_OUTER_BOUND('',#6116,.T.);
#4290=FACE_OUTER_BOUND('',#6117,.T.);
#4291=FACE_OUTER_BOUND('',#6118,.T.);
#4292=FACE_OUTER_BOUND('',#6119,.T.);
#4293=FACE_OUTER_BOUND('',#6120,.T.);
#4294=FACE_OUTER_BOUND('',#6121,.T.);
#4295=FACE_OUTER_BOUND('',#6122,.T.);
#4296=FACE_OUTER_BOUND('',#6123,.T.);
#4297=FACE_OUTER_BOUND('',#6124,.T.);
#4298=FACE_OUTER_BOUND('',#6125,.T.);
#4299=FACE_OUTER_BOUND('',#6126,.T.);
#4300=FACE_OUTER_BOUND('',#6127,.T.);
#4301=FACE_OUTER_BOUND('',#6128,.T.);
#4302=FACE_OUTER_BOUND('',#6129,.T.);
#4303=FACE_OUTER_BOUND('',#6130,.T.);
#4304=FACE_OUTER_BOUND('',#6131,.T.);
#4305=FACE_OUTER_BOUND('',#6132,.T.);
#4306=FACE_OUTER_BOUND('',#6133,.T.);
#4307=FACE_OUTER_BOUND('',#6134,.T.);
#4308=FACE_OUTER_BOUND('',#6135,.T.);
#4309=FACE_OUTER_BOUND('',#6136,.T.);
#4310=FACE_OUTER_BOUND('',#6137,.T.);
#4311=FACE_OUTER_BOUND('',#6138,.T.);
#4312=FACE_OUTER_BOUND('',#6139,.T.);
#4313=FACE_OUTER_BOUND('',#6140,.T.);
#4314=FACE_OUTER_BOUND('',#6141,.T.);
#4315=FACE_OUTER_BOUND('',#6142,.T.);
#4316=FACE_OUTER_BOUND('',#6143,.T.);
#4317=FACE_OUTER_BOUND('',#6144,.T.);
#4318=FACE_OUTER_BOUND('',#6145,.T.);
#4319=FACE_OUTER_BOUND('',#6146,.T.);
#4320=FACE_OUTER_BOUND('',#6147,.T.);
#4321=FACE_OUTER_BOUND('',#6148,.T.);
#4322=FACE_OUTER_BOUND('',#6149,.T.);
#4323=FACE_OUTER_BOUND('',#6150,.T.);
#4324=FACE_OUTER_BOUND('',#6151,.T.);
#4325=FACE_OUTER_BOUND('',#6152,.T.);
#4326=FACE_OUTER_BOUND('',#6153,.T.);
#4327=FACE_OUTER_BOUND('',#6154,.T.);
#4328=FACE_OUTER_BOUND('',#6155,.T.);
#4329=FACE_OUTER_BOUND('',#6156,.T.);
#4330=FACE_OUTER_BOUND('',#6157,.T.);
#4331=FACE_OUTER_BOUND('',#6158,.T.);
#4332=FACE_OUTER_BOUND('',#6159,.T.);
#4333=FACE_OUTER_BOUND('',#6160,.T.);
#4334=FACE_OUTER_BOUND('',#6161,.T.);
#4335=FACE_OUTER_BOUND('',#6162,.T.);
#4336=FACE_OUTER_BOUND('',#6163,.T.);
#4337=FACE_OUTER_BOUND('',#6164,.T.);
#4338=FACE_OUTER_BOUND('',#6165,.T.);
#4339=FACE_OUTER_BOUND('',#6166,.T.);
#4340=FACE_OUTER_BOUND('',#6167,.T.);
#4341=FACE_OUTER_BOUND('',#6168,.T.);
#4342=FACE_OUTER_BOUND('',#6169,.T.);
#4343=FACE_OUTER_BOUND('',#6170,.T.);
#4344=FACE_OUTER_BOUND('',#6171,.T.);
#4345=FACE_OUTER_BOUND('',#6172,.T.);
#4346=FACE_OUTER_BOUND('',#6173,.T.);
#4347=FACE_OUTER_BOUND('',#6174,.T.);
#4348=FACE_OUTER_BOUND('',#6175,.T.);
#4349=FACE_OUTER_BOUND('',#6176,.T.);
#4350=FACE_OUTER_BOUND('',#6177,.T.);
#4351=FACE_OUTER_BOUND('',#6178,.T.);
#4352=FACE_OUTER_BOUND('',#6179,.T.);
#4353=FACE_OUTER_BOUND('',#6180,.T.);
#4354=FACE_OUTER_BOUND('',#6181,.T.);
#4355=FACE_OUTER_BOUND('',#6182,.T.);
#4356=FACE_OUTER_BOUND('',#6183,.T.);
#4357=FACE_OUTER_BOUND('',#6184,.T.);
#4358=FACE_OUTER_BOUND('',#6185,.T.);
#4359=FACE_OUTER_BOUND('',#6186,.T.);
#4360=FACE_OUTER_BOUND('',#6187,.T.);
#4361=FACE_OUTER_BOUND('',#6188,.T.);
#4362=FACE_OUTER_BOUND('',#6189,.T.);
#4363=FACE_OUTER_BOUND('',#6190,.T.);
#4364=FACE_OUTER_BOUND('',#6191,.T.);
#4365=FACE_OUTER_BOUND('',#6192,.T.);
#4366=FACE_OUTER_BOUND('',#6193,.T.);
#4367=FACE_OUTER_BOUND('',#6194,.T.);
#4368=FACE_OUTER_BOUND('',#6195,.T.);
#4369=FACE_OUTER_BOUND('',#6196,.T.);
#4370=FACE_OUTER_BOUND('',#6197,.T.);
#4371=FACE_OUTER_BOUND('',#6198,.T.);
#4372=FACE_OUTER_BOUND('',#6199,.T.);
#4373=FACE_OUTER_BOUND('',#6200,.T.);
#4374=FACE_OUTER_BOUND('',#6201,.T.);
#4375=FACE_OUTER_BOUND('',#6202,.T.);
#4376=FACE_OUTER_BOUND('',#6203,.T.);
#4377=FACE_OUTER_BOUND('',#6204,.T.);
#4378=FACE_OUTER_BOUND('',#6205,.T.);
#4379=FACE_OUTER_BOUND('',#6206,.T.);
#4380=FACE_OUTER_BOUND('',#6207,.T.);
#4381=FACE_OUTER_BOUND('',#6208,.T.);
#4382=FACE_OUTER_BOUND('',#6209,.T.);
#4383=FACE_OUTER_BOUND('',#6210,.T.);
#4384=FACE_OUTER_BOUND('',#6211,.T.);
#4385=FACE_OUTER_BOUND('',#6212,.T.);
#4386=FACE_OUTER_BOUND('',#6213,.T.);
#4387=FACE_OUTER_BOUND('',#6214,.T.);
#4388=FACE_OUTER_BOUND('',#6215,.T.);
#4389=FACE_OUTER_BOUND('',#6216,.T.);
#4390=FACE_OUTER_BOUND('',#6217,.T.);
#4391=FACE_OUTER_BOUND('',#6218,.T.);
#4392=FACE_OUTER_BOUND('',#6219,.T.);
#4393=FACE_OUTER_BOUND('',#6220,.T.);
#4394=FACE_OUTER_BOUND('',#6221,.T.);
#4395=FACE_OUTER_BOUND('',#6222,.T.);
#4396=FACE_OUTER_BOUND('',#6223,.T.);
#4397=FACE_OUTER_BOUND('',#6224,.T.);
#4398=FACE_OUTER_BOUND('',#6225,.T.);
#4399=FACE_OUTER_BOUND('',#6226,.T.);
#4400=FACE_OUTER_BOUND('',#6227,.T.);
#4401=FACE_OUTER_BOUND('',#6228,.T.);
#4402=FACE_OUTER_BOUND('',#6229,.T.);
#4403=FACE_OUTER_BOUND('',#6230,.T.);
#4404=FACE_OUTER_BOUND('',#6231,.T.);
#4405=FACE_OUTER_BOUND('',#6232,.T.);
#4406=FACE_OUTER_BOUND('',#6233,.T.);
#4407=FACE_OUTER_BOUND('',#6234,.T.);
#4408=FACE_OUTER_BOUND('',#6235,.T.);
#4409=FACE_OUTER_BOUND('',#6236,.T.);
#4410=FACE_OUTER_BOUND('',#6237,.T.);
#4411=FACE_OUTER_BOUND('',#6238,.T.);
#4412=FACE_OUTER_BOUND('',#6239,.T.);
#4413=FACE_OUTER_BOUND('',#6240,.T.);
#4414=FACE_OUTER_BOUND('',#6241,.T.);
#4415=FACE_OUTER_BOUND('',#6242,.T.);
#4416=FACE_OUTER_BOUND('',#6243,.T.);
#4417=FACE_OUTER_BOUND('',#6244,.T.);
#4418=FACE_OUTER_BOUND('',#6245,.T.);
#4419=FACE_OUTER_BOUND('',#6246,.T.);
#4420=FACE_OUTER_BOUND('',#6247,.T.);
#4421=FACE_OUTER_BOUND('',#6248,.T.);
#4422=FACE_OUTER_BOUND('',#6249,.T.);
#4423=FACE_OUTER_BOUND('',#6250,.T.);
#4424=FACE_OUTER_BOUND('',#6251,.T.);
#4425=FACE_OUTER_BOUND('',#6252,.T.);
#4426=FACE_OUTER_BOUND('',#6253,.T.);
#4427=FACE_OUTER_BOUND('',#6254,.T.);
#4428=FACE_OUTER_BOUND('',#6255,.T.);
#4429=FACE_OUTER_BOUND('',#6256,.T.);
#4430=FACE_OUTER_BOUND('',#6257,.T.);
#4431=FACE_OUTER_BOUND('',#6258,.T.);
#4432=FACE_OUTER_BOUND('',#6259,.T.);
#4433=FACE_OUTER_BOUND('',#6260,.T.);
#4434=FACE_OUTER_BOUND('',#6261,.T.);
#4435=FACE_OUTER_BOUND('',#6262,.T.);
#4436=FACE_OUTER_BOUND('',#6263,.T.);
#4437=FACE_OUTER_BOUND('',#6264,.T.);
#4438=FACE_OUTER_BOUND('',#6265,.T.);
#4439=FACE_OUTER_BOUND('',#6266,.T.);
#4440=FACE_OUTER_BOUND('',#6267,.T.);
#4441=FACE_OUTER_BOUND('',#6268,.T.);
#4442=FACE_OUTER_BOUND('',#6269,.T.);
#4443=FACE_OUTER_BOUND('',#6270,.T.);
#4444=FACE_OUTER_BOUND('',#6271,.T.);
#4445=FACE_OUTER_BOUND('',#6272,.T.);
#4446=FACE_OUTER_BOUND('',#6273,.T.);
#4447=FACE_OUTER_BOUND('',#6274,.T.);
#4448=FACE_OUTER_BOUND('',#6275,.T.);
#4449=FACE_OUTER_BOUND('',#6276,.T.);
#4450=FACE_OUTER_BOUND('',#6277,.T.);
#4451=FACE_OUTER_BOUND('',#6278,.T.);
#4452=FACE_OUTER_BOUND('',#6279,.T.);
#4453=FACE_OUTER_BOUND('',#6280,.T.);
#4454=FACE_OUTER_BOUND('',#6281,.T.);
#4455=FACE_OUTER_BOUND('',#6282,.T.);
#4456=FACE_OUTER_BOUND('',#6283,.T.);
#4457=FACE_OUTER_BOUND('',#6284,.T.);
#4458=FACE_OUTER_BOUND('',#6285,.T.);
#4459=FACE_OUTER_BOUND('',#6286,.T.);
#4460=FACE_OUTER_BOUND('',#6287,.T.);
#4461=FACE_OUTER_BOUND('',#6288,.T.);
#4462=FACE_OUTER_BOUND('',#6289,.T.);
#4463=FACE_OUTER_BOUND('',#6290,.T.);
#4464=FACE_OUTER_BOUND('',#6291,.T.);
#4465=FACE_OUTER_BOUND('',#6292,.T.);
#4466=FACE_OUTER_BOUND('',#6293,.T.);
#4467=FACE_OUTER_BOUND('',#6294,.T.);
#4468=FACE_OUTER_BOUND('',#6295,.T.);
#4469=FACE_OUTER_BOUND('',#6296,.T.);
#4470=FACE_OUTER_BOUND('',#6297,.T.);
#4471=FACE_OUTER_BOUND('',#6298,.T.);
#4472=FACE_OUTER_BOUND('',#6299,.T.);
#4473=FACE_OUTER_BOUND('',#6300,.T.);
#4474=FACE_OUTER_BOUND('',#6301,.T.);
#4475=FACE_OUTER_BOUND('',#6302,.T.);
#4476=FACE_OUTER_BOUND('',#6303,.T.);
#4477=FACE_OUTER_BOUND('',#6304,.T.);
#4478=FACE_OUTER_BOUND('',#6305,.T.);
#4479=FACE_OUTER_BOUND('',#6306,.T.);
#4480=FACE_OUTER_BOUND('',#6307,.T.);
#4481=FACE_OUTER_BOUND('',#6308,.T.);
#4482=FACE_OUTER_BOUND('',#6309,.T.);
#4483=FACE_OUTER_BOUND('',#6310,.T.);
#4484=FACE_OUTER_BOUND('',#6311,.T.);
#4485=FACE_OUTER_BOUND('',#6312,.T.);
#4486=FACE_OUTER_BOUND('',#6313,.T.);
#4487=FACE_OUTER_BOUND('',#6314,.T.);
#4488=FACE_OUTER_BOUND('',#6315,.T.);
#4489=FACE_OUTER_BOUND('',#6316,.T.);
#4490=FACE_OUTER_BOUND('',#6317,.T.);
#4491=FACE_OUTER_BOUND('',#6318,.T.);
#4492=FACE_OUTER_BOUND('',#6319,.T.);
#4493=FACE_OUTER_BOUND('',#6320,.T.);
#4494=FACE_OUTER_BOUND('',#6321,.T.);
#4495=FACE_OUTER_BOUND('',#6322,.T.);
#4496=FACE_OUTER_BOUND('',#6323,.T.);
#4497=FACE_OUTER_BOUND('',#6324,.T.);
#4498=FACE_OUTER_BOUND('',#6325,.T.);
#4499=FACE_OUTER_BOUND('',#6326,.T.);
#4500=FACE_OUTER_BOUND('',#6327,.T.);
#4501=FACE_OUTER_BOUND('',#6328,.T.);
#4502=FACE_OUTER_BOUND('',#6433,.T.);
#5524=EDGE_LOOP('',(#22782,#22783,#22784,#22785));
#5525=EDGE_LOOP('',(#22786,#22787,#22788,#22789));
#5526=EDGE_LOOP('',(#22790,#22791,#22792,#22793));
#5527=EDGE_LOOP('',(#22794,#22795,#22796,#22797));
#5528=EDGE_LOOP('',(#22798,#22799,#22800,#22801));
#5529=EDGE_LOOP('',(#22802,#22803,#22804,#22805));
#5530=EDGE_LOOP('',(#22806,#22807,#22808,#22809));
#5531=EDGE_LOOP('',(#22810,#22811,#22812,#22813));
#5532=EDGE_LOOP('',(#22814,#22815,#22816,#22817));
#5533=EDGE_LOOP('',(#22818,#22819,#22820,#22821));
#5534=EDGE_LOOP('',(#22822,#22823,#22824,#22825));
#5535=EDGE_LOOP('',(#22826,#22827,#22828,#22829));
#5536=EDGE_LOOP('',(#22830,#22831,#22832,#22833));
#5537=EDGE_LOOP('',(#22834,#22835,#22836,#22837));
#5538=EDGE_LOOP('',(#22838,#22839,#22840,#22841));
#5539=EDGE_LOOP('',(#22842,#22843,#22844,#22845));
#5540=EDGE_LOOP('',(#22846,#22847,#22848,#22849));
#5541=EDGE_LOOP('',(#22850,#22851,#22852,#22853));
#5542=EDGE_LOOP('',(#22854,#22855,#22856,#22857));
#5543=EDGE_LOOP('',(#22858,#22859,#22860,#22861));
#5544=EDGE_LOOP('',(#22862,#22863,#22864,#22865,#22866,#22867,#22868,#22869,
#22870,#22871,#22872,#22873));
#5545=EDGE_LOOP('',(#22874,#22875,#22876,#22877,#22878,#22879,#22880,#22881));
#5546=EDGE_LOOP('',(#22882,#22883,#22884,#22885));
#5547=EDGE_LOOP('',(#22886,#22887,#22888,#22889));
#5548=EDGE_LOOP('',(#22890,#22891,#22892,#22893));
#5549=EDGE_LOOP('',(#22894,#22895,#22896,#22897));
#5550=EDGE_LOOP('',(#22898,#22899,#22900,#22901));
#5551=EDGE_LOOP('',(#22902,#22903,#22904,#22905));
#5552=EDGE_LOOP('',(#22906,#22907,#22908,#22909));
#5553=EDGE_LOOP('',(#22910,#22911,#22912,#22913));
#5554=EDGE_LOOP('',(#22914,#22915,#22916,#22917));
#5555=EDGE_LOOP('',(#22918,#22919,#22920,#22921));
#5556=EDGE_LOOP('',(#22922,#22923,#22924,#22925));
#5557=EDGE_LOOP('',(#22926,#22927,#22928,#22929));
#5558=EDGE_LOOP('',(#22930,#22931,#22932,#22933));
#5559=EDGE_LOOP('',(#22934,#22935,#22936,#22937));
#5560=EDGE_LOOP('',(#22938,#22939,#22940,#22941,#22942,#22943,#22944,#22945,
#22946,#22947,#22948));
#5561=EDGE_LOOP('',(#22949,#22950,#22951));
#5562=EDGE_LOOP('',(#22952,#22953,#22954));
#5563=EDGE_LOOP('',(#22955,#22956,#22957,#22958,#22959,#22960,#22961,#22962));
#5564=EDGE_LOOP('',(#22963,#22964,#22965,#22966));
#5565=EDGE_LOOP('',(#22967,#22968,#22969,#22970));
#5566=EDGE_LOOP('',(#22971,#22972,#22973,#22974));
#5567=EDGE_LOOP('',(#22975,#22976,#22977,#22978));
#5568=EDGE_LOOP('',(#22979,#22980,#22981,#22982));
#5569=EDGE_LOOP('',(#22983,#22984,#22985,#22986));
#5570=EDGE_LOOP('',(#22987,#22988,#22989,#22990));
#5571=EDGE_LOOP('',(#22991,#22992,#22993,#22994));
#5572=EDGE_LOOP('',(#22995,#22996,#22997,#22998));
#5573=EDGE_LOOP('',(#22999,#23000,#23001,#23002));
#5574=EDGE_LOOP('',(#23003,#23004,#23005,#23006));
#5575=EDGE_LOOP('',(#23007,#23008,#23009,#23010));
#5576=EDGE_LOOP('',(#23011,#23012,#23013,#23014));
#5577=EDGE_LOOP('',(#23015,#23016,#23017,#23018));
#5578=EDGE_LOOP('',(#23019,#23020,#23021,#23022));
#5579=EDGE_LOOP('',(#23023,#23024,#23025,#23026));
#5580=EDGE_LOOP('',(#23027,#23028,#23029,#23030));
#5581=EDGE_LOOP('',(#23031,#23032,#23033,#23034));
#5582=EDGE_LOOP('',(#23035,#23036,#23037,#23038));
#5583=EDGE_LOOP('',(#23039,#23040,#23041,#23042));
#5584=EDGE_LOOP('',(#23043,#23044,#23045,#23046,#23047,#23048,#23049,#23050,
#23051,#23052,#23053,#23054));
#5585=EDGE_LOOP('',(#23055,#23056,#23057,#23058,#23059,#23060,#23061,#23062));
#5586=EDGE_LOOP('',(#23063,#23064,#23065,#23066));
#5587=EDGE_LOOP('',(#23067,#23068,#23069,#23070));
#5588=EDGE_LOOP('',(#23071,#23072,#23073,#23074));
#5589=EDGE_LOOP('',(#23075,#23076,#23077,#23078));
#5590=EDGE_LOOP('',(#23079,#23080,#23081,#23082));
#5591=EDGE_LOOP('',(#23083,#23084,#23085,#23086));
#5592=EDGE_LOOP('',(#23087,#23088,#23089,#23090));
#5593=EDGE_LOOP('',(#23091,#23092,#23093,#23094));
#5594=EDGE_LOOP('',(#23095,#23096,#23097,#23098));
#5595=EDGE_LOOP('',(#23099,#23100,#23101,#23102));
#5596=EDGE_LOOP('',(#23103,#23104,#23105,#23106));
#5597=EDGE_LOOP('',(#23107,#23108,#23109,#23110));
#5598=EDGE_LOOP('',(#23111,#23112,#23113,#23114));
#5599=EDGE_LOOP('',(#23115,#23116,#23117,#23118));
#5600=EDGE_LOOP('',(#23119,#23120,#23121,#23122));
#5601=EDGE_LOOP('',(#23123,#23124,#23125,#23126));
#5602=EDGE_LOOP('',(#23127,#23128,#23129,#23130));
#5603=EDGE_LOOP('',(#23131,#23132,#23133,#23134));
#5604=EDGE_LOOP('',(#23135,#23136,#23137,#23138));
#5605=EDGE_LOOP('',(#23139,#23140,#23141,#23142));
#5606=EDGE_LOOP('',(#23143,#23144,#23145,#23146));
#5607=EDGE_LOOP('',(#23147,#23148,#23149,#23150));
#5608=EDGE_LOOP('',(#23151,#23152,#23153,#23154));
#5609=EDGE_LOOP('',(#23155,#23156,#23157,#23158));
#5610=EDGE_LOOP('',(#23159,#23160,#23161,#23162));
#5611=EDGE_LOOP('',(#23163,#23164,#23165,#23166));
#5612=EDGE_LOOP('',(#23167,#23168,#23169,#23170));
#5613=EDGE_LOOP('',(#23171,#23172,#23173,#23174));
#5614=EDGE_LOOP('',(#23175,#23176,#23177,#23178));
#5615=EDGE_LOOP('',(#23179,#23180,#23181,#23182));
#5616=EDGE_LOOP('',(#23183,#23184,#23185,#23186,#23187,#23188,#23189,#23190,
#23191,#23192,#23193,#23194,#23195,#23196,#23197,#23198,#23199,#23200,#23201,
#23202,#23203,#23204,#23205,#23206,#23207,#23208,#23209,#23210,#23211,#23212));
#5617=EDGE_LOOP('',(#23213,#23214,#23215,#23216,#23217,#23218,#23219,#23220));
#5618=EDGE_LOOP('',(#23221,#23222,#23223,#23224));
#5619=EDGE_LOOP('',(#23225,#23226,#23227,#23228));
#5620=EDGE_LOOP('',(#23229,#23230,#23231,#23232));
#5621=EDGE_LOOP('',(#23233,#23234,#23235,#23236));
#5622=EDGE_LOOP('',(#23237,#23238,#23239,#23240));
#5623=EDGE_LOOP('',(#23241,#23242,#23243,#23244));
#5624=EDGE_LOOP('',(#23245,#23246,#23247,#23248));
#5625=EDGE_LOOP('',(#23249,#23250,#23251,#23252));
#5626=EDGE_LOOP('',(#23253,#23254,#23255,#23256));
#5627=EDGE_LOOP('',(#23257,#23258,#23259,#23260));
#5628=EDGE_LOOP('',(#23261,#23262,#23263,#23264));
#5629=EDGE_LOOP('',(#23265,#23266,#23267,#23268));
#5630=EDGE_LOOP('',(#23269,#23270,#23271,#23272));
#5631=EDGE_LOOP('',(#23273,#23274,#23275,#23276));
#5632=EDGE_LOOP('',(#23277,#23278,#23279,#23280));
#5633=EDGE_LOOP('',(#23281,#23282,#23283,#23284));
#5634=EDGE_LOOP('',(#23285,#23286,#23287,#23288));
#5635=EDGE_LOOP('',(#23289,#23290,#23291,#23292));
#5636=EDGE_LOOP('',(#23293,#23294,#23295,#23296));
#5637=EDGE_LOOP('',(#23297,#23298,#23299,#23300));
#5638=EDGE_LOOP('',(#23301,#23302,#23303,#23304,#23305,#23306,#23307,#23308,
#23309,#23310,#23311,#23312));
#5639=EDGE_LOOP('',(#23313,#23314,#23315,#23316,#23317,#23318,#23319,#23320));
#5640=EDGE_LOOP('',(#23321,#23322,#23323,#23324));
#5641=EDGE_LOOP('',(#23325,#23326,#23327,#23328));
#5642=EDGE_LOOP('',(#23329,#23330,#23331,#23332));
#5643=EDGE_LOOP('',(#23333,#23334,#23335,#23336));
#5644=EDGE_LOOP('',(#23337,#23338,#23339,#23340));
#5645=EDGE_LOOP('',(#23341,#23342,#23343,#23344));
#5646=EDGE_LOOP('',(#23345,#23346,#23347,#23348));
#5647=EDGE_LOOP('',(#23349,#23350,#23351,#23352));
#5648=EDGE_LOOP('',(#23353,#23354,#23355,#23356));
#5649=EDGE_LOOP('',(#23357,#23358,#23359,#23360));
#5650=EDGE_LOOP('',(#23361,#23362,#23363,#23364));
#5651=EDGE_LOOP('',(#23365,#23366,#23367,#23368));
#5652=EDGE_LOOP('',(#23369,#23370,#23371,#23372));
#5653=EDGE_LOOP('',(#23373,#23374,#23375,#23376));
#5654=EDGE_LOOP('',(#23377,#23378,#23379,#23380));
#5655=EDGE_LOOP('',(#23381,#23382,#23383,#23384));
#5656=EDGE_LOOP('',(#23385,#23386,#23387,#23388));
#5657=EDGE_LOOP('',(#23389,#23390,#23391,#23392));
#5658=EDGE_LOOP('',(#23393,#23394,#23395,#23396));
#5659=EDGE_LOOP('',(#23397,#23398,#23399,#23400));
#5660=EDGE_LOOP('',(#23401,#23402,#23403,#23404));
#5661=EDGE_LOOP('',(#23405,#23406,#23407,#23408));
#5662=EDGE_LOOP('',(#23409,#23410,#23411,#23412,#23413,#23414,#23415,#23416,
#23417,#23418,#23419,#23420,#23421,#23422,#23423,#23424,#23425,#23426,#23427,
#23428,#23429,#23430));
#5663=EDGE_LOOP('',(#23431,#23432,#23433,#23434,#23435,#23436,#23437,#23438));
#5664=EDGE_LOOP('',(#23439,#23440,#23441,#23442));
#5665=EDGE_LOOP('',(#23443,#23444,#23445,#23446));
#5666=EDGE_LOOP('',(#23447,#23448,#23449,#23450));
#5667=EDGE_LOOP('',(#23451,#23452,#23453,#23454));
#5668=EDGE_LOOP('',(#23455,#23456,#23457,#23458));
#5669=EDGE_LOOP('',(#23459,#23460,#23461,#23462));
#5670=EDGE_LOOP('',(#23463,#23464,#23465,#23466));
#5671=EDGE_LOOP('',(#23467,#23468,#23469,#23470));
#5672=EDGE_LOOP('',(#23471,#23472,#23473,#23474));
#5673=EDGE_LOOP('',(#23475,#23476,#23477,#23478));
#5674=EDGE_LOOP('',(#23479,#23480,#23481,#23482));
#5675=EDGE_LOOP('',(#23483,#23484,#23485,#23486));
#5676=EDGE_LOOP('',(#23487,#23488,#23489,#23490));
#5677=EDGE_LOOP('',(#23491,#23492,#23493,#23494));
#5678=EDGE_LOOP('',(#23495,#23496,#23497,#23498));
#5679=EDGE_LOOP('',(#23499,#23500,#23501,#23502));
#5680=EDGE_LOOP('',(#23503,#23504,#23505,#23506));
#5681=EDGE_LOOP('',(#23507,#23508,#23509,#23510));
#5682=EDGE_LOOP('',(#23511,#23512,#23513,#23514));
#5683=EDGE_LOOP('',(#23515,#23516,#23517,#23518));
#5684=EDGE_LOOP('',(#23519,#23520,#23521,#23522,#23523,#23524,#23525,#23526,
#23527,#23528,#23529,#23530));
#5685=EDGE_LOOP('',(#23531,#23532,#23533,#23534,#23535,#23536,#23537,#23538));
#5686=EDGE_LOOP('',(#23539,#23540,#23541,#23542));
#5687=EDGE_LOOP('',(#23543,#23544,#23545,#23546));
#5688=EDGE_LOOP('',(#23547,#23548,#23549,#23550));
#5689=EDGE_LOOP('',(#23551,#23552,#23553,#23554));
#5690=EDGE_LOOP('',(#23555,#23556,#23557,#23558));
#5691=EDGE_LOOP('',(#23559,#23560,#23561,#23562));
#5692=EDGE_LOOP('',(#23563,#23564,#23565,#23566));
#5693=EDGE_LOOP('',(#23567,#23568,#23569,#23570));
#5694=EDGE_LOOP('',(#23571,#23572,#23573,#23574));
#5695=EDGE_LOOP('',(#23575,#23576,#23577,#23578,#23579,#23580,#23581,#23582,
#23583));
#5696=EDGE_LOOP('',(#23584,#23585,#23586,#23587,#23588,#23589,#23590,#23591));
#5697=EDGE_LOOP('',(#23592,#23593,#23594,#23595));
#5698=EDGE_LOOP('',(#23596,#23597,#23598,#23599));
#5699=EDGE_LOOP('',(#23600,#23601,#23602,#23603));
#5700=EDGE_LOOP('',(#23604,#23605,#23606,#23607));
#5701=EDGE_LOOP('',(#23608,#23609,#23610,#23611));
#5702=EDGE_LOOP('',(#23612,#23613,#23614,#23615));
#5703=EDGE_LOOP('',(#23616,#23617,#23618,#23619));
#5704=EDGE_LOOP('',(#23620,#23621,#23622,#23623));
#5705=EDGE_LOOP('',(#23624,#23625,#23626,#23627));
#5706=EDGE_LOOP('',(#23628,#23629,#23630,#23631));
#5707=EDGE_LOOP('',(#23632,#23633,#23634,#23635));
#5708=EDGE_LOOP('',(#23636,#23637,#23638,#23639));
#5709=EDGE_LOOP('',(#23640,#23641,#23642,#23643));
#5710=EDGE_LOOP('',(#23644,#23645,#23646,#23647));
#5711=EDGE_LOOP('',(#23648,#23649,#23650,#23651));
#5712=EDGE_LOOP('',(#23652,#23653,#23654,#23655));
#5713=EDGE_LOOP('',(#23656,#23657,#23658,#23659));
#5714=EDGE_LOOP('',(#23660,#23661,#23662,#23663));
#5715=EDGE_LOOP('',(#23664,#23665,#23666,#23667));
#5716=EDGE_LOOP('',(#23668,#23669,#23670,#23671));
#5717=EDGE_LOOP('',(#23672,#23673,#23674,#23675,#23676,#23677,#23678,#23679,
#23680,#23681,#23682,#23683));
#5718=EDGE_LOOP('',(#23684,#23685,#23686,#23687,#23688,#23689,#23690,#23691));
#5719=EDGE_LOOP('',(#23692,#23693,#23694,#23695,#23696,#23697,#23698,#23699));
#5720=EDGE_LOOP('',(#23700,#23701,#23702,#23703));
#5721=EDGE_LOOP('',(#23704,#23705,#23706,#23707));
#5722=EDGE_LOOP('',(#23708,#23709,#23710,#23711));
#5723=EDGE_LOOP('',(#23712,#23713,#23714,#23715));
#5724=EDGE_LOOP('',(#23716,#23717,#23718,#23719));
#5725=EDGE_LOOP('',(#23720,#23721,#23722,#23723));
#5726=EDGE_LOOP('',(#23724,#23725,#23726,#23727));
#5727=EDGE_LOOP('',(#23728,#23729,#23730,#23731));
#5728=EDGE_LOOP('',(#23732,#23733,#23734,#23735));
#5729=EDGE_LOOP('',(#23736,#23737,#23738,#23739));
#5730=EDGE_LOOP('',(#23740,#23741,#23742,#23743));
#5731=EDGE_LOOP('',(#23744,#23745,#23746,#23747));
#5732=EDGE_LOOP('',(#23748,#23749,#23750,#23751));
#5733=EDGE_LOOP('',(#23752,#23753,#23754,#23755));
#5734=EDGE_LOOP('',(#23756,#23757,#23758,#23759));
#5735=EDGE_LOOP('',(#23760,#23761,#23762,#23763));
#5736=EDGE_LOOP('',(#23764,#23765,#23766,#23767));
#5737=EDGE_LOOP('',(#23768,#23769,#23770,#23771));
#5738=EDGE_LOOP('',(#23772,#23773,#23774,#23775));
#5739=EDGE_LOOP('',(#23776,#23777,#23778,#23779));
#5740=EDGE_LOOP('',(#23780,#23781,#23782,#23783,#23784,#23785,#23786,#23787,
#23788,#23789,#23790,#23791));
#5741=EDGE_LOOP('',(#23792,#23793,#23794,#23795,#23796,#23797,#23798,#23799));
#5742=EDGE_LOOP('',(#23800,#23801,#23802,#23803));
#5743=EDGE_LOOP('',(#23804,#23805,#23806,#23807));
#5744=EDGE_LOOP('',(#23808,#23809,#23810,#23811));
#5745=EDGE_LOOP('',(#23812,#23813,#23814,#23815));
#5746=EDGE_LOOP('',(#23816,#23817,#23818,#23819));
#5747=EDGE_LOOP('',(#23820,#23821,#23822,#23823));
#5748=EDGE_LOOP('',(#23824,#23825,#23826,#23827));
#5749=EDGE_LOOP('',(#23828,#23829,#23830,#23831));
#5750=EDGE_LOOP('',(#23832,#23833,#23834,#23835));
#5751=EDGE_LOOP('',(#23836,#23837,#23838,#23839,#23840,#23841,#23842,#23843,
#23844));
#5752=EDGE_LOOP('',(#23845,#23846,#23847,#23848,#23849,#23850,#23851,#23852));
#5753=EDGE_LOOP('',(#23853,#23854,#23855,#23856));
#5754=EDGE_LOOP('',(#23857,#23858,#23859,#23860));
#5755=EDGE_LOOP('',(#23861,#23862,#23863,#23864));
#5756=EDGE_LOOP('',(#23865,#23866,#23867,#23868));
#5757=EDGE_LOOP('',(#23869,#23870,#23871,#23872));
#5758=EDGE_LOOP('',(#23873,#23874,#23875,#23876));
#5759=EDGE_LOOP('',(#23877,#23878,#23879,#23880));
#5760=EDGE_LOOP('',(#23881,#23882,#23883,#23884));
#5761=EDGE_LOOP('',(#23885,#23886,#23887,#23888));
#5762=EDGE_LOOP('',(#23889,#23890,#23891,#23892));
#5763=EDGE_LOOP('',(#23893,#23894,#23895,#23896));
#5764=EDGE_LOOP('',(#23897,#23898,#23899,#23900));
#5765=EDGE_LOOP('',(#23901,#23902,#23903,#23904));
#5766=EDGE_LOOP('',(#23905,#23906,#23907,#23908));
#5767=EDGE_LOOP('',(#23909,#23910,#23911,#23912));
#5768=EDGE_LOOP('',(#23913,#23914,#23915,#23916));
#5769=EDGE_LOOP('',(#23917,#23918,#23919,#23920));
#5770=EDGE_LOOP('',(#23921,#23922,#23923,#23924));
#5771=EDGE_LOOP('',(#23925,#23926,#23927,#23928));
#5772=EDGE_LOOP('',(#23929,#23930,#23931,#23932));
#5773=EDGE_LOOP('',(#23933,#23934,#23935,#23936,#23937,#23938,#23939,#23940,
#23941,#23942,#23943,#23944));
#5774=EDGE_LOOP('',(#23945,#23946,#23947,#23948,#23949,#23950,#23951,#23952));
#5775=EDGE_LOOP('',(#23953,#23954,#23955,#23956));
#5776=EDGE_LOOP('',(#23957,#23958,#23959,#23960));
#5777=EDGE_LOOP('',(#23961,#23962,#23963,#23964));
#5778=EDGE_LOOP('',(#23965,#23966,#23967,#23968));
#5779=EDGE_LOOP('',(#23969,#23970,#23971,#23972));
#5780=EDGE_LOOP('',(#23973,#23974,#23975,#23976));
#5781=EDGE_LOOP('',(#23977,#23978,#23979,#23980));
#5782=EDGE_LOOP('',(#23981,#23982,#23983,#23984));
#5783=EDGE_LOOP('',(#23985,#23986,#23987,#23988));
#5784=EDGE_LOOP('',(#23989,#23990,#23991,#23992));
#5785=EDGE_LOOP('',(#23993,#23994,#23995,#23996));
#5786=EDGE_LOOP('',(#23997,#23998,#23999,#24000));
#5787=EDGE_LOOP('',(#24001,#24002,#24003,#24004));
#5788=EDGE_LOOP('',(#24005,#24006,#24007,#24008));
#5789=EDGE_LOOP('',(#24009,#24010,#24011,#24012));
#5790=EDGE_LOOP('',(#24013,#24014,#24015,#24016));
#5791=EDGE_LOOP('',(#24017,#24018,#24019,#24020));
#5792=EDGE_LOOP('',(#24021,#24022,#24023,#24024));
#5793=EDGE_LOOP('',(#24025,#24026,#24027,#24028));
#5794=EDGE_LOOP('',(#24029,#24030,#24031,#24032));
#5795=EDGE_LOOP('',(#24033,#24034,#24035,#24036));
#5796=EDGE_LOOP('',(#24037,#24038,#24039,#24040));
#5797=EDGE_LOOP('',(#24041,#24042,#24043,#24044,#24045,#24046,#24047,#24048,
#24049,#24050,#24051,#24052,#24053,#24054,#24055,#24056,#24057,#24058,#24059,
#24060,#24061,#24062));
#5798=EDGE_LOOP('',(#24063,#24064,#24065,#24066,#24067,#24068,#24069,#24070));
#5799=EDGE_LOOP('',(#24071,#24072,#24073,#24074));
#5800=EDGE_LOOP('',(#24075,#24076,#24077,#24078));
#5801=EDGE_LOOP('',(#24079,#24080,#24081,#24082));
#5802=EDGE_LOOP('',(#24083,#24084,#24085,#24086));
#5803=EDGE_LOOP('',(#24087,#24088,#24089,#24090));
#5804=EDGE_LOOP('',(#24091,#24092,#24093,#24094));
#5805=EDGE_LOOP('',(#24095,#24096,#24097,#24098));
#5806=EDGE_LOOP('',(#24099,#24100,#24101,#24102));
#5807=EDGE_LOOP('',(#24103,#24104,#24105,#24106));
#5808=EDGE_LOOP('',(#24107,#24108,#24109,#24110));
#5809=EDGE_LOOP('',(#24111,#24112,#24113,#24114));
#5810=EDGE_LOOP('',(#24115,#24116,#24117,#24118));
#5811=EDGE_LOOP('',(#24119,#24120,#24121,#24122));
#5812=EDGE_LOOP('',(#24123,#24124,#24125,#24126));
#5813=EDGE_LOOP('',(#24127,#24128,#24129,#24130));
#5814=EDGE_LOOP('',(#24131,#24132,#24133,#24134));
#5815=EDGE_LOOP('',(#24135,#24136,#24137,#24138));
#5816=EDGE_LOOP('',(#24139,#24140,#24141,#24142));
#5817=EDGE_LOOP('',(#24143,#24144,#24145,#24146));
#5818=EDGE_LOOP('',(#24147,#24148,#24149,#24150));
#5819=EDGE_LOOP('',(#24151,#24152,#24153,#24154,#24155,#24156,#24157,#24158,
#24159,#24160,#24161,#24162));
#5820=EDGE_LOOP('',(#24163,#24164,#24165,#24166,#24167,#24168,#24169,#24170));
#5821=EDGE_LOOP('',(#24171,#24172,#24173,#24174));
#5822=EDGE_LOOP('',(#24175,#24176,#24177,#24178));
#5823=EDGE_LOOP('',(#24179,#24180,#24181,#24182));
#5824=EDGE_LOOP('',(#24183,#24184,#24185,#24186));
#5825=EDGE_LOOP('',(#24187,#24188,#24189,#24190));
#5826=EDGE_LOOP('',(#24191,#24192,#24193,#24194));
#5827=EDGE_LOOP('',(#24195,#24196,#24197,#24198));
#5828=EDGE_LOOP('',(#24199,#24200,#24201,#24202));
#5829=EDGE_LOOP('',(#24203,#24204,#24205,#24206));
#5830=EDGE_LOOP('',(#24207,#24208,#24209,#24210));
#5831=EDGE_LOOP('',(#24211,#24212,#24213,#24214));
#5832=EDGE_LOOP('',(#24215,#24216,#24217,#24218));
#5833=EDGE_LOOP('',(#24219,#24220,#24221,#24222));
#5834=EDGE_LOOP('',(#24223,#24224,#24225,#24226));
#5835=EDGE_LOOP('',(#24227,#24228,#24229,#24230));
#5836=EDGE_LOOP('',(#24231,#24232,#24233,#24234));
#5837=EDGE_LOOP('',(#24235,#24236,#24237,#24238));
#5838=EDGE_LOOP('',(#24239,#24240,#24241,#24242));
#5839=EDGE_LOOP('',(#24243,#24244,#24245,#24246));
#5840=EDGE_LOOP('',(#24247,#24248,#24249,#24250));
#5841=EDGE_LOOP('',(#24251,#24252,#24253,#24254));
#5842=EDGE_LOOP('',(#24255,#24256,#24257,#24258));
#5843=EDGE_LOOP('',(#24259,#24260,#24261,#24262));
#5844=EDGE_LOOP('',(#24263,#24264,#24265,#24266));
#5845=EDGE_LOOP('',(#24267,#24268,#24269,#24270));
#5846=EDGE_LOOP('',(#24271,#24272,#24273,#24274));
#5847=EDGE_LOOP('',(#24275,#24276,#24277,#24278));
#5848=EDGE_LOOP('',(#24279,#24280,#24281,#24282));
#5849=EDGE_LOOP('',(#24283,#24284,#24285,#24286));
#5850=EDGE_LOOP('',(#24287,#24288,#24289,#24290));
#5851=EDGE_LOOP('',(#24291,#24292,#24293,#24294,#24295,#24296,#24297,#24298,
#24299,#24300,#24301,#24302,#24303,#24304,#24305,#24306,#24307,#24308,#24309,
#24310,#24311,#24312,#24313,#24314,#24315,#24316,#24317,#24318,#24319,#24320));
#5852=EDGE_LOOP('',(#24321,#24322,#24323,#24324,#24325,#24326,#24327,#24328));
#5853=EDGE_LOOP('',(#24329,#24330,#24331,#24332));
#5854=EDGE_LOOP('',(#24333,#24334,#24335,#24336));
#5855=EDGE_LOOP('',(#24337,#24338,#24339,#24340));
#5856=EDGE_LOOP('',(#24341,#24342,#24343,#24344));
#5857=EDGE_LOOP('',(#24345,#24346,#24347,#24348));
#5858=EDGE_LOOP('',(#24349,#24350,#24351,#24352));
#5859=EDGE_LOOP('',(#24353,#24354,#24355,#24356));
#5860=EDGE_LOOP('',(#24357,#24358,#24359,#24360));
#5861=EDGE_LOOP('',(#24361,#24362,#24363,#24364));
#5862=EDGE_LOOP('',(#24365,#24366,#24367,#24368));
#5863=EDGE_LOOP('',(#24369,#24370,#24371,#24372));
#5864=EDGE_LOOP('',(#24373,#24374,#24375,#24376));
#5865=EDGE_LOOP('',(#24377,#24378,#24379,#24380));
#5866=EDGE_LOOP('',(#24381,#24382,#24383,#24384));
#5867=EDGE_LOOP('',(#24385,#24386,#24387,#24388));
#5868=EDGE_LOOP('',(#24389,#24390,#24391,#24392));
#5869=EDGE_LOOP('',(#24393,#24394,#24395,#24396));
#5870=EDGE_LOOP('',(#24397,#24398,#24399,#24400));
#5871=EDGE_LOOP('',(#24401,#24402,#24403,#24404));
#5872=EDGE_LOOP('',(#24405,#24406,#24407,#24408));
#5873=EDGE_LOOP('',(#24409,#24410,#24411,#24412,#24413,#24414,#24415,#24416,
#24417,#24418,#24419,#24420));
#5874=EDGE_LOOP('',(#24421,#24422,#24423,#24424,#24425,#24426,#24427,#24428));
#5875=EDGE_LOOP('',(#24429,#24430,#24431,#24432));
#5876=EDGE_LOOP('',(#24433,#24434,#24435,#24436));
#5877=EDGE_LOOP('',(#24437,#24438,#24439,#24440));
#5878=EDGE_LOOP('',(#24441,#24442,#24443,#24444));
#5879=EDGE_LOOP('',(#24445,#24446,#24447,#24448));
#5880=EDGE_LOOP('',(#24449,#24450,#24451,#24452));
#5881=EDGE_LOOP('',(#24453,#24454,#24455,#24456));
#5882=EDGE_LOOP('',(#24457,#24458,#24459,#24460));
#5883=EDGE_LOOP('',(#24461,#24462,#24463,#24464));
#5884=EDGE_LOOP('',(#24465,#24466,#24467,#24468));
#5885=EDGE_LOOP('',(#24469,#24470,#24471,#24472));
#5886=EDGE_LOOP('',(#24473,#24474,#24475,#24476));
#5887=EDGE_LOOP('',(#24477,#24478,#24479,#24480));
#5888=EDGE_LOOP('',(#24481,#24482,#24483,#24484));
#5889=EDGE_LOOP('',(#24485,#24486,#24487,#24488,#24489,#24490,#24491,#24492,
#24493,#24494,#24495));
#5890=EDGE_LOOP('',(#24496,#24497,#24498));
#5891=EDGE_LOOP('',(#24499,#24500,#24501));
#5892=EDGE_LOOP('',(#24502,#24503,#24504,#24505,#24506,#24507,#24508,#24509));
#5893=EDGE_LOOP('',(#24510,#24511,#24512,#24513));
#5894=EDGE_LOOP('',(#24514,#24515,#24516,#24517));
#5895=EDGE_LOOP('',(#24518,#24519,#24520,#24521));
#5896=EDGE_LOOP('',(#24522,#24523,#24524,#24525));
#5897=EDGE_LOOP('',(#24526,#24527,#24528,#24529));
#5898=EDGE_LOOP('',(#24530,#24531,#24532,#24533));
#5899=EDGE_LOOP('',(#24534,#24535,#24536,#24537));
#5900=EDGE_LOOP('',(#24538,#24539,#24540,#24541));
#5901=EDGE_LOOP('',(#24542,#24543,#24544,#24545));
#5902=EDGE_LOOP('',(#24546,#24547,#24548,#24549));
#5903=EDGE_LOOP('',(#24550,#24551,#24552,#24553));
#5904=EDGE_LOOP('',(#24554,#24555,#24556,#24557));
#5905=EDGE_LOOP('',(#24558,#24559,#24560,#24561));
#5906=EDGE_LOOP('',(#24562,#24563,#24564,#24565));
#5907=EDGE_LOOP('',(#24566,#24567,#24568,#24569));
#5908=EDGE_LOOP('',(#24570,#24571,#24572,#24573));
#5909=EDGE_LOOP('',(#24574,#24575,#24576,#24577));
#5910=EDGE_LOOP('',(#24578,#24579,#24580,#24581));
#5911=EDGE_LOOP('',(#24582,#24583,#24584,#24585));
#5912=EDGE_LOOP('',(#24586,#24587,#24588,#24589));
#5913=EDGE_LOOP('',(#24590,#24591,#24592,#24593));
#5914=EDGE_LOOP('',(#24594,#24595,#24596,#24597));
#5915=EDGE_LOOP('',(#24598,#24599,#24600,#24601));
#5916=EDGE_LOOP('',(#24602,#24603,#24604,#24605));
#5917=EDGE_LOOP('',(#24606,#24607,#24608,#24609));
#5918=EDGE_LOOP('',(#24610,#24611,#24612,#24613));
#5919=EDGE_LOOP('',(#24614,#24615,#24616,#24617));
#5920=EDGE_LOOP('',(#24618,#24619,#24620,#24621));
#5921=EDGE_LOOP('',(#24622,#24623,#24624,#24625));
#5922=EDGE_LOOP('',(#24626,#24627,#24628,#24629));
#5923=EDGE_LOOP('',(#24630,#24631,#24632,#24633));
#5924=EDGE_LOOP('',(#24634,#24635,#24636,#24637));
#5925=EDGE_LOOP('',(#24638,#24639,#24640,#24641));
#5926=EDGE_LOOP('',(#24642,#24643,#24644,#24645));
#5927=EDGE_LOOP('',(#24646,#24647,#24648,#24649));
#5928=EDGE_LOOP('',(#24650,#24651,#24652,#24653));
#5929=EDGE_LOOP('',(#24654,#24655,#24656,#24657));
#5930=EDGE_LOOP('',(#24658,#24659,#24660,#24661));
#5931=EDGE_LOOP('',(#24662,#24663,#24664,#24665));
#5932=EDGE_LOOP('',(#24666,#24667,#24668,#24669));
#5933=EDGE_LOOP('',(#24670,#24671,#24672,#24673));
#5934=EDGE_LOOP('',(#24674,#24675,#24676,#24677));
#5935=EDGE_LOOP('',(#24678,#24679,#24680,#24681));
#5936=EDGE_LOOP('',(#24682,#24683,#24684,#24685));
#5937=EDGE_LOOP('',(#24686,#24687,#24688,#24689));
#5938=EDGE_LOOP('',(#24690,#24691,#24692,#24693));
#5939=EDGE_LOOP('',(#24694,#24695,#24696,#24697));
#5940=EDGE_LOOP('',(#24698,#24699,#24700,#24701));
#5941=EDGE_LOOP('',(#24702,#24703,#24704,#24705));
#5942=EDGE_LOOP('',(#24706,#24707,#24708,#24709));
#5943=EDGE_LOOP('',(#24710,#24711,#24712,#24713));
#5944=EDGE_LOOP('',(#24714,#24715,#24716,#24717));
#5945=EDGE_LOOP('',(#24718,#24719,#24720,#24721));
#5946=EDGE_LOOP('',(#24722,#24723,#24724,#24725));
#5947=EDGE_LOOP('',(#24726,#24727,#24728,#24729));
#5948=EDGE_LOOP('',(#24730,#24731,#24732,#24733));
#5949=EDGE_LOOP('',(#24734,#24735,#24736,#24737));
#5950=EDGE_LOOP('',(#24738,#24739,#24740,#24741));
#5951=EDGE_LOOP('',(#24742,#24743,#24744,#24745));
#5952=EDGE_LOOP('',(#24746,#24747,#24748,#24749));
#5953=EDGE_LOOP('',(#24750,#24751,#24752,#24753));
#5954=EDGE_LOOP('',(#24754,#24755,#24756,#24757));
#5955=EDGE_LOOP('',(#24758,#24759,#24760,#24761));
#5956=EDGE_LOOP('',(#24762,#24763,#24764,#24765));
#5957=EDGE_LOOP('',(#24766,#24767,#24768,#24769));
#5958=EDGE_LOOP('',(#24770,#24771,#24772,#24773));
#5959=EDGE_LOOP('',(#24774,#24775,#24776,#24777));
#5960=EDGE_LOOP('',(#24778,#24779,#24780,#24781));
#5961=EDGE_LOOP('',(#24782,#24783,#24784,#24785));
#5962=EDGE_LOOP('',(#24786,#24787,#24788,#24789));
#5963=EDGE_LOOP('',(#24790,#24791,#24792,#24793));
#5964=EDGE_LOOP('',(#24794,#24795,#24796,#24797));
#5965=EDGE_LOOP('',(#24798,#24799,#24800,#24801));
#5966=EDGE_LOOP('',(#24802,#24803,#24804,#24805));
#5967=EDGE_LOOP('',(#24806,#24807,#24808,#24809));
#5968=EDGE_LOOP('',(#24810,#24811,#24812,#24813));
#5969=EDGE_LOOP('',(#24814,#24815,#24816,#24817));
#5970=EDGE_LOOP('',(#24818,#24819,#24820,#24821));
#5971=EDGE_LOOP('',(#24822,#24823,#24824,#24825));
#5972=EDGE_LOOP('',(#24826,#24827,#24828,#24829));
#5973=EDGE_LOOP('',(#24830,#24831,#24832,#24833));
#5974=EDGE_LOOP('',(#24834,#24835,#24836,#24837));
#5975=EDGE_LOOP('',(#24838,#24839,#24840,#24841));
#5976=EDGE_LOOP('',(#24842,#24843,#24844,#24845));
#5977=EDGE_LOOP('',(#24846,#24847,#24848,#24849));
#5978=EDGE_LOOP('',(#24850,#24851,#24852,#24853));
#5979=EDGE_LOOP('',(#24854,#24855,#24856,#24857));
#5980=EDGE_LOOP('',(#24858,#24859,#24860,#24861));
#5981=EDGE_LOOP('',(#24862,#24863,#24864,#24865));
#5982=EDGE_LOOP('',(#24866,#24867,#24868,#24869));
#5983=EDGE_LOOP('',(#24870,#24871,#24872,#24873));
#5984=EDGE_LOOP('',(#24874,#24875,#24876,#24877));
#5985=EDGE_LOOP('',(#24878,#24879,#24880,#24881));
#5986=EDGE_LOOP('',(#24882,#24883,#24884,#24885));
#5987=EDGE_LOOP('',(#24886,#24887,#24888,#24889));
#5988=EDGE_LOOP('',(#24890,#24891,#24892,#24893));
#5989=EDGE_LOOP('',(#24894,#24895,#24896,#24897));
#5990=EDGE_LOOP('',(#24898,#24899,#24900,#24901));
#5991=EDGE_LOOP('',(#24902,#24903,#24904,#24905));
#5992=EDGE_LOOP('',(#24906,#24907,#24908,#24909));
#5993=EDGE_LOOP('',(#24910,#24911,#24912,#24913));
#5994=EDGE_LOOP('',(#24914,#24915,#24916,#24917));
#5995=EDGE_LOOP('',(#24918,#24919,#24920,#24921));
#5996=EDGE_LOOP('',(#24922,#24923,#24924,#24925));
#5997=EDGE_LOOP('',(#24926,#24927,#24928,#24929));
#5998=EDGE_LOOP('',(#24930,#24931,#24932,#24933));
#5999=EDGE_LOOP('',(#24934,#24935,#24936,#24937));
#6000=EDGE_LOOP('',(#24938,#24939,#24940,#24941));
#6001=EDGE_LOOP('',(#24942,#24943,#24944,#24945));
#6002=EDGE_LOOP('',(#24946,#24947,#24948,#24949));
#6003=EDGE_LOOP('',(#24950,#24951,#24952,#24953));
#6004=EDGE_LOOP('',(#24954,#24955,#24956,#24957));
#6005=EDGE_LOOP('',(#24958,#24959,#24960,#24961));
#6006=EDGE_LOOP('',(#24962,#24963,#24964,#24965));
#6007=EDGE_LOOP('',(#24966,#24967,#24968,#24969));
#6008=EDGE_LOOP('',(#24970,#24971,#24972,#24973));
#6009=EDGE_LOOP('',(#24974,#24975,#24976,#24977));
#6010=EDGE_LOOP('',(#24978,#24979,#24980,#24981));
#6011=EDGE_LOOP('',(#24982,#24983,#24984,#24985));
#6012=EDGE_LOOP('',(#24986,#24987,#24988,#24989));
#6013=EDGE_LOOP('',(#24990,#24991,#24992,#24993));
#6014=EDGE_LOOP('',(#24994,#24995,#24996,#24997));
#6015=EDGE_LOOP('',(#24998,#24999,#25000,#25001));
#6016=EDGE_LOOP('',(#25002,#25003,#25004,#25005));
#6017=EDGE_LOOP('',(#25006,#25007,#25008,#25009));
#6018=EDGE_LOOP('',(#25010,#25011,#25012,#25013));
#6019=EDGE_LOOP('',(#25014,#25015,#25016,#25017));
#6020=EDGE_LOOP('',(#25018,#25019,#25020,#25021));
#6021=EDGE_LOOP('',(#25022,#25023,#25024,#25025));
#6022=EDGE_LOOP('',(#25026,#25027,#25028,#25029));
#6023=EDGE_LOOP('',(#25030,#25031,#25032,#25033));
#6024=EDGE_LOOP('',(#25034,#25035,#25036,#25037));
#6025=EDGE_LOOP('',(#25038,#25039,#25040,#25041));
#6026=EDGE_LOOP('',(#25042,#25043,#25044,#25045));
#6027=EDGE_LOOP('',(#25046,#25047,#25048,#25049));
#6028=EDGE_LOOP('',(#25050,#25051,#25052,#25053));
#6029=EDGE_LOOP('',(#25054,#25055,#25056,#25057));
#6030=EDGE_LOOP('',(#25058,#25059,#25060,#25061));
#6031=EDGE_LOOP('',(#25062,#25063,#25064,#25065));
#6032=EDGE_LOOP('',(#25066,#25067,#25068,#25069));
#6033=EDGE_LOOP('',(#25070,#25071,#25072,#25073));
#6034=EDGE_LOOP('',(#25074,#25075,#25076,#25077));
#6035=EDGE_LOOP('',(#25078,#25079,#25080,#25081));
#6036=EDGE_LOOP('',(#25082,#25083,#25084,#25085));
#6037=EDGE_LOOP('',(#25086,#25087,#25088,#25089));
#6038=EDGE_LOOP('',(#25090,#25091,#25092,#25093));
#6039=EDGE_LOOP('',(#25094,#25095,#25096,#25097));
#6040=EDGE_LOOP('',(#25098,#25099,#25100,#25101));
#6041=EDGE_LOOP('',(#25102,#25103,#25104,#25105));
#6042=EDGE_LOOP('',(#25106,#25107,#25108,#25109));
#6043=EDGE_LOOP('',(#25110,#25111,#25112,#25113));
#6044=EDGE_LOOP('',(#25114,#25115,#25116,#25117));
#6045=EDGE_LOOP('',(#25118,#25119,#25120,#25121));
#6046=EDGE_LOOP('',(#25122,#25123,#25124,#25125));
#6047=EDGE_LOOP('',(#25126,#25127,#25128,#25129));
#6048=EDGE_LOOP('',(#25130,#25131,#25132,#25133));
#6049=EDGE_LOOP('',(#25134,#25135,#25136,#25137));
#6050=EDGE_LOOP('',(#25138,#25139,#25140,#25141));
#6051=EDGE_LOOP('',(#25142,#25143,#25144,#25145));
#6052=EDGE_LOOP('',(#25146,#25147,#25148,#25149));
#6053=EDGE_LOOP('',(#25150,#25151,#25152,#25153));
#6054=EDGE_LOOP('',(#25154,#25155,#25156,#25157));
#6055=EDGE_LOOP('',(#25158,#25159,#25160,#25161));
#6056=EDGE_LOOP('',(#25162,#25163,#25164,#25165));
#6057=EDGE_LOOP('',(#25166,#25167,#25168,#25169));
#6058=EDGE_LOOP('',(#25170,#25171,#25172,#25173));
#6059=EDGE_LOOP('',(#25174,#25175,#25176,#25177));
#6060=EDGE_LOOP('',(#25178,#25179,#25180,#25181));
#6061=EDGE_LOOP('',(#25182,#25183,#25184,#25185));
#6062=EDGE_LOOP('',(#25186,#25187,#25188,#25189));
#6063=EDGE_LOOP('',(#25190,#25191,#25192,#25193));
#6064=EDGE_LOOP('',(#25194,#25195,#25196,#25197));
#6065=EDGE_LOOP('',(#25198,#25199,#25200,#25201));
#6066=EDGE_LOOP('',(#25202,#25203,#25204,#25205));
#6067=EDGE_LOOP('',(#25206,#25207,#25208,#25209));
#6068=EDGE_LOOP('',(#25210,#25211,#25212,#25213));
#6069=EDGE_LOOP('',(#25214,#25215,#25216,#25217));
#6070=EDGE_LOOP('',(#25218,#25219,#25220,#25221));
#6071=EDGE_LOOP('',(#25222,#25223,#25224,#25225));
#6072=EDGE_LOOP('',(#25226,#25227,#25228,#25229));
#6073=EDGE_LOOP('',(#25230,#25231,#25232,#25233));
#6074=EDGE_LOOP('',(#25234,#25235,#25236,#25237));
#6075=EDGE_LOOP('',(#25238,#25239,#25240,#25241));
#6076=EDGE_LOOP('',(#25242,#25243,#25244,#25245));
#6077=EDGE_LOOP('',(#25246,#25247,#25248,#25249));
#6078=EDGE_LOOP('',(#25250,#25251,#25252,#25253));
#6079=EDGE_LOOP('',(#25254,#25255,#25256,#25257));
#6080=EDGE_LOOP('',(#25258,#25259,#25260,#25261));
#6081=EDGE_LOOP('',(#25262,#25263,#25264,#25265));
#6082=EDGE_LOOP('',(#25266,#25267,#25268,#25269));
#6083=EDGE_LOOP('',(#25270,#25271,#25272,#25273));
#6084=EDGE_LOOP('',(#25274,#25275,#25276,#25277));
#6085=EDGE_LOOP('',(#25278,#25279,#25280,#25281));
#6086=EDGE_LOOP('',(#25282,#25283,#25284,#25285));
#6087=EDGE_LOOP('',(#25286,#25287,#25288,#25289));
#6088=EDGE_LOOP('',(#25290,#25291,#25292,#25293));
#6089=EDGE_LOOP('',(#25294,#25295,#25296,#25297));
#6090=EDGE_LOOP('',(#25298,#25299,#25300,#25301));
#6091=EDGE_LOOP('',(#25302,#25303,#25304,#25305));
#6092=EDGE_LOOP('',(#25306,#25307,#25308,#25309));
#6093=EDGE_LOOP('',(#25310,#25311,#25312,#25313));
#6094=EDGE_LOOP('',(#25314,#25315,#25316,#25317));
#6095=EDGE_LOOP('',(#25318,#25319,#25320,#25321));
#6096=EDGE_LOOP('',(#25322,#25323,#25324,#25325));
#6097=EDGE_LOOP('',(#25326,#25327,#25328,#25329));
#6098=EDGE_LOOP('',(#25330,#25331,#25332,#25333));
#6099=EDGE_LOOP('',(#25334,#25335,#25336,#25337));
#6100=EDGE_LOOP('',(#25338,#25339,#25340,#25341));
#6101=EDGE_LOOP('',(#25342,#25343,#25344,#25345));
#6102=EDGE_LOOP('',(#25346,#25347,#25348,#25349));
#6103=EDGE_LOOP('',(#25350,#25351,#25352,#25353));
#6104=EDGE_LOOP('',(#25354,#25355,#25356,#25357));
#6105=EDGE_LOOP('',(#25358,#25359,#25360,#25361));
#6106=EDGE_LOOP('',(#25362,#25363,#25364,#25365));
#6107=EDGE_LOOP('',(#25366,#25367,#25368,#25369));
#6108=EDGE_LOOP('',(#25370,#25371,#25372,#25373));
#6109=EDGE_LOOP('',(#25374,#25375,#25376,#25377));
#6110=EDGE_LOOP('',(#25378,#25379,#25380,#25381));
#6111=EDGE_LOOP('',(#25382,#25383,#25384,#25385));
#6112=EDGE_LOOP('',(#25386,#25387,#25388,#25389));
#6113=EDGE_LOOP('',(#25390,#25391,#25392,#25393));
#6114=EDGE_LOOP('',(#25394,#25395,#25396,#25397));
#6115=EDGE_LOOP('',(#25398,#25399,#25400,#25401));
#6116=EDGE_LOOP('',(#25402,#25403,#25404,#25405));
#6117=EDGE_LOOP('',(#25406,#25407,#25408,#25409));
#6118=EDGE_LOOP('',(#25410,#25411,#25412,#25413));
#6119=EDGE_LOOP('',(#25414,#25415,#25416,#25417));
#6120=EDGE_LOOP('',(#25418,#25419,#25420,#25421));
#6121=EDGE_LOOP('',(#25422,#25423,#25424,#25425));
#6122=EDGE_LOOP('',(#25426,#25427,#25428,#25429));
#6123=EDGE_LOOP('',(#25430,#25431,#25432,#25433));
#6124=EDGE_LOOP('',(#25434,#25435,#25436,#25437));
#6125=EDGE_LOOP('',(#25438,#25439,#25440,#25441));
#6126=EDGE_LOOP('',(#25442,#25443,#25444,#25445));
#6127=EDGE_LOOP('',(#25446,#25447,#25448,#25449));
#6128=EDGE_LOOP('',(#25450,#25451,#25452,#25453));
#6129=EDGE_LOOP('',(#25454,#25455,#25456,#25457));
#6130=EDGE_LOOP('',(#25458,#25459,#25460,#25461));
#6131=EDGE_LOOP('',(#25462,#25463,#25464,#25465));
#6132=EDGE_LOOP('',(#25466,#25467,#25468,#25469));
#6133=EDGE_LOOP('',(#25470,#25471,#25472,#25473));
#6134=EDGE_LOOP('',(#25474,#25475,#25476,#25477));
#6135=EDGE_LOOP('',(#25478,#25479,#25480,#25481));
#6136=EDGE_LOOP('',(#25482,#25483,#25484,#25485));
#6137=EDGE_LOOP('',(#25486,#25487,#25488,#25489));
#6138=EDGE_LOOP('',(#25490,#25491,#25492,#25493));
#6139=EDGE_LOOP('',(#25494,#25495,#25496,#25497));
#6140=EDGE_LOOP('',(#25498,#25499,#25500,#25501));
#6141=EDGE_LOOP('',(#25502,#25503,#25504,#25505));
#6142=EDGE_LOOP('',(#25506,#25507,#25508,#25509));
#6143=EDGE_LOOP('',(#25510,#25511,#25512,#25513));
#6144=EDGE_LOOP('',(#25514,#25515,#25516,#25517));
#6145=EDGE_LOOP('',(#25518,#25519,#25520,#25521));
#6146=EDGE_LOOP('',(#25522,#25523,#25524,#25525));
#6147=EDGE_LOOP('',(#25526,#25527,#25528,#25529));
#6148=EDGE_LOOP('',(#25530,#25531,#25532,#25533));
#6149=EDGE_LOOP('',(#25534,#25535,#25536,#25537));
#6150=EDGE_LOOP('',(#25538,#25539,#25540,#25541));
#6151=EDGE_LOOP('',(#25542,#25543,#25544,#25545));
#6152=EDGE_LOOP('',(#25546,#25547,#25548,#25549));
#6153=EDGE_LOOP('',(#25550,#25551,#25552,#25553));
#6154=EDGE_LOOP('',(#25554,#25555,#25556,#25557));
#6155=EDGE_LOOP('',(#25558,#25559,#25560,#25561));
#6156=EDGE_LOOP('',(#25562,#25563,#25564,#25565));
#6157=EDGE_LOOP('',(#25566,#25567,#25568,#25569));
#6158=EDGE_LOOP('',(#25570,#25571,#25572,#25573));
#6159=EDGE_LOOP('',(#25574,#25575,#25576,#25577));
#6160=EDGE_LOOP('',(#25578,#25579,#25580,#25581));
#6161=EDGE_LOOP('',(#25582,#25583,#25584,#25585));
#6162=EDGE_LOOP('',(#25586,#25587,#25588,#25589));
#6163=EDGE_LOOP('',(#25590,#25591,#25592,#25593));
#6164=EDGE_LOOP('',(#25594,#25595,#25596,#25597));
#6165=EDGE_LOOP('',(#25598,#25599,#25600,#25601));
#6166=EDGE_LOOP('',(#25602,#25603,#25604,#25605));
#6167=EDGE_LOOP('',(#25606,#25607,#25608,#25609));
#6168=EDGE_LOOP('',(#25610,#25611,#25612,#25613));
#6169=EDGE_LOOP('',(#25614,#25615,#25616,#25617));
#6170=EDGE_LOOP('',(#25618,#25619,#25620,#25621));
#6171=EDGE_LOOP('',(#25622,#25623,#25624,#25625));
#6172=EDGE_LOOP('',(#25626,#25627,#25628,#25629));
#6173=EDGE_LOOP('',(#25630,#25631,#25632,#25633));
#6174=EDGE_LOOP('',(#25634,#25635,#25636,#25637));
#6175=EDGE_LOOP('',(#25638,#25639,#25640,#25641));
#6176=EDGE_LOOP('',(#25642,#25643,#25644,#25645));
#6177=EDGE_LOOP('',(#25646,#25647,#25648,#25649));
#6178=EDGE_LOOP('',(#25650,#25651,#25652,#25653));
#6179=EDGE_LOOP('',(#25654,#25655,#25656,#25657));
#6180=EDGE_LOOP('',(#25658,#25659,#25660,#25661));
#6181=EDGE_LOOP('',(#25662,#25663,#25664,#25665));
#6182=EDGE_LOOP('',(#25666,#25667,#25668,#25669));
#6183=EDGE_LOOP('',(#25670,#25671,#25672,#25673));
#6184=EDGE_LOOP('',(#25674,#25675,#25676,#25677));
#6185=EDGE_LOOP('',(#25678,#25679,#25680,#25681));
#6186=EDGE_LOOP('',(#25682,#25683,#25684,#25685));
#6187=EDGE_LOOP('',(#25686,#25687,#25688,#25689));
#6188=EDGE_LOOP('',(#25690,#25691,#25692,#25693));
#6189=EDGE_LOOP('',(#25694,#25695,#25696,#25697));
#6190=EDGE_LOOP('',(#25698,#25699,#25700,#25701));
#6191=EDGE_LOOP('',(#25702,#25703,#25704,#25705));
#6192=EDGE_LOOP('',(#25706,#25707,#25708,#25709));
#6193=EDGE_LOOP('',(#25710,#25711,#25712,#25713));
#6194=EDGE_LOOP('',(#25714,#25715,#25716,#25717));
#6195=EDGE_LOOP('',(#25718,#25719,#25720,#25721));
#6196=EDGE_LOOP('',(#25722,#25723,#25724,#25725));
#6197=EDGE_LOOP('',(#25726,#25727,#25728,#25729));
#6198=EDGE_LOOP('',(#25730,#25731,#25732,#25733));
#6199=EDGE_LOOP('',(#25734,#25735,#25736,#25737));
#6200=EDGE_LOOP('',(#25738,#25739,#25740,#25741));
#6201=EDGE_LOOP('',(#25742,#25743,#25744,#25745));
#6202=EDGE_LOOP('',(#25746,#25747,#25748,#25749));
#6203=EDGE_LOOP('',(#25750,#25751,#25752,#25753));
#6204=EDGE_LOOP('',(#25754,#25755,#25756,#25757));
#6205=EDGE_LOOP('',(#25758,#25759,#25760,#25761));
#6206=EDGE_LOOP('',(#25762,#25763,#25764,#25765));
#6207=EDGE_LOOP('',(#25766,#25767,#25768,#25769));
#6208=EDGE_LOOP('',(#25770,#25771,#25772,#25773));
#6209=EDGE_LOOP('',(#25774,#25775,#25776,#25777));
#6210=EDGE_LOOP('',(#25778,#25779,#25780,#25781));
#6211=EDGE_LOOP('',(#25782,#25783,#25784,#25785));
#6212=EDGE_LOOP('',(#25786,#25787,#25788,#25789));
#6213=EDGE_LOOP('',(#25790,#25791,#25792,#25793));
#6214=EDGE_LOOP('',(#25794,#25795,#25796,#25797));
#6215=EDGE_LOOP('',(#25798,#25799,#25800,#25801));
#6216=EDGE_LOOP('',(#25802,#25803,#25804,#25805));
#6217=EDGE_LOOP('',(#25806,#25807,#25808,#25809));
#6218=EDGE_LOOP('',(#25810,#25811,#25812,#25813));
#6219=EDGE_LOOP('',(#25814,#25815,#25816,#25817));
#6220=EDGE_LOOP('',(#25818,#25819,#25820,#25821));
#6221=EDGE_LOOP('',(#25822,#25823,#25824,#25825));
#6222=EDGE_LOOP('',(#25826,#25827,#25828,#25829));
#6223=EDGE_LOOP('',(#25830,#25831,#25832,#25833));
#6224=EDGE_LOOP('',(#25834,#25835,#25836,#25837));
#6225=EDGE_LOOP('',(#25838,#25839,#25840,#25841));
#6226=EDGE_LOOP('',(#25842,#25843,#25844,#25845));
#6227=EDGE_LOOP('',(#25846,#25847,#25848,#25849));
#6228=EDGE_LOOP('',(#25850,#25851,#25852,#25853));
#6229=EDGE_LOOP('',(#25854,#25855,#25856,#25857));
#6230=EDGE_LOOP('',(#25858,#25859,#25860,#25861));
#6231=EDGE_LOOP('',(#25862,#25863,#25864,#25865));
#6232=EDGE_LOOP('',(#25866,#25867,#25868,#25869));
#6233=EDGE_LOOP('',(#25870,#25871,#25872,#25873));
#6234=EDGE_LOOP('',(#25874,#25875,#25876,#25877));
#6235=EDGE_LOOP('',(#25878,#25879,#25880,#25881));
#6236=EDGE_LOOP('',(#25882,#25883,#25884,#25885));
#6237=EDGE_LOOP('',(#25886,#25887,#25888,#25889));
#6238=EDGE_LOOP('',(#25890,#25891,#25892,#25893));
#6239=EDGE_LOOP('',(#25894,#25895,#25896,#25897));
#6240=EDGE_LOOP('',(#25898,#25899,#25900,#25901));
#6241=EDGE_LOOP('',(#25902,#25903,#25904,#25905));
#6242=EDGE_LOOP('',(#25906,#25907,#25908,#25909));
#6243=EDGE_LOOP('',(#25910,#25911,#25912,#25913));
#6244=EDGE_LOOP('',(#25914,#25915,#25916,#25917));
#6245=EDGE_LOOP('',(#25918,#25919,#25920,#25921));
#6246=EDGE_LOOP('',(#25922,#25923,#25924,#25925));
#6247=EDGE_LOOP('',(#25926,#25927,#25928,#25929));
#6248=EDGE_LOOP('',(#25930,#25931,#25932,#25933));
#6249=EDGE_LOOP('',(#25934,#25935,#25936,#25937));
#6250=EDGE_LOOP('',(#25938,#25939,#25940,#25941));
#6251=EDGE_LOOP('',(#25942,#25943,#25944,#25945));
#6252=EDGE_LOOP('',(#25946,#25947,#25948,#25949));
#6253=EDGE_LOOP('',(#25950,#25951,#25952,#25953));
#6254=EDGE_LOOP('',(#25954,#25955,#25956,#25957));
#6255=EDGE_LOOP('',(#25958,#25959,#25960,#25961));
#6256=EDGE_LOOP('',(#25962,#25963,#25964,#25965));
#6257=EDGE_LOOP('',(#25966,#25967,#25968,#25969));
#6258=EDGE_LOOP('',(#25970,#25971,#25972,#25973));
#6259=EDGE_LOOP('',(#25974,#25975,#25976,#25977));
#6260=EDGE_LOOP('',(#25978,#25979,#25980,#25981));
#6261=EDGE_LOOP('',(#25982,#25983,#25984,#25985));
#6262=EDGE_LOOP('',(#25986,#25987,#25988,#25989));
#6263=EDGE_LOOP('',(#25990,#25991,#25992,#25993));
#6264=EDGE_LOOP('',(#25994,#25995,#25996,#25997));
#6265=EDGE_LOOP('',(#25998,#25999,#26000,#26001));
#6266=EDGE_LOOP('',(#26002,#26003,#26004,#26005));
#6267=EDGE_LOOP('',(#26006,#26007,#26008,#26009));
#6268=EDGE_LOOP('',(#26010,#26011,#26012,#26013));
#6269=EDGE_LOOP('',(#26014,#26015,#26016,#26017));
#6270=EDGE_LOOP('',(#26018,#26019,#26020,#26021));
#6271=EDGE_LOOP('',(#26022,#26023,#26024,#26025));
#6272=EDGE_LOOP('',(#26026,#26027,#26028,#26029));
#6273=EDGE_LOOP('',(#26030,#26031,#26032,#26033));
#6274=EDGE_LOOP('',(#26034,#26035,#26036,#26037));
#6275=EDGE_LOOP('',(#26038,#26039,#26040,#26041));
#6276=EDGE_LOOP('',(#26042,#26043,#26044,#26045));
#6277=EDGE_LOOP('',(#26046,#26047,#26048,#26049));
#6278=EDGE_LOOP('',(#26050,#26051,#26052,#26053));
#6279=EDGE_LOOP('',(#26054,#26055,#26056,#26057));
#6280=EDGE_LOOP('',(#26058,#26059,#26060,#26061));
#6281=EDGE_LOOP('',(#26062,#26063,#26064,#26065));
#6282=EDGE_LOOP('',(#26066,#26067,#26068,#26069));
#6283=EDGE_LOOP('',(#26070,#26071,#26072,#26073));
#6284=EDGE_LOOP('',(#26074,#26075,#26076,#26077));
#6285=EDGE_LOOP('',(#26078,#26079,#26080,#26081));
#6286=EDGE_LOOP('',(#26082,#26083,#26084,#26085));
#6287=EDGE_LOOP('',(#26086,#26087,#26088,#26089));
#6288=EDGE_LOOP('',(#26090,#26091,#26092,#26093));
#6289=EDGE_LOOP('',(#26094,#26095,#26096,#26097));
#6290=EDGE_LOOP('',(#26098,#26099,#26100,#26101));
#6291=EDGE_LOOP('',(#26102,#26103,#26104,#26105));
#6292=EDGE_LOOP('',(#26106,#26107,#26108,#26109));
#6293=EDGE_LOOP('',(#26110,#26111,#26112,#26113));
#6294=EDGE_LOOP('',(#26114,#26115,#26116,#26117));
#6295=EDGE_LOOP('',(#26118,#26119,#26120,#26121));
#6296=EDGE_LOOP('',(#26122,#26123,#26124,#26125));
#6297=EDGE_LOOP('',(#26126,#26127,#26128,#26129));
#6298=EDGE_LOOP('',(#26130,#26131,#26132,#26133));
#6299=EDGE_LOOP('',(#26134,#26135,#26136,#26137));
#6300=EDGE_LOOP('',(#26138,#26139,#26140,#26141));
#6301=EDGE_LOOP('',(#26142,#26143,#26144,#26145));
#6302=EDGE_LOOP('',(#26146,#26147,#26148,#26149));
#6303=EDGE_LOOP('',(#26150,#26151,#26152,#26153));
#6304=EDGE_LOOP('',(#26154,#26155,#26156,#26157));
#6305=EDGE_LOOP('',(#26158,#26159,#26160,#26161));
#6306=EDGE_LOOP('',(#26162,#26163,#26164,#26165));
#6307=EDGE_LOOP('',(#26166,#26167,#26168,#26169));
#6308=EDGE_LOOP('',(#26170,#26171,#26172,#26173));
#6309=EDGE_LOOP('',(#26174,#26175,#26176,#26177));
#6310=EDGE_LOOP('',(#26178,#26179,#26180,#26181));
#6311=EDGE_LOOP('',(#26182,#26183,#26184,#26185));
#6312=EDGE_LOOP('',(#26186,#26187,#26188,#26189));
#6313=EDGE_LOOP('',(#26190,#26191,#26192,#26193));
#6314=EDGE_LOOP('',(#26194,#26195,#26196,#26197));
#6315=EDGE_LOOP('',(#26198,#26199,#26200,#26201));
#6316=EDGE_LOOP('',(#26202,#26203,#26204,#26205));
#6317=EDGE_LOOP('',(#26206,#26207,#26208,#26209));
#6318=EDGE_LOOP('',(#26210,#26211,#26212,#26213));
#6319=EDGE_LOOP('',(#26214,#26215,#26216,#26217));
#6320=EDGE_LOOP('',(#26218,#26219,#26220,#26221));
#6321=EDGE_LOOP('',(#26222,#26223,#26224,#26225));
#6322=EDGE_LOOP('',(#26226,#26227,#26228,#26229));
#6323=EDGE_LOOP('',(#26230,#26231,#26232,#26233));
#6324=EDGE_LOOP('',(#26234,#26235,#26236,#26237));
#6325=EDGE_LOOP('',(#26238,#26239,#26240,#26241));
#6326=EDGE_LOOP('',(#26242,#26243,#26244,#26245));
#6327=EDGE_LOOP('',(#26246,#26247,#26248,#26249));
#6328=EDGE_LOOP('',(#26250,#26251,#26252,#26253,#26254,#26255,#26256,#26257));
#6329=EDGE_LOOP('',(#26258,#26259,#26260,#26261,#26262,#26263,#26264,#26265,
#26266,#26267,#26268,#26269));
#6330=EDGE_LOOP('',(#26270,#26271,#26272,#26273,#26274,#26275,#26276,#26277,
#26278,#26279,#26280,#26281,#26282,#26283,#26284,#26285,#26286,#26287,#26288,
#26289,#26290,#26291,#26292,#26293,#26294,#26295,#26296,#26297,#26298,#26299));
#6331=EDGE_LOOP('',(#26300,#26301,#26302,#26303,#26304,#26305,#26306,#26307,
#26308,#26309,#26310,#26311));
#6332=EDGE_LOOP('',(#26312,#26313,#26314,#26315,#26316,#26317,#26318,#26319,
#26320));
#6333=EDGE_LOOP('',(#26321,#26322,#26323,#26324,#26325,#26326,#26327,#26328,
#26329,#26330,#26331,#26332));
#6334=EDGE_LOOP('',(#26333,#26334,#26335,#26336,#26337,#26338,#26339,#26340,
#26341));
#6335=EDGE_LOOP('',(#26342,#26343,#26344,#26345,#26346,#26347,#26348,#26349,
#26350,#26351,#26352,#26353));
#6336=EDGE_LOOP('',(#26354,#26355,#26356,#26357,#26358,#26359,#26360,#26361,
#26362,#26363,#26364,#26365,#26366,#26367,#26368,#26369,#26370,#26371,#26372,
#26373,#26374,#26375,#26376,#26377,#26378,#26379,#26380,#26381,#26382,#26383));
#6337=EDGE_LOOP('',(#26384,#26385,#26386,#26387));
#6338=EDGE_LOOP('',(#26388,#26389,#26390,#26391));
#6339=EDGE_LOOP('',(#26392,#26393,#26394,#26395));
#6340=EDGE_LOOP('',(#26396,#26397,#26398,#26399));
#6341=EDGE_LOOP('',(#26400,#26401,#26402,#26403));
#6342=EDGE_LOOP('',(#26404,#26405,#26406,#26407));
#6343=EDGE_LOOP('',(#26408,#26409,#26410,#26411));
#6344=EDGE_LOOP('',(#26412,#26413,#26414,#26415));
#6345=EDGE_LOOP('',(#26416,#26417,#26418,#26419));
#6346=EDGE_LOOP('',(#26420,#26421,#26422,#26423));
#6347=EDGE_LOOP('',(#26424,#26425,#26426,#26427));
#6348=EDGE_LOOP('',(#26428,#26429,#26430,#26431));
#6349=EDGE_LOOP('',(#26432,#26433,#26434,#26435));
#6350=EDGE_LOOP('',(#26436,#26437,#26438,#26439));
#6351=EDGE_LOOP('',(#26440,#26441,#26442,#26443));
#6352=EDGE_LOOP('',(#26444,#26445,#26446,#26447));
#6353=EDGE_LOOP('',(#26448,#26449,#26450,#26451));
#6354=EDGE_LOOP('',(#26452,#26453,#26454,#26455));
#6355=EDGE_LOOP('',(#26456,#26457,#26458,#26459));
#6356=EDGE_LOOP('',(#26460,#26461,#26462,#26463));
#6357=EDGE_LOOP('',(#26464,#26465,#26466,#26467));
#6358=EDGE_LOOP('',(#26468,#26469,#26470,#26471));
#6359=EDGE_LOOP('',(#26472,#26473,#26474,#26475));
#6360=EDGE_LOOP('',(#26476,#26477,#26478,#26479));
#6361=EDGE_LOOP('',(#26480,#26481,#26482,#26483));
#6362=EDGE_LOOP('',(#26484,#26485,#26486,#26487));
#6363=EDGE_LOOP('',(#26488,#26489,#26490,#26491));
#6364=EDGE_LOOP('',(#26492,#26493,#26494,#26495));
#6365=EDGE_LOOP('',(#26496,#26497,#26498,#26499));
#6366=EDGE_LOOP('',(#26500,#26501,#26502,#26503));
#6367=EDGE_LOOP('',(#26504,#26505,#26506,#26507));
#6368=EDGE_LOOP('',(#26508,#26509,#26510,#26511));
#6369=EDGE_LOOP('',(#26512,#26513,#26514,#26515));
#6370=EDGE_LOOP('',(#26516,#26517,#26518,#26519));
#6371=EDGE_LOOP('',(#26520,#26521,#26522,#26523));
#6372=EDGE_LOOP('',(#26524,#26525,#26526,#26527));
#6373=EDGE_LOOP('',(#26528,#26529,#26530,#26531));
#6374=EDGE_LOOP('',(#26532,#26533,#26534,#26535));
#6375=EDGE_LOOP('',(#26536,#26537,#26538,#26539));
#6376=EDGE_LOOP('',(#26540,#26541,#26542,#26543));
#6377=EDGE_LOOP('',(#26544,#26545,#26546,#26547));
#6378=EDGE_LOOP('',(#26548,#26549,#26550,#26551));
#6379=EDGE_LOOP('',(#26552,#26553,#26554,#26555));
#6380=EDGE_LOOP('',(#26556,#26557,#26558,#26559));
#6381=EDGE_LOOP('',(#26560,#26561,#26562,#26563));
#6382=EDGE_LOOP('',(#26564,#26565,#26566,#26567));
#6383=EDGE_LOOP('',(#26568,#26569,#26570,#26571));
#6384=EDGE_LOOP('',(#26572,#26573,#26574,#26575));
#6385=EDGE_LOOP('',(#26576,#26577,#26578,#26579));
#6386=EDGE_LOOP('',(#26580,#26581,#26582,#26583));
#6387=EDGE_LOOP('',(#26584,#26585,#26586,#26587));
#6388=EDGE_LOOP('',(#26588,#26589,#26590,#26591));
#6389=EDGE_LOOP('',(#26592,#26593,#26594,#26595));
#6390=EDGE_LOOP('',(#26596,#26597,#26598,#26599));
#6391=EDGE_LOOP('',(#26600,#26601,#26602,#26603));
#6392=EDGE_LOOP('',(#26604,#26605,#26606,#26607));
#6393=EDGE_LOOP('',(#26608,#26609,#26610,#26611));
#6394=EDGE_LOOP('',(#26612,#26613,#26614,#26615));
#6395=EDGE_LOOP('',(#26616,#26617,#26618,#26619));
#6396=EDGE_LOOP('',(#26620,#26621,#26622,#26623));
#6397=EDGE_LOOP('',(#26624,#26625,#26626,#26627));
#6398=EDGE_LOOP('',(#26628,#26629,#26630,#26631));
#6399=EDGE_LOOP('',(#26632,#26633,#26634,#26635));
#6400=EDGE_LOOP('',(#26636,#26637,#26638,#26639));
#6401=EDGE_LOOP('',(#26640,#26641,#26642,#26643));
#6402=EDGE_LOOP('',(#26644,#26645,#26646,#26647));
#6403=EDGE_LOOP('',(#26648,#26649,#26650,#26651));
#6404=EDGE_LOOP('',(#26652,#26653,#26654,#26655));
#6405=EDGE_LOOP('',(#26656,#26657,#26658,#26659));
#6406=EDGE_LOOP('',(#26660,#26661,#26662,#26663));
#6407=EDGE_LOOP('',(#26664,#26665,#26666,#26667));
#6408=EDGE_LOOP('',(#26668,#26669,#26670,#26671));
#6409=EDGE_LOOP('',(#26672,#26673,#26674,#26675));
#6410=EDGE_LOOP('',(#26676,#26677,#26678,#26679));
#6411=EDGE_LOOP('',(#26680,#26681,#26682,#26683));
#6412=EDGE_LOOP('',(#26684,#26685,#26686,#26687));
#6413=EDGE_LOOP('',(#26688,#26689,#26690,#26691));
#6414=EDGE_LOOP('',(#26692,#26693,#26694,#26695));
#6415=EDGE_LOOP('',(#26696,#26697,#26698,#26699));
#6416=EDGE_LOOP('',(#26700,#26701,#26702,#26703));
#6417=EDGE_LOOP('',(#26704,#26705,#26706,#26707));
#6418=EDGE_LOOP('',(#26708,#26709,#26710,#26711));
#6419=EDGE_LOOP('',(#26712,#26713,#26714,#26715));
#6420=EDGE_LOOP('',(#26716,#26717,#26718,#26719));
#6421=EDGE_LOOP('',(#26720,#26721,#26722,#26723));
#6422=EDGE_LOOP('',(#26724));
#6423=EDGE_LOOP('',(#26725));
#6424=EDGE_LOOP('',(#26726,#26727,#26728,#26729,#26730,#26731,#26732,#26733,
#26734,#26735,#26736));
#6425=EDGE_LOOP('',(#26737,#26738,#26739,#26740,#26741,#26742,#26743,#26744,
#26745,#26746,#26747,#26748));
#6426=EDGE_LOOP('',(#26749,#26750,#26751,#26752,#26753,#26754,#26755,#26756,
#26757,#26758,#26759,#26760,#26761,#26762,#26763,#26764,#26765,#26766,#26767,
#26768,#26769,#26770));
#6427=EDGE_LOOP('',(#26771,#26772,#26773,#26774,#26775,#26776,#26777,#26778,
#26779,#26780,#26781,#26782));
#6428=EDGE_LOOP('',(#26783,#26784,#26785,#26786,#26787,#26788,#26789,#26790,
#26791,#26792,#26793,#26794));
#6429=EDGE_LOOP('',(#26795,#26796,#26797,#26798,#26799,#26800,#26801,#26802,
#26803,#26804,#26805,#26806,#26807,#26808,#26809,#26810,#26811,#26812,#26813,
#26814,#26815,#26816));
#6430=EDGE_LOOP('',(#26817,#26818,#26819,#26820,#26821,#26822,#26823,#26824,
#26825,#26826,#26827,#26828));
#6431=EDGE_LOOP('',(#26829,#26830,#26831,#26832,#26833,#26834,#26835,#26836,
#26837,#26838,#26839));
#6432=EDGE_LOOP('',(#26840,#26841,#26842,#26843,#26844,#26845,#26846,#26847,
#26848,#26849,#26850,#26851));
#6433=EDGE_LOOP('',(#26852,#26853,#26854,#26855,#26856,#26857,#26858,#26859));
#6434=EDGE_LOOP('',(#26860));
#6435=EDGE_LOOP('',(#26861));
#7586=LINE('',#69963,#10423);
#7587=LINE('',#69968,#10424);
#7588=LINE('',#69980,#10425);
#7589=LINE('',#69995,#10426);
#7590=LINE('',#70010,#10427);
#7591=LINE('',#70025,#10428);
#7592=LINE('',#70040,#10429);
#7593=LINE('',#70055,#10430);
#7594=LINE('',#70083,#10431);
#7595=LINE('',#70088,#10432);
#7596=LINE('',#70100,#10433);
#7597=LINE('',#70115,#10434);
#7598=LINE('',#70130,#10435);
#7599=LINE('',#70145,#10436);
#7600=LINE('',#70160,#10437);
#7601=LINE('',#70175,#10438);
#7602=LINE('',#70190,#10439);
#7603=LINE('',#70205,#10440);
#7604=LINE('',#70220,#10441);
#7605=LINE('',#70235,#10442);
#7606=LINE('',#70255,#10443);
#7607=LINE('',#70257,#10444);
#7608=LINE('',#70259,#10445);
#7609=LINE('',#70260,#10446);
#7610=LINE('',#70263,#10447);
#7611=LINE('',#70265,#10448);
#7612=LINE('',#70266,#10449);
#7613=LINE('',#70268,#10450);
#7614=LINE('',#70269,#10451);
#7615=LINE('',#70273,#10452);
#7616=LINE('',#70275,#10453);
#7617=LINE('',#70277,#10454);
#7618=LINE('',#70278,#10455);
#7619=LINE('',#70281,#10456);
#7620=LINE('',#70283,#10457);
#7621=LINE('',#70284,#10458);
#7622=LINE('',#70287,#10459);
#7623=LINE('',#70289,#10460);
#7624=LINE('',#70290,#10461);
#7625=LINE('',#70293,#10462);
#7626=LINE('',#70295,#10463);
#7627=LINE('',#70296,#10464);
#7628=LINE('',#70299,#10465);
#7629=LINE('',#70301,#10466);
#7630=LINE('',#70302,#10467);
#7631=LINE('',#70305,#10468);
#7632=LINE('',#70307,#10469);
#7633=LINE('',#70308,#10470);
#7634=LINE('',#70311,#10471);
#7635=LINE('',#70313,#10472);
#7636=LINE('',#70314,#10473);
#7637=LINE('',#70317,#10474);
#7638=LINE('',#70319,#10475);
#7639=LINE('',#70320,#10476);
#7640=LINE('',#70323,#10477);
#7641=LINE('',#70325,#10478);
#7642=LINE('',#70326,#10479);
#7643=LINE('',#70329,#10480);
#7644=LINE('',#70331,#10481);
#7645=LINE('',#70332,#10482);
#7646=LINE('',#70334,#10483);
#7647=LINE('',#70335,#10484);
#7648=LINE('',#70351,#10485);
#7649=LINE('',#70356,#10486);
#7650=LINE('',#70368,#10487);
#7651=LINE('',#70383,#10488);
#7652=LINE('',#70398,#10489);
#7653=LINE('',#70413,#10490);
#7654=LINE('',#70428,#10491);
#7655=LINE('',#70443,#10492);
#7656=LINE('',#70471,#10493);
#7657=LINE('',#70476,#10494);
#7658=LINE('',#70488,#10495);
#7659=LINE('',#70503,#10496);
#7660=LINE('',#70518,#10497);
#7661=LINE('',#70533,#10498);
#7662=LINE('',#70548,#10499);
#7663=LINE('',#70563,#10500);
#7664=LINE('',#70578,#10501);
#7665=LINE('',#70593,#10502);
#7666=LINE('',#70608,#10503);
#7667=LINE('',#70623,#10504);
#7668=LINE('',#70652,#10505);
#7669=LINE('',#70657,#10506);
#7670=LINE('',#70669,#10507);
#7671=LINE('',#70684,#10508);
#7672=LINE('',#70699,#10509);
#7673=LINE('',#70714,#10510);
#7674=LINE('',#70729,#10511);
#7675=LINE('',#70744,#10512);
#7676=LINE('',#70759,#10513);
#7677=LINE('',#70774,#10514);
#7678=LINE('',#70789,#10515);
#7679=LINE('',#70804,#10516);
#7680=LINE('',#70819,#10517);
#7681=LINE('',#70825,#10518);
#7682=LINE('',#70827,#10519);
#7683=LINE('',#70828,#10520);
#7684=LINE('',#70840,#10521);
#7685=LINE('',#70855,#10522);
#7686=LINE('',#70870,#10523);
#7687=LINE('',#70885,#10524);
#7688=LINE('',#70900,#10525);
#7689=LINE('',#70915,#10526);
#7690=LINE('',#70930,#10527);
#7691=LINE('',#70936,#10528);
#7692=LINE('',#70938,#10529);
#7693=LINE('',#70939,#10530);
#7694=LINE('',#70951,#10531);
#7695=LINE('',#70966,#10532);
#7696=LINE('',#70981,#10533);
#7697=LINE('',#70996,#10534);
#7698=LINE('',#71011,#10535);
#7699=LINE('',#71026,#10536);
#7700=LINE('',#71041,#10537);
#7701=LINE('',#71047,#10538);
#7702=LINE('',#71049,#10539);
#7703=LINE('',#71050,#10540);
#7704=LINE('',#71077,#10541);
#7705=LINE('',#71082,#10542);
#7706=LINE('',#71094,#10543);
#7707=LINE('',#71109,#10544);
#7708=LINE('',#71124,#10545);
#7709=LINE('',#71139,#10546);
#7710=LINE('',#71154,#10547);
#7711=LINE('',#71169,#10548);
#7712=LINE('',#71197,#10549);
#7713=LINE('',#71202,#10550);
#7714=LINE('',#71214,#10551);
#7715=LINE('',#71229,#10552);
#7716=LINE('',#71244,#10553);
#7717=LINE('',#71259,#10554);
#7718=LINE('',#71274,#10555);
#7719=LINE('',#71289,#10556);
#7720=LINE('',#71304,#10557);
#7721=LINE('',#71319,#10558);
#7722=LINE('',#71334,#10559);
#7723=LINE('',#71349,#10560);
#7724=LINE('',#71378,#10561);
#7725=LINE('',#71383,#10562);
#7726=LINE('',#71395,#10563);
#7727=LINE('',#71410,#10564);
#7728=LINE('',#71425,#10565);
#7729=LINE('',#71440,#10566);
#7730=LINE('',#71455,#10567);
#7731=LINE('',#71470,#10568);
#7732=LINE('',#71485,#10569);
#7733=LINE('',#71500,#10570);
#7734=LINE('',#71506,#10571);
#7735=LINE('',#71508,#10572);
#7736=LINE('',#71509,#10573);
#7737=LINE('',#71521,#10574);
#7738=LINE('',#71536,#10575);
#7739=LINE('',#71551,#10576);
#7740=LINE('',#71566,#10577);
#7741=LINE('',#71581,#10578);
#7742=LINE('',#71596,#10579);
#7743=LINE('',#71611,#10580);
#7744=LINE('',#71626,#10581);
#7745=LINE('',#71641,#10582);
#7746=LINE('',#71647,#10583);
#7747=LINE('',#71649,#10584);
#7748=LINE('',#71650,#10585);
#7749=LINE('',#71653,#10586);
#7750=LINE('',#71655,#10587);
#7751=LINE('',#71656,#10588);
#7752=LINE('',#71658,#10589);
#7753=LINE('',#71659,#10590);
#7754=LINE('',#71674,#10591);
#7755=LINE('',#71679,#10592);
#7756=LINE('',#71691,#10593);
#7757=LINE('',#71706,#10594);
#7758=LINE('',#71721,#10595);
#7759=LINE('',#71736,#10596);
#7760=LINE('',#71751,#10597);
#7761=LINE('',#71766,#10598);
#7762=LINE('',#71794,#10599);
#7763=LINE('',#71799,#10600);
#7764=LINE('',#71811,#10601);
#7765=LINE('',#71826,#10602);
#7766=LINE('',#71841,#10603);
#7767=LINE('',#71856,#10604);
#7768=LINE('',#71871,#10605);
#7769=LINE('',#71886,#10606);
#7770=LINE('',#71901,#10607);
#7771=LINE('',#71916,#10608);
#7772=LINE('',#71931,#10609);
#7773=LINE('',#71946,#10610);
#7774=LINE('',#71966,#10611);
#7775=LINE('',#71968,#10612);
#7776=LINE('',#71970,#10613);
#7777=LINE('',#71971,#10614);
#7778=LINE('',#71983,#10615);
#7779=LINE('',#71998,#10616);
#7780=LINE('',#72004,#10617);
#7781=LINE('',#72006,#10618);
#7782=LINE('',#72007,#10619);
#7783=LINE('',#72019,#10620);
#7784=LINE('',#72034,#10621);
#7785=LINE('',#72040,#10622);
#7786=LINE('',#72042,#10623);
#7787=LINE('',#72043,#10624);
#7788=LINE('',#72046,#10625);
#7789=LINE('',#72048,#10626);
#7790=LINE('',#72049,#10627);
#7791=LINE('',#72051,#10628);
#7792=LINE('',#72052,#10629);
#7793=LINE('',#72067,#10630);
#7794=LINE('',#72072,#10631);
#7795=LINE('',#72084,#10632);
#7796=LINE('',#72099,#10633);
#7797=LINE('',#72114,#10634);
#7798=LINE('',#72129,#10635);
#7799=LINE('',#72144,#10636);
#7800=LINE('',#72159,#10637);
#7801=LINE('',#72187,#10638);
#7802=LINE('',#72192,#10639);
#7803=LINE('',#72204,#10640);
#7804=LINE('',#72219,#10641);
#7805=LINE('',#72234,#10642);
#7806=LINE('',#72249,#10643);
#7807=LINE('',#72264,#10644);
#7808=LINE('',#72279,#10645);
#7809=LINE('',#72294,#10646);
#7810=LINE('',#72309,#10647);
#7811=LINE('',#72324,#10648);
#7812=LINE('',#72339,#10649);
#7813=LINE('',#72369,#10650);
#7814=LINE('',#72374,#10651);
#7815=LINE('',#72386,#10652);
#7816=LINE('',#72401,#10653);
#7817=LINE('',#72416,#10654);
#7818=LINE('',#72431,#10655);
#7819=LINE('',#72446,#10656);
#7820=LINE('',#72461,#10657);
#7821=LINE('',#72489,#10658);
#7822=LINE('',#72494,#10659);
#7823=LINE('',#72506,#10660);
#7824=LINE('',#72521,#10661);
#7825=LINE('',#72536,#10662);
#7826=LINE('',#72551,#10663);
#7827=LINE('',#72566,#10664);
#7828=LINE('',#72581,#10665);
#7829=LINE('',#72596,#10666);
#7830=LINE('',#72611,#10667);
#7831=LINE('',#72626,#10668);
#7832=LINE('',#72641,#10669);
#7833=LINE('',#72661,#10670);
#7834=LINE('',#72663,#10671);
#7835=LINE('',#72665,#10672);
#7836=LINE('',#72666,#10673);
#7837=LINE('',#72678,#10674);
#7838=LINE('',#72693,#10675);
#7839=LINE('',#72699,#10676);
#7840=LINE('',#72701,#10677);
#7841=LINE('',#72702,#10678);
#7842=LINE('',#72714,#10679);
#7843=LINE('',#72729,#10680);
#7844=LINE('',#72735,#10681);
#7845=LINE('',#72737,#10682);
#7846=LINE('',#72738,#10683);
#7847=LINE('',#72741,#10684);
#7848=LINE('',#72743,#10685);
#7849=LINE('',#72744,#10686);
#7850=LINE('',#72746,#10687);
#7851=LINE('',#72747,#10688);
#7852=LINE('',#72762,#10689);
#7853=LINE('',#72767,#10690);
#7854=LINE('',#72779,#10691);
#7855=LINE('',#72794,#10692);
#7856=LINE('',#72809,#10693);
#7857=LINE('',#72824,#10694);
#7858=LINE('',#72839,#10695);
#7859=LINE('',#72854,#10696);
#7860=LINE('',#72882,#10697);
#7861=LINE('',#72887,#10698);
#7862=LINE('',#72899,#10699);
#7863=LINE('',#72914,#10700);
#7864=LINE('',#72929,#10701);
#7865=LINE('',#72944,#10702);
#7866=LINE('',#72959,#10703);
#7867=LINE('',#72974,#10704);
#7868=LINE('',#72989,#10705);
#7869=LINE('',#73004,#10706);
#7870=LINE('',#73019,#10707);
#7871=LINE('',#73034,#10708);
#7872=LINE('',#73063,#10709);
#7873=LINE('',#73068,#10710);
#7874=LINE('',#73080,#10711);
#7875=LINE('',#73095,#10712);
#7876=LINE('',#73110,#10713);
#7877=LINE('',#73125,#10714);
#7878=LINE('',#73140,#10715);
#7879=LINE('',#73155,#10716);
#7880=LINE('',#73170,#10717);
#7881=LINE('',#73185,#10718);
#7882=LINE('',#73191,#10719);
#7883=LINE('',#73193,#10720);
#7884=LINE('',#73194,#10721);
#7885=LINE('',#73206,#10722);
#7886=LINE('',#73221,#10723);
#7887=LINE('',#73236,#10724);
#7888=LINE('',#73251,#10725);
#7889=LINE('',#73266,#10726);
#7890=LINE('',#73281,#10727);
#7891=LINE('',#73296,#10728);
#7892=LINE('',#73311,#10729);
#7893=LINE('',#73326,#10730);
#7894=LINE('',#73332,#10731);
#7895=LINE('',#73334,#10732);
#7896=LINE('',#73335,#10733);
#7897=LINE('',#73338,#10734);
#7898=LINE('',#73340,#10735);
#7899=LINE('',#73341,#10736);
#7900=LINE('',#73343,#10737);
#7901=LINE('',#73344,#10738);
#7902=LINE('',#73359,#10739);
#7903=LINE('',#73364,#10740);
#7904=LINE('',#73376,#10741);
#7905=LINE('',#73391,#10742);
#7906=LINE('',#73406,#10743);
#7907=LINE('',#73421,#10744);
#7908=LINE('',#73436,#10745);
#7909=LINE('',#73451,#10746);
#7910=LINE('',#73479,#10747);
#7911=LINE('',#73484,#10748);
#7912=LINE('',#73496,#10749);
#7913=LINE('',#73511,#10750);
#7914=LINE('',#73526,#10751);
#7915=LINE('',#73541,#10752);
#7916=LINE('',#73556,#10753);
#7917=LINE('',#73571,#10754);
#7918=LINE('',#73586,#10755);
#7919=LINE('',#73601,#10756);
#7920=LINE('',#73616,#10757);
#7921=LINE('',#73631,#10758);
#7922=LINE('',#73660,#10759);
#7923=LINE('',#73665,#10760);
#7924=LINE('',#73677,#10761);
#7925=LINE('',#73692,#10762);
#7926=LINE('',#73707,#10763);
#7927=LINE('',#73722,#10764);
#7928=LINE('',#73737,#10765);
#7929=LINE('',#73752,#10766);
#7930=LINE('',#73767,#10767);
#7931=LINE('',#73782,#10768);
#7932=LINE('',#73797,#10769);
#7933=LINE('',#73812,#10770);
#7934=LINE('',#73827,#10771);
#7935=LINE('',#73833,#10772);
#7936=LINE('',#73835,#10773);
#7937=LINE('',#73836,#10774);
#7938=LINE('',#73848,#10775);
#7939=LINE('',#73863,#10776);
#7940=LINE('',#73878,#10777);
#7941=LINE('',#73893,#10778);
#7942=LINE('',#73908,#10779);
#7943=LINE('',#73923,#10780);
#7944=LINE('',#73938,#10781);
#7945=LINE('',#73944,#10782);
#7946=LINE('',#73946,#10783);
#7947=LINE('',#73947,#10784);
#7948=LINE('',#73959,#10785);
#7949=LINE('',#73974,#10786);
#7950=LINE('',#73989,#10787);
#7951=LINE('',#74004,#10788);
#7952=LINE('',#74019,#10789);
#7953=LINE('',#74034,#10790);
#7954=LINE('',#74049,#10791);
#7955=LINE('',#74055,#10792);
#7956=LINE('',#74057,#10793);
#7957=LINE('',#74058,#10794);
#7958=LINE('',#74085,#10795);
#7959=LINE('',#74090,#10796);
#7960=LINE('',#74102,#10797);
#7961=LINE('',#74117,#10798);
#7962=LINE('',#74132,#10799);
#7963=LINE('',#74147,#10800);
#7964=LINE('',#74162,#10801);
#7965=LINE('',#74177,#10802);
#7966=LINE('',#74205,#10803);
#7967=LINE('',#74210,#10804);
#7968=LINE('',#74222,#10805);
#7969=LINE('',#74237,#10806);
#7970=LINE('',#74252,#10807);
#7971=LINE('',#74267,#10808);
#7972=LINE('',#74282,#10809);
#7973=LINE('',#74297,#10810);
#7974=LINE('',#74312,#10811);
#7975=LINE('',#74327,#10812);
#7976=LINE('',#74342,#10813);
#7977=LINE('',#74357,#10814);
#7978=LINE('',#74377,#10815);
#7979=LINE('',#74379,#10816);
#7980=LINE('',#74381,#10817);
#7981=LINE('',#74382,#10818);
#7982=LINE('',#74385,#10819);
#7983=LINE('',#74387,#10820);
#7984=LINE('',#74388,#10821);
#7985=LINE('',#74390,#10822);
#7986=LINE('',#74391,#10823);
#7987=LINE('',#74395,#10824);
#7988=LINE('',#74397,#10825);
#7989=LINE('',#74399,#10826);
#7990=LINE('',#74400,#10827);
#7991=LINE('',#74403,#10828);
#7992=LINE('',#74405,#10829);
#7993=LINE('',#74406,#10830);
#7994=LINE('',#74409,#10831);
#7995=LINE('',#74411,#10832);
#7996=LINE('',#74412,#10833);
#7997=LINE('',#74415,#10834);
#7998=LINE('',#74417,#10835);
#7999=LINE('',#74418,#10836);
#8000=LINE('',#74421,#10837);
#8001=LINE('',#74423,#10838);
#8002=LINE('',#74424,#10839);
#8003=LINE('',#74427,#10840);
#8004=LINE('',#74429,#10841);
#8005=LINE('',#74430,#10842);
#8006=LINE('',#74433,#10843);
#8007=LINE('',#74435,#10844);
#8008=LINE('',#74436,#10845);
#8009=LINE('',#74439,#10846);
#8010=LINE('',#74441,#10847);
#8011=LINE('',#74442,#10848);
#8012=LINE('',#74445,#10849);
#8013=LINE('',#74447,#10850);
#8014=LINE('',#74448,#10851);
#8015=LINE('',#74451,#10852);
#8016=LINE('',#74453,#10853);
#8017=LINE('',#74454,#10854);
#8018=LINE('',#74456,#10855);
#8019=LINE('',#74457,#10856);
#8020=LINE('',#74464,#10857);
#8021=LINE('',#74466,#10858);
#8022=LINE('',#74468,#10859);
#8023=LINE('',#74469,#10860);
#8024=LINE('',#74472,#10861);
#8025=LINE('',#74474,#10862);
#8026=LINE('',#74475,#10863);
#8027=LINE('',#74478,#10864);
#8028=LINE('',#74480,#10865);
#8029=LINE('',#74481,#10866);
#8030=LINE('',#74483,#10867);
#8031=LINE('',#74484,#10868);
#8032=LINE('',#74489,#10869);
#8033=LINE('',#74491,#10870);
#8034=LINE('',#74493,#10871);
#8035=LINE('',#74494,#10872);
#8036=LINE('',#74497,#10873);
#8037=LINE('',#74499,#10874);
#8038=LINE('',#74500,#10875);
#8039=LINE('',#74503,#10876);
#8040=LINE('',#74505,#10877);
#8041=LINE('',#74506,#10878);
#8042=LINE('',#74508,#10879);
#8043=LINE('',#74509,#10880);
#8044=LINE('',#74514,#10881);
#8045=LINE('',#74516,#10882);
#8046=LINE('',#74518,#10883);
#8047=LINE('',#74519,#10884);
#8048=LINE('',#74522,#10885);
#8049=LINE('',#74524,#10886);
#8050=LINE('',#74525,#10887);
#8051=LINE('',#74528,#10888);
#8052=LINE('',#74530,#10889);
#8053=LINE('',#74531,#10890);
#8054=LINE('',#74533,#10891);
#8055=LINE('',#74534,#10892);
#8056=LINE('',#74539,#10893);
#8057=LINE('',#74541,#10894);
#8058=LINE('',#74543,#10895);
#8059=LINE('',#74544,#10896);
#8060=LINE('',#74547,#10897);
#8061=LINE('',#74549,#10898);
#8062=LINE('',#74550,#10899);
#8063=LINE('',#74553,#10900);
#8064=LINE('',#74555,#10901);
#8065=LINE('',#74556,#10902);
#8066=LINE('',#74558,#10903);
#8067=LINE('',#74559,#10904);
#8068=LINE('',#74564,#10905);
#8069=LINE('',#74566,#10906);
#8070=LINE('',#74568,#10907);
#8071=LINE('',#74569,#10908);
#8072=LINE('',#74572,#10909);
#8073=LINE('',#74574,#10910);
#8074=LINE('',#74575,#10911);
#8075=LINE('',#74578,#10912);
#8076=LINE('',#74580,#10913);
#8077=LINE('',#74581,#10914);
#8078=LINE('',#74583,#10915);
#8079=LINE('',#74584,#10916);
#8080=LINE('',#74589,#10917);
#8081=LINE('',#74591,#10918);
#8082=LINE('',#74593,#10919);
#8083=LINE('',#74594,#10920);
#8084=LINE('',#74597,#10921);
#8085=LINE('',#74599,#10922);
#8086=LINE('',#74600,#10923);
#8087=LINE('',#74603,#10924);
#8088=LINE('',#74605,#10925);
#8089=LINE('',#74606,#10926);
#8090=LINE('',#74608,#10927);
#8091=LINE('',#74609,#10928);
#8092=LINE('',#74614,#10929);
#8093=LINE('',#74616,#10930);
#8094=LINE('',#74618,#10931);
#8095=LINE('',#74619,#10932);
#8096=LINE('',#74622,#10933);
#8097=LINE('',#74624,#10934);
#8098=LINE('',#74625,#10935);
#8099=LINE('',#74628,#10936);
#8100=LINE('',#74630,#10937);
#8101=LINE('',#74631,#10938);
#8102=LINE('',#74633,#10939);
#8103=LINE('',#74634,#10940);
#8104=LINE('',#74639,#10941);
#8105=LINE('',#74641,#10942);
#8106=LINE('',#74643,#10943);
#8107=LINE('',#74644,#10944);
#8108=LINE('',#74647,#10945);
#8109=LINE('',#74649,#10946);
#8110=LINE('',#74650,#10947);
#8111=LINE('',#74653,#10948);
#8112=LINE('',#74655,#10949);
#8113=LINE('',#74656,#10950);
#8114=LINE('',#74658,#10951);
#8115=LINE('',#74659,#10952);
#8116=LINE('',#74664,#10953);
#8117=LINE('',#74666,#10954);
#8118=LINE('',#74668,#10955);
#8119=LINE('',#74669,#10956);
#8120=LINE('',#74672,#10957);
#8121=LINE('',#74674,#10958);
#8122=LINE('',#74675,#10959);
#8123=LINE('',#74678,#10960);
#8124=LINE('',#74680,#10961);
#8125=LINE('',#74681,#10962);
#8126=LINE('',#74683,#10963);
#8127=LINE('',#74684,#10964);
#8128=LINE('',#74689,#10965);
#8129=LINE('',#74691,#10966);
#8130=LINE('',#74693,#10967);
#8131=LINE('',#74694,#10968);
#8132=LINE('',#74697,#10969);
#8133=LINE('',#74699,#10970);
#8134=LINE('',#74700,#10971);
#8135=LINE('',#74703,#10972);
#8136=LINE('',#74705,#10973);
#8137=LINE('',#74706,#10974);
#8138=LINE('',#74708,#10975);
#8139=LINE('',#74709,#10976);
#8140=LINE('',#74714,#10977);
#8141=LINE('',#74716,#10978);
#8142=LINE('',#74718,#10979);
#8143=LINE('',#74719,#10980);
#8144=LINE('',#74722,#10981);
#8145=LINE('',#74724,#10982);
#8146=LINE('',#74725,#10983);
#8147=LINE('',#74728,#10984);
#8148=LINE('',#74730,#10985);
#8149=LINE('',#74731,#10986);
#8150=LINE('',#74733,#10987);
#8151=LINE('',#74734,#10988);
#8152=LINE('',#74739,#10989);
#8153=LINE('',#74741,#10990);
#8154=LINE('',#74743,#10991);
#8155=LINE('',#74744,#10992);
#8156=LINE('',#74747,#10993);
#8157=LINE('',#74749,#10994);
#8158=LINE('',#74750,#10995);
#8159=LINE('',#74753,#10996);
#8160=LINE('',#74755,#10997);
#8161=LINE('',#74756,#10998);
#8162=LINE('',#74758,#10999);
#8163=LINE('',#74759,#11000);
#8164=LINE('',#74764,#11001);
#8165=LINE('',#74766,#11002);
#8166=LINE('',#74768,#11003);
#8167=LINE('',#74769,#11004);
#8168=LINE('',#74772,#11005);
#8169=LINE('',#74774,#11006);
#8170=LINE('',#74775,#11007);
#8171=LINE('',#74778,#11008);
#8172=LINE('',#74780,#11009);
#8173=LINE('',#74781,#11010);
#8174=LINE('',#74783,#11011);
#8175=LINE('',#74784,#11012);
#8176=LINE('',#74789,#11013);
#8177=LINE('',#74791,#11014);
#8178=LINE('',#74793,#11015);
#8179=LINE('',#74794,#11016);
#8180=LINE('',#74797,#11017);
#8181=LINE('',#74799,#11018);
#8182=LINE('',#74800,#11019);
#8183=LINE('',#74803,#11020);
#8184=LINE('',#74805,#11021);
#8185=LINE('',#74806,#11022);
#8186=LINE('',#74808,#11023);
#8187=LINE('',#74809,#11024);
#8188=LINE('',#74814,#11025);
#8189=LINE('',#74816,#11026);
#8190=LINE('',#74818,#11027);
#8191=LINE('',#74819,#11028);
#8192=LINE('',#74822,#11029);
#8193=LINE('',#74824,#11030);
#8194=LINE('',#74825,#11031);
#8195=LINE('',#74828,#11032);
#8196=LINE('',#74830,#11033);
#8197=LINE('',#74831,#11034);
#8198=LINE('',#74833,#11035);
#8199=LINE('',#74834,#11036);
#8200=LINE('',#74839,#11037);
#8201=LINE('',#74841,#11038);
#8202=LINE('',#74843,#11039);
#8203=LINE('',#74844,#11040);
#8204=LINE('',#74847,#11041);
#8205=LINE('',#74849,#11042);
#8206=LINE('',#74850,#11043);
#8207=LINE('',#74853,#11044);
#8208=LINE('',#74855,#11045);
#8209=LINE('',#74856,#11046);
#8210=LINE('',#74858,#11047);
#8211=LINE('',#74859,#11048);
#8212=LINE('',#74864,#11049);
#8213=LINE('',#74866,#11050);
#8214=LINE('',#74868,#11051);
#8215=LINE('',#74869,#11052);
#8216=LINE('',#74872,#11053);
#8217=LINE('',#74874,#11054);
#8218=LINE('',#74875,#11055);
#8219=LINE('',#74878,#11056);
#8220=LINE('',#74880,#11057);
#8221=LINE('',#74881,#11058);
#8222=LINE('',#74883,#11059);
#8223=LINE('',#74884,#11060);
#8224=LINE('',#74889,#11061);
#8225=LINE('',#74891,#11062);
#8226=LINE('',#74893,#11063);
#8227=LINE('',#74894,#11064);
#8228=LINE('',#74897,#11065);
#8229=LINE('',#74899,#11066);
#8230=LINE('',#74900,#11067);
#8231=LINE('',#74903,#11068);
#8232=LINE('',#74905,#11069);
#8233=LINE('',#74906,#11070);
#8234=LINE('',#74908,#11071);
#8235=LINE('',#74909,#11072);
#8236=LINE('',#74914,#11073);
#8237=LINE('',#74916,#11074);
#8238=LINE('',#74918,#11075);
#8239=LINE('',#74919,#11076);
#8240=LINE('',#74922,#11077);
#8241=LINE('',#74924,#11078);
#8242=LINE('',#74925,#11079);
#8243=LINE('',#74928,#11080);
#8244=LINE('',#74930,#11081);
#8245=LINE('',#74931,#11082);
#8246=LINE('',#74933,#11083);
#8247=LINE('',#74934,#11084);
#8248=LINE('',#74939,#11085);
#8249=LINE('',#74941,#11086);
#8250=LINE('',#74943,#11087);
#8251=LINE('',#74944,#11088);
#8252=LINE('',#74947,#11089);
#8253=LINE('',#74949,#11090);
#8254=LINE('',#74950,#11091);
#8255=LINE('',#74953,#11092);
#8256=LINE('',#74955,#11093);
#8257=LINE('',#74956,#11094);
#8258=LINE('',#74958,#11095);
#8259=LINE('',#74959,#11096);
#8260=LINE('',#74964,#11097);
#8261=LINE('',#74966,#11098);
#8262=LINE('',#74968,#11099);
#8263=LINE('',#74969,#11100);
#8264=LINE('',#74972,#11101);
#8265=LINE('',#74974,#11102);
#8266=LINE('',#74975,#11103);
#8267=LINE('',#74978,#11104);
#8268=LINE('',#74980,#11105);
#8269=LINE('',#74981,#11106);
#8270=LINE('',#74983,#11107);
#8271=LINE('',#74984,#11108);
#8272=LINE('',#74989,#11109);
#8273=LINE('',#74991,#11110);
#8274=LINE('',#74993,#11111);
#8275=LINE('',#74994,#11112);
#8276=LINE('',#74997,#11113);
#8277=LINE('',#74999,#11114);
#8278=LINE('',#75000,#11115);
#8279=LINE('',#75003,#11116);
#8280=LINE('',#75005,#11117);
#8281=LINE('',#75006,#11118);
#8282=LINE('',#75008,#11119);
#8283=LINE('',#75009,#11120);
#8284=LINE('',#75014,#11121);
#8285=LINE('',#75016,#11122);
#8286=LINE('',#75018,#11123);
#8287=LINE('',#75019,#11124);
#8288=LINE('',#75022,#11125);
#8289=LINE('',#75024,#11126);
#8290=LINE('',#75025,#11127);
#8291=LINE('',#75028,#11128);
#8292=LINE('',#75030,#11129);
#8293=LINE('',#75031,#11130);
#8294=LINE('',#75033,#11131);
#8295=LINE('',#75034,#11132);
#8296=LINE('',#75039,#11133);
#8297=LINE('',#75041,#11134);
#8298=LINE('',#75043,#11135);
#8299=LINE('',#75044,#11136);
#8300=LINE('',#75047,#11137);
#8301=LINE('',#75049,#11138);
#8302=LINE('',#75050,#11139);
#8303=LINE('',#75053,#11140);
#8304=LINE('',#75055,#11141);
#8305=LINE('',#75056,#11142);
#8306=LINE('',#75058,#11143);
#8307=LINE('',#75059,#11144);
#8308=LINE('',#75064,#11145);
#8309=LINE('',#75066,#11146);
#8310=LINE('',#75068,#11147);
#8311=LINE('',#75069,#11148);
#8312=LINE('',#75072,#11149);
#8313=LINE('',#75074,#11150);
#8314=LINE('',#75075,#11151);
#8315=LINE('',#75078,#11152);
#8316=LINE('',#75080,#11153);
#8317=LINE('',#75081,#11154);
#8318=LINE('',#75083,#11155);
#8319=LINE('',#75084,#11156);
#8320=LINE('',#75089,#11157);
#8321=LINE('',#75091,#11158);
#8322=LINE('',#75093,#11159);
#8323=LINE('',#75094,#11160);
#8324=LINE('',#75097,#11161);
#8325=LINE('',#75099,#11162);
#8326=LINE('',#75100,#11163);
#8327=LINE('',#75103,#11164);
#8328=LINE('',#75105,#11165);
#8329=LINE('',#75106,#11166);
#8330=LINE('',#75108,#11167);
#8331=LINE('',#75109,#11168);
#8332=LINE('',#75114,#11169);
#8333=LINE('',#75116,#11170);
#8334=LINE('',#75118,#11171);
#8335=LINE('',#75119,#11172);
#8336=LINE('',#75122,#11173);
#8337=LINE('',#75124,#11174);
#8338=LINE('',#75125,#11175);
#8339=LINE('',#75128,#11176);
#8340=LINE('',#75130,#11177);
#8341=LINE('',#75131,#11178);
#8342=LINE('',#75133,#11179);
#8343=LINE('',#75134,#11180);
#8344=LINE('',#75139,#11181);
#8345=LINE('',#75141,#11182);
#8346=LINE('',#75143,#11183);
#8347=LINE('',#75144,#11184);
#8348=LINE('',#75147,#11185);
#8349=LINE('',#75149,#11186);
#8350=LINE('',#75150,#11187);
#8351=LINE('',#75153,#11188);
#8352=LINE('',#75155,#11189);
#8353=LINE('',#75156,#11190);
#8354=LINE('',#75158,#11191);
#8355=LINE('',#75159,#11192);
#8356=LINE('',#75164,#11193);
#8357=LINE('',#75166,#11194);
#8358=LINE('',#75168,#11195);
#8359=LINE('',#75169,#11196);
#8360=LINE('',#75172,#11197);
#8361=LINE('',#75174,#11198);
#8362=LINE('',#75175,#11199);
#8363=LINE('',#75178,#11200);
#8364=LINE('',#75180,#11201);
#8365=LINE('',#75181,#11202);
#8366=LINE('',#75183,#11203);
#8367=LINE('',#75184,#11204);
#8368=LINE('',#75189,#11205);
#8369=LINE('',#75191,#11206);
#8370=LINE('',#75193,#11207);
#8371=LINE('',#75194,#11208);
#8372=LINE('',#75197,#11209);
#8373=LINE('',#75199,#11210);
#8374=LINE('',#75200,#11211);
#8375=LINE('',#75203,#11212);
#8376=LINE('',#75205,#11213);
#8377=LINE('',#75206,#11214);
#8378=LINE('',#75208,#11215);
#8379=LINE('',#75209,#11216);
#8380=LINE('',#75214,#11217);
#8381=LINE('',#75216,#11218);
#8382=LINE('',#75218,#11219);
#8383=LINE('',#75219,#11220);
#8384=LINE('',#75222,#11221);
#8385=LINE('',#75224,#11222);
#8386=LINE('',#75225,#11223);
#8387=LINE('',#75228,#11224);
#8388=LINE('',#75230,#11225);
#8389=LINE('',#75231,#11226);
#8390=LINE('',#75233,#11227);
#8391=LINE('',#75234,#11228);
#8392=LINE('',#75239,#11229);
#8393=LINE('',#75241,#11230);
#8394=LINE('',#75243,#11231);
#8395=LINE('',#75244,#11232);
#8396=LINE('',#75247,#11233);
#8397=LINE('',#75249,#11234);
#8398=LINE('',#75250,#11235);
#8399=LINE('',#75253,#11236);
#8400=LINE('',#75255,#11237);
#8401=LINE('',#75256,#11238);
#8402=LINE('',#75258,#11239);
#8403=LINE('',#75259,#11240);
#8404=LINE('',#75264,#11241);
#8405=LINE('',#75266,#11242);
#8406=LINE('',#75268,#11243);
#8407=LINE('',#75269,#11244);
#8408=LINE('',#75272,#11245);
#8409=LINE('',#75274,#11246);
#8410=LINE('',#75275,#11247);
#8411=LINE('',#75278,#11248);
#8412=LINE('',#75280,#11249);
#8413=LINE('',#75281,#11250);
#8414=LINE('',#75283,#11251);
#8415=LINE('',#75284,#11252);
#8416=LINE('',#75289,#11253);
#8417=LINE('',#75291,#11254);
#8418=LINE('',#75293,#11255);
#8419=LINE('',#75294,#11256);
#8420=LINE('',#75297,#11257);
#8421=LINE('',#75299,#11258);
#8422=LINE('',#75300,#11259);
#8423=LINE('',#75303,#11260);
#8424=LINE('',#75305,#11261);
#8425=LINE('',#75306,#11262);
#8426=LINE('',#75308,#11263);
#8427=LINE('',#75309,#11264);
#8428=LINE('',#75314,#11265);
#8429=LINE('',#75316,#11266);
#8430=LINE('',#75318,#11267);
#8431=LINE('',#75319,#11268);
#8432=LINE('',#75322,#11269);
#8433=LINE('',#75324,#11270);
#8434=LINE('',#75325,#11271);
#8435=LINE('',#75328,#11272);
#8436=LINE('',#75330,#11273);
#8437=LINE('',#75331,#11274);
#8438=LINE('',#75333,#11275);
#8439=LINE('',#75334,#11276);
#8440=LINE('',#75339,#11277);
#8441=LINE('',#75341,#11278);
#8442=LINE('',#75343,#11279);
#8443=LINE('',#75344,#11280);
#8444=LINE('',#75347,#11281);
#8445=LINE('',#75349,#11282);
#8446=LINE('',#75350,#11283);
#8447=LINE('',#75353,#11284);
#8448=LINE('',#75355,#11285);
#8449=LINE('',#75356,#11286);
#8450=LINE('',#75358,#11287);
#8451=LINE('',#75359,#11288);
#8452=LINE('',#75364,#11289);
#8453=LINE('',#75366,#11290);
#8454=LINE('',#75368,#11291);
#8455=LINE('',#75369,#11292);
#8456=LINE('',#75372,#11293);
#8457=LINE('',#75374,#11294);
#8458=LINE('',#75375,#11295);
#8459=LINE('',#75378,#11296);
#8460=LINE('',#75380,#11297);
#8461=LINE('',#75381,#11298);
#8462=LINE('',#75383,#11299);
#8463=LINE('',#75384,#11300);
#8464=LINE('',#75389,#11301);
#8465=LINE('',#75391,#11302);
#8466=LINE('',#75393,#11303);
#8467=LINE('',#75394,#11304);
#8468=LINE('',#75397,#11305);
#8469=LINE('',#75399,#11306);
#8470=LINE('',#75400,#11307);
#8471=LINE('',#75403,#11308);
#8472=LINE('',#75405,#11309);
#8473=LINE('',#75406,#11310);
#8474=LINE('',#75408,#11311);
#8475=LINE('',#75409,#11312);
#8476=LINE('',#75414,#11313);
#8477=LINE('',#75416,#11314);
#8478=LINE('',#75418,#11315);
#8479=LINE('',#75419,#11316);
#8480=LINE('',#75422,#11317);
#8481=LINE('',#75424,#11318);
#8482=LINE('',#75425,#11319);
#8483=LINE('',#75428,#11320);
#8484=LINE('',#75430,#11321);
#8485=LINE('',#75431,#11322);
#8486=LINE('',#75433,#11323);
#8487=LINE('',#75434,#11324);
#8488=LINE('',#75439,#11325);
#8489=LINE('',#75441,#11326);
#8490=LINE('',#75443,#11327);
#8491=LINE('',#75444,#11328);
#8492=LINE('',#75447,#11329);
#8493=LINE('',#75449,#11330);
#8494=LINE('',#75450,#11331);
#8495=LINE('',#75453,#11332);
#8496=LINE('',#75455,#11333);
#8497=LINE('',#75456,#11334);
#8498=LINE('',#75458,#11335);
#8499=LINE('',#75459,#11336);
#8500=LINE('',#75464,#11337);
#8501=LINE('',#75466,#11338);
#8502=LINE('',#75468,#11339);
#8503=LINE('',#75469,#11340);
#8504=LINE('',#75472,#11341);
#8505=LINE('',#75474,#11342);
#8506=LINE('',#75475,#11343);
#8507=LINE('',#75478,#11344);
#8508=LINE('',#75480,#11345);
#8509=LINE('',#75481,#11346);
#8510=LINE('',#75483,#11347);
#8511=LINE('',#75484,#11348);
#8512=LINE('',#75489,#11349);
#8513=LINE('',#75491,#11350);
#8514=LINE('',#75493,#11351);
#8515=LINE('',#75494,#11352);
#8516=LINE('',#75497,#11353);
#8517=LINE('',#75499,#11354);
#8518=LINE('',#75500,#11355);
#8519=LINE('',#75503,#11356);
#8520=LINE('',#75505,#11357);
#8521=LINE('',#75506,#11358);
#8522=LINE('',#75508,#11359);
#8523=LINE('',#75509,#11360);
#8524=LINE('',#75514,#11361);
#8525=LINE('',#75516,#11362);
#8526=LINE('',#75518,#11363);
#8527=LINE('',#75519,#11364);
#8528=LINE('',#75522,#11365);
#8529=LINE('',#75524,#11366);
#8530=LINE('',#75525,#11367);
#8531=LINE('',#75528,#11368);
#8532=LINE('',#75530,#11369);
#8533=LINE('',#75531,#11370);
#8534=LINE('',#75533,#11371);
#8535=LINE('',#75534,#11372);
#8536=LINE('',#75539,#11373);
#8537=LINE('',#75541,#11374);
#8538=LINE('',#75543,#11375);
#8539=LINE('',#75544,#11376);
#8540=LINE('',#75547,#11377);
#8541=LINE('',#75549,#11378);
#8542=LINE('',#75550,#11379);
#8543=LINE('',#75553,#11380);
#8544=LINE('',#75555,#11381);
#8545=LINE('',#75556,#11382);
#8546=LINE('',#75558,#11383);
#8547=LINE('',#75559,#11384);
#8548=LINE('',#75564,#11385);
#8549=LINE('',#75566,#11386);
#8550=LINE('',#75568,#11387);
#8551=LINE('',#75569,#11388);
#8552=LINE('',#75572,#11389);
#8553=LINE('',#75574,#11390);
#8554=LINE('',#75575,#11391);
#8555=LINE('',#75578,#11392);
#8556=LINE('',#75580,#11393);
#8557=LINE('',#75581,#11394);
#8558=LINE('',#75583,#11395);
#8559=LINE('',#75584,#11396);
#8560=LINE('',#75589,#11397);
#8561=LINE('',#75591,#11398);
#8562=LINE('',#75593,#11399);
#8563=LINE('',#75594,#11400);
#8564=LINE('',#75597,#11401);
#8565=LINE('',#75599,#11402);
#8566=LINE('',#75600,#11403);
#8567=LINE('',#75603,#11404);
#8568=LINE('',#75605,#11405);
#8569=LINE('',#75606,#11406);
#8570=LINE('',#75608,#11407);
#8571=LINE('',#75609,#11408);
#8572=LINE('',#75614,#11409);
#8573=LINE('',#75616,#11410);
#8574=LINE('',#75618,#11411);
#8575=LINE('',#75619,#11412);
#8576=LINE('',#75622,#11413);
#8577=LINE('',#75624,#11414);
#8578=LINE('',#75625,#11415);
#8579=LINE('',#75628,#11416);
#8580=LINE('',#75630,#11417);
#8581=LINE('',#75631,#11418);
#8582=LINE('',#75633,#11419);
#8583=LINE('',#75634,#11420);
#8584=LINE('',#75639,#11421);
#8585=LINE('',#75641,#11422);
#8586=LINE('',#75643,#11423);
#8587=LINE('',#75644,#11424);
#8588=LINE('',#75647,#11425);
#8589=LINE('',#75649,#11426);
#8590=LINE('',#75650,#11427);
#8591=LINE('',#75653,#11428);
#8592=LINE('',#75655,#11429);
#8593=LINE('',#75656,#11430);
#8594=LINE('',#75658,#11431);
#8595=LINE('',#75659,#11432);
#8596=LINE('',#75664,#11433);
#8597=LINE('',#75666,#11434);
#8598=LINE('',#75668,#11435);
#8599=LINE('',#75669,#11436);
#8600=LINE('',#75672,#11437);
#8601=LINE('',#75674,#11438);
#8602=LINE('',#75675,#11439);
#8603=LINE('',#75678,#11440);
#8604=LINE('',#75680,#11441);
#8605=LINE('',#75681,#11442);
#8606=LINE('',#75683,#11443);
#8607=LINE('',#75684,#11444);
#8608=LINE('',#75689,#11445);
#8609=LINE('',#75691,#11446);
#8610=LINE('',#75693,#11447);
#8611=LINE('',#75694,#11448);
#8612=LINE('',#75697,#11449);
#8613=LINE('',#75699,#11450);
#8614=LINE('',#75700,#11451);
#8615=LINE('',#75703,#11452);
#8616=LINE('',#75705,#11453);
#8617=LINE('',#75706,#11454);
#8618=LINE('',#75708,#11455);
#8619=LINE('',#75709,#11456);
#8620=LINE('',#75714,#11457);
#8621=LINE('',#75716,#11458);
#8622=LINE('',#75718,#11459);
#8623=LINE('',#75719,#11460);
#8624=LINE('',#75722,#11461);
#8625=LINE('',#75724,#11462);
#8626=LINE('',#75725,#11463);
#8627=LINE('',#75728,#11464);
#8628=LINE('',#75730,#11465);
#8629=LINE('',#75731,#11466);
#8630=LINE('',#75733,#11467);
#8631=LINE('',#75734,#11468);
#8632=LINE('',#75739,#11469);
#8633=LINE('',#75741,#11470);
#8634=LINE('',#75743,#11471);
#8635=LINE('',#75744,#11472);
#8636=LINE('',#75747,#11473);
#8637=LINE('',#75749,#11474);
#8638=LINE('',#75750,#11475);
#8639=LINE('',#75753,#11476);
#8640=LINE('',#75755,#11477);
#8641=LINE('',#75756,#11478);
#8642=LINE('',#75758,#11479);
#8643=LINE('',#75759,#11480);
#8644=LINE('',#75764,#11481);
#8645=LINE('',#75766,#11482);
#8646=LINE('',#75768,#11483);
#8647=LINE('',#75769,#11484);
#8648=LINE('',#75772,#11485);
#8649=LINE('',#75774,#11486);
#8650=LINE('',#75775,#11487);
#8651=LINE('',#75778,#11488);
#8652=LINE('',#75780,#11489);
#8653=LINE('',#75781,#11490);
#8654=LINE('',#75783,#11491);
#8655=LINE('',#75784,#11492);
#8656=LINE('',#75789,#11493);
#8657=LINE('',#75791,#11494);
#8658=LINE('',#75793,#11495);
#8659=LINE('',#75794,#11496);
#8660=LINE('',#75797,#11497);
#8661=LINE('',#75799,#11498);
#8662=LINE('',#75800,#11499);
#8663=LINE('',#75803,#11500);
#8664=LINE('',#75805,#11501);
#8665=LINE('',#75806,#11502);
#8666=LINE('',#75808,#11503);
#8667=LINE('',#75809,#11504);
#8668=LINE('',#75814,#11505);
#8669=LINE('',#75816,#11506);
#8670=LINE('',#75818,#11507);
#8671=LINE('',#75819,#11508);
#8672=LINE('',#75822,#11509);
#8673=LINE('',#75824,#11510);
#8674=LINE('',#75825,#11511);
#8675=LINE('',#75828,#11512);
#8676=LINE('',#75830,#11513);
#8677=LINE('',#75831,#11514);
#8678=LINE('',#75833,#11515);
#8679=LINE('',#75834,#11516);
#8680=LINE('',#75839,#11517);
#8681=LINE('',#75841,#11518);
#8682=LINE('',#75843,#11519);
#8683=LINE('',#75844,#11520);
#8684=LINE('',#75847,#11521);
#8685=LINE('',#75849,#11522);
#8686=LINE('',#75850,#11523);
#8687=LINE('',#75853,#11524);
#8688=LINE('',#75855,#11525);
#8689=LINE('',#75856,#11526);
#8690=LINE('',#75858,#11527);
#8691=LINE('',#75859,#11528);
#8692=LINE('',#75864,#11529);
#8693=LINE('',#75866,#11530);
#8694=LINE('',#75868,#11531);
#8695=LINE('',#75869,#11532);
#8696=LINE('',#75872,#11533);
#8697=LINE('',#75874,#11534);
#8698=LINE('',#75875,#11535);
#8699=LINE('',#75878,#11536);
#8700=LINE('',#75880,#11537);
#8701=LINE('',#75881,#11538);
#8702=LINE('',#75883,#11539);
#8703=LINE('',#75884,#11540);
#8704=LINE('',#75889,#11541);
#8705=LINE('',#75891,#11542);
#8706=LINE('',#75893,#11543);
#8707=LINE('',#75894,#11544);
#8708=LINE('',#75897,#11545);
#8709=LINE('',#75899,#11546);
#8710=LINE('',#75900,#11547);
#8711=LINE('',#75903,#11548);
#8712=LINE('',#75905,#11549);
#8713=LINE('',#75906,#11550);
#8714=LINE('',#75908,#11551);
#8715=LINE('',#75909,#11552);
#8716=LINE('',#75914,#11553);
#8717=LINE('',#75916,#11554);
#8718=LINE('',#75918,#11555);
#8719=LINE('',#75919,#11556);
#8720=LINE('',#75922,#11557);
#8721=LINE('',#75924,#11558);
#8722=LINE('',#75925,#11559);
#8723=LINE('',#75928,#11560);
#8724=LINE('',#75930,#11561);
#8725=LINE('',#75931,#11562);
#8726=LINE('',#75933,#11563);
#8727=LINE('',#75934,#11564);
#8728=LINE('',#75939,#11565);
#8729=LINE('',#75941,#11566);
#8730=LINE('',#75943,#11567);
#8731=LINE('',#75944,#11568);
#8732=LINE('',#75947,#11569);
#8733=LINE('',#75949,#11570);
#8734=LINE('',#75950,#11571);
#8735=LINE('',#75953,#11572);
#8736=LINE('',#75955,#11573);
#8737=LINE('',#75956,#11574);
#8738=LINE('',#75958,#11575);
#8739=LINE('',#75959,#11576);
#8740=LINE('',#75964,#11577);
#8741=LINE('',#75966,#11578);
#8742=LINE('',#75968,#11579);
#8743=LINE('',#75969,#11580);
#8744=LINE('',#75972,#11581);
#8745=LINE('',#75974,#11582);
#8746=LINE('',#75975,#11583);
#8747=LINE('',#75978,#11584);
#8748=LINE('',#75980,#11585);
#8749=LINE('',#75981,#11586);
#8750=LINE('',#75983,#11587);
#8751=LINE('',#75984,#11588);
#8752=LINE('',#75989,#11589);
#8753=LINE('',#75991,#11590);
#8754=LINE('',#75993,#11591);
#8755=LINE('',#75994,#11592);
#8756=LINE('',#75997,#11593);
#8757=LINE('',#75999,#11594);
#8758=LINE('',#76000,#11595);
#8759=LINE('',#76003,#11596);
#8760=LINE('',#76005,#11597);
#8761=LINE('',#76006,#11598);
#8762=LINE('',#76008,#11599);
#8763=LINE('',#76009,#11600);
#8764=LINE('',#76014,#11601);
#8765=LINE('',#76016,#11602);
#8766=LINE('',#76018,#11603);
#8767=LINE('',#76019,#11604);
#8768=LINE('',#76022,#11605);
#8769=LINE('',#76024,#11606);
#8770=LINE('',#76025,#11607);
#8771=LINE('',#76028,#11608);
#8772=LINE('',#76030,#11609);
#8773=LINE('',#76031,#11610);
#8774=LINE('',#76033,#11611);
#8775=LINE('',#76034,#11612);
#8776=LINE('',#76039,#11613);
#8777=LINE('',#76041,#11614);
#8778=LINE('',#76043,#11615);
#8779=LINE('',#76044,#11616);
#8780=LINE('',#76047,#11617);
#8781=LINE('',#76049,#11618);
#8782=LINE('',#76050,#11619);
#8783=LINE('',#76053,#11620);
#8784=LINE('',#76055,#11621);
#8785=LINE('',#76056,#11622);
#8786=LINE('',#76058,#11623);
#8787=LINE('',#76059,#11624);
#8788=LINE('',#76064,#11625);
#8789=LINE('',#76066,#11626);
#8790=LINE('',#76068,#11627);
#8791=LINE('',#76069,#11628);
#8792=LINE('',#76072,#11629);
#8793=LINE('',#76074,#11630);
#8794=LINE('',#76075,#11631);
#8795=LINE('',#76078,#11632);
#8796=LINE('',#76080,#11633);
#8797=LINE('',#76081,#11634);
#8798=LINE('',#76083,#11635);
#8799=LINE('',#76084,#11636);
#8800=LINE('',#76089,#11637);
#8801=LINE('',#76091,#11638);
#8802=LINE('',#76093,#11639);
#8803=LINE('',#76094,#11640);
#8804=LINE('',#76097,#11641);
#8805=LINE('',#76099,#11642);
#8806=LINE('',#76100,#11643);
#8807=LINE('',#76103,#11644);
#8808=LINE('',#76105,#11645);
#8809=LINE('',#76106,#11646);
#8810=LINE('',#76108,#11647);
#8811=LINE('',#76109,#11648);
#8812=LINE('',#76114,#11649);
#8813=LINE('',#76116,#11650);
#8814=LINE('',#76118,#11651);
#8815=LINE('',#76119,#11652);
#8816=LINE('',#76122,#11653);
#8817=LINE('',#76124,#11654);
#8818=LINE('',#76125,#11655);
#8819=LINE('',#76128,#11656);
#8820=LINE('',#76130,#11657);
#8821=LINE('',#76131,#11658);
#8822=LINE('',#76133,#11659);
#8823=LINE('',#76134,#11660);
#8824=LINE('',#76139,#11661);
#8825=LINE('',#76141,#11662);
#8826=LINE('',#76143,#11663);
#8827=LINE('',#76144,#11664);
#8828=LINE('',#76147,#11665);
#8829=LINE('',#76149,#11666);
#8830=LINE('',#76150,#11667);
#8831=LINE('',#76153,#11668);
#8832=LINE('',#76155,#11669);
#8833=LINE('',#76156,#11670);
#8834=LINE('',#76158,#11671);
#8835=LINE('',#76159,#11672);
#8836=LINE('',#76164,#11673);
#8837=LINE('',#76166,#11674);
#8838=LINE('',#76168,#11675);
#8839=LINE('',#76169,#11676);
#8840=LINE('',#76172,#11677);
#8841=LINE('',#76174,#11678);
#8842=LINE('',#76175,#11679);
#8843=LINE('',#76178,#11680);
#8844=LINE('',#76180,#11681);
#8845=LINE('',#76181,#11682);
#8846=LINE('',#76183,#11683);
#8847=LINE('',#76184,#11684);
#8848=LINE('',#76189,#11685);
#8849=LINE('',#76191,#11686);
#8850=LINE('',#76193,#11687);
#8851=LINE('',#76194,#11688);
#8852=LINE('',#76197,#11689);
#8853=LINE('',#76199,#11690);
#8854=LINE('',#76200,#11691);
#8855=LINE('',#76203,#11692);
#8856=LINE('',#76205,#11693);
#8857=LINE('',#76206,#11694);
#8858=LINE('',#76208,#11695);
#8859=LINE('',#76209,#11696);
#8860=LINE('',#76214,#11697);
#8861=LINE('',#76216,#11698);
#8862=LINE('',#76218,#11699);
#8863=LINE('',#76219,#11700);
#8864=LINE('',#76222,#11701);
#8865=LINE('',#76224,#11702);
#8866=LINE('',#76225,#11703);
#8867=LINE('',#76228,#11704);
#8868=LINE('',#76230,#11705);
#8869=LINE('',#76231,#11706);
#8870=LINE('',#76233,#11707);
#8871=LINE('',#76234,#11708);
#8872=LINE('',#76239,#11709);
#8873=LINE('',#76241,#11710);
#8874=LINE('',#76243,#11711);
#8875=LINE('',#76244,#11712);
#8876=LINE('',#76247,#11713);
#8877=LINE('',#76249,#11714);
#8878=LINE('',#76250,#11715);
#8879=LINE('',#76253,#11716);
#8880=LINE('',#76255,#11717);
#8881=LINE('',#76256,#11718);
#8882=LINE('',#76258,#11719);
#8883=LINE('',#76259,#11720);
#8884=LINE('',#76264,#11721);
#8885=LINE('',#76266,#11722);
#8886=LINE('',#76268,#11723);
#8887=LINE('',#76269,#11724);
#8888=LINE('',#76272,#11725);
#8889=LINE('',#76274,#11726);
#8890=LINE('',#76275,#11727);
#8891=LINE('',#76278,#11728);
#8892=LINE('',#76280,#11729);
#8893=LINE('',#76281,#11730);
#8894=LINE('',#76283,#11731);
#8895=LINE('',#76284,#11732);
#8896=LINE('',#76289,#11733);
#8897=LINE('',#76291,#11734);
#8898=LINE('',#76293,#11735);
#8899=LINE('',#76294,#11736);
#8900=LINE('',#76297,#11737);
#8901=LINE('',#76299,#11738);
#8902=LINE('',#76300,#11739);
#8903=LINE('',#76303,#11740);
#8904=LINE('',#76305,#11741);
#8905=LINE('',#76306,#11742);
#8906=LINE('',#76308,#11743);
#8907=LINE('',#76309,#11744);
#8908=LINE('',#76314,#11745);
#8909=LINE('',#76316,#11746);
#8910=LINE('',#76318,#11747);
#8911=LINE('',#76319,#11748);
#8912=LINE('',#76322,#11749);
#8913=LINE('',#76324,#11750);
#8914=LINE('',#76325,#11751);
#8915=LINE('',#76328,#11752);
#8916=LINE('',#76330,#11753);
#8917=LINE('',#76331,#11754);
#8918=LINE('',#76333,#11755);
#8919=LINE('',#76334,#11756);
#8920=LINE('',#76339,#11757);
#8921=LINE('',#76341,#11758);
#8922=LINE('',#76343,#11759);
#8923=LINE('',#76344,#11760);
#8924=LINE('',#76347,#11761);
#8925=LINE('',#76349,#11762);
#8926=LINE('',#76350,#11763);
#8927=LINE('',#76353,#11764);
#8928=LINE('',#76355,#11765);
#8929=LINE('',#76356,#11766);
#8930=LINE('',#76358,#11767);
#8931=LINE('',#76359,#11768);
#8932=LINE('',#76364,#11769);
#8933=LINE('',#76366,#11770);
#8934=LINE('',#76368,#11771);
#8935=LINE('',#76369,#11772);
#8936=LINE('',#76372,#11773);
#8937=LINE('',#76374,#11774);
#8938=LINE('',#76375,#11775);
#8939=LINE('',#76378,#11776);
#8940=LINE('',#76380,#11777);
#8941=LINE('',#76381,#11778);
#8942=LINE('',#76383,#11779);
#8943=LINE('',#76384,#11780);
#8944=LINE('',#76389,#11781);
#8945=LINE('',#76391,#11782);
#8946=LINE('',#76393,#11783);
#8947=LINE('',#76394,#11784);
#8948=LINE('',#76397,#11785);
#8949=LINE('',#76399,#11786);
#8950=LINE('',#76400,#11787);
#8951=LINE('',#76403,#11788);
#8952=LINE('',#76405,#11789);
#8953=LINE('',#76406,#11790);
#8954=LINE('',#76408,#11791);
#8955=LINE('',#76409,#11792);
#8956=LINE('',#76414,#11793);
#8957=LINE('',#76416,#11794);
#8958=LINE('',#76418,#11795);
#8959=LINE('',#76419,#11796);
#8960=LINE('',#76422,#11797);
#8961=LINE('',#76424,#11798);
#8962=LINE('',#76425,#11799);
#8963=LINE('',#76428,#11800);
#8964=LINE('',#76430,#11801);
#8965=LINE('',#76431,#11802);
#8966=LINE('',#76433,#11803);
#8967=LINE('',#76434,#11804);
#8968=LINE('',#76439,#11805);
#8969=LINE('',#76441,#11806);
#8970=LINE('',#76443,#11807);
#8971=LINE('',#76444,#11808);
#8972=LINE('',#76447,#11809);
#8973=LINE('',#76449,#11810);
#8974=LINE('',#76450,#11811);
#8975=LINE('',#76453,#11812);
#8976=LINE('',#76455,#11813);
#8977=LINE('',#76456,#11814);
#8978=LINE('',#76458,#11815);
#8979=LINE('',#76459,#11816);
#8980=LINE('',#76464,#11817);
#8981=LINE('',#76466,#11818);
#8982=LINE('',#76468,#11819);
#8983=LINE('',#76469,#11820);
#8984=LINE('',#76472,#11821);
#8985=LINE('',#76474,#11822);
#8986=LINE('',#76475,#11823);
#8987=LINE('',#76478,#11824);
#8988=LINE('',#76480,#11825);
#8989=LINE('',#76481,#11826);
#8990=LINE('',#76483,#11827);
#8991=LINE('',#76484,#11828);
#8992=LINE('',#76489,#11829);
#8993=LINE('',#76491,#11830);
#8994=LINE('',#76493,#11831);
#8995=LINE('',#76494,#11832);
#8996=LINE('',#76497,#11833);
#8997=LINE('',#76499,#11834);
#8998=LINE('',#76500,#11835);
#8999=LINE('',#76503,#11836);
#9000=LINE('',#76505,#11837);
#9001=LINE('',#76506,#11838);
#9002=LINE('',#76508,#11839);
#9003=LINE('',#76509,#11840);
#9004=LINE('',#76514,#11841);
#9005=LINE('',#76516,#11842);
#9006=LINE('',#76518,#11843);
#9007=LINE('',#76519,#11844);
#9008=LINE('',#76522,#11845);
#9009=LINE('',#76524,#11846);
#9010=LINE('',#76525,#11847);
#9011=LINE('',#76528,#11848);
#9012=LINE('',#76530,#11849);
#9013=LINE('',#76531,#11850);
#9014=LINE('',#76533,#11851);
#9015=LINE('',#76534,#11852);
#9016=LINE('',#76539,#11853);
#9017=LINE('',#76541,#11854);
#9018=LINE('',#76543,#11855);
#9019=LINE('',#76544,#11856);
#9020=LINE('',#76547,#11857);
#9021=LINE('',#76549,#11858);
#9022=LINE('',#76550,#11859);
#9023=LINE('',#76553,#11860);
#9024=LINE('',#76555,#11861);
#9025=LINE('',#76556,#11862);
#9026=LINE('',#76558,#11863);
#9027=LINE('',#76559,#11864);
#9028=LINE('',#76564,#11865);
#9029=LINE('',#76566,#11866);
#9030=LINE('',#76568,#11867);
#9031=LINE('',#76569,#11868);
#9032=LINE('',#76572,#11869);
#9033=LINE('',#76574,#11870);
#9034=LINE('',#76575,#11871);
#9035=LINE('',#76578,#11872);
#9036=LINE('',#76580,#11873);
#9037=LINE('',#76581,#11874);
#9038=LINE('',#76583,#11875);
#9039=LINE('',#76584,#11876);
#9040=LINE('',#76590,#11877);
#9041=LINE('',#76596,#11878);
#9042=LINE('',#76601,#11879);
#9043=LINE('',#76603,#11880);
#9044=LINE('',#76605,#11881);
#9045=LINE('',#76606,#11882);
#9046=LINE('',#76612,#11883);
#9047=LINE('',#76615,#11884);
#9048=LINE('',#76617,#11885);
#9049=LINE('',#76618,#11886);
#9050=LINE('',#76624,#11887);
#9051=LINE('',#76627,#11888);
#9052=LINE('',#76629,#11889);
#9053=LINE('',#76630,#11890);
#9054=LINE('',#76636,#11891);
#9055=LINE('',#76639,#11892);
#9056=LINE('',#76641,#11893);
#9057=LINE('',#76642,#11894);
#10423=VECTOR('',#35792,10.);
#10424=VECTOR('',#35793,10.);
#10425=VECTOR('',#35794,10.);
#10426=VECTOR('',#35795,10.);
#10427=VECTOR('',#35796,10.);
#10428=VECTOR('',#35797,10.);
#10429=VECTOR('',#35798,10.);
#10430=VECTOR('',#35799,10.);
#10431=VECTOR('',#35800,10.);
#10432=VECTOR('',#35801,10.);
#10433=VECTOR('',#35802,10.);
#10434=VECTOR('',#35803,10.);
#10435=VECTOR('',#35804,10.);
#10436=VECTOR('',#35805,10.);
#10437=VECTOR('',#35806,10.);
#10438=VECTOR('',#35807,10.);
#10439=VECTOR('',#35808,10.);
#10440=VECTOR('',#35809,10.);
#10441=VECTOR('',#35810,10.);
#10442=VECTOR('',#35811,10.);
#10443=VECTOR('',#35816,10.);
#10444=VECTOR('',#35817,10.);
#10445=VECTOR('',#35818,10.);
#10446=VECTOR('',#35819,10.);
#10447=VECTOR('',#35822,10.);
#10448=VECTOR('',#35823,10.);
#10449=VECTOR('',#35824,10.);
#10450=VECTOR('',#35827,10.);
#10451=VECTOR('',#35828,10.);
#10452=VECTOR('',#35831,10.);
#10453=VECTOR('',#35832,10.);
#10454=VECTOR('',#35833,10.);
#10455=VECTOR('',#35834,10.);
#10456=VECTOR('',#35837,10.);
#10457=VECTOR('',#35838,10.);
#10458=VECTOR('',#35839,10.);
#10459=VECTOR('',#35842,10.);
#10460=VECTOR('',#35843,10.);
#10461=VECTOR('',#35844,10.);
#10462=VECTOR('',#35847,10.);
#10463=VECTOR('',#35848,10.);
#10464=VECTOR('',#35849,10.);
#10465=VECTOR('',#35852,10.);
#10466=VECTOR('',#35853,10.);
#10467=VECTOR('',#35854,10.);
#10468=VECTOR('',#35857,10.);
#10469=VECTOR('',#35858,10.);
#10470=VECTOR('',#35859,10.);
#10471=VECTOR('',#35862,9.99999999999999);
#10472=VECTOR('',#35863,10.);
#10473=VECTOR('',#35864,9.99999999999999);
#10474=VECTOR('',#35867,10.);
#10475=VECTOR('',#35868,10.);
#10476=VECTOR('',#35869,10.);
#10477=VECTOR('',#35872,10.);
#10478=VECTOR('',#35873,10.);
#10479=VECTOR('',#35874,10.);
#10480=VECTOR('',#35877,10.);
#10481=VECTOR('',#35878,10.);
#10482=VECTOR('',#35879,10.);
#10483=VECTOR('',#35882,10.);
#10484=VECTOR('',#35883,10.);
#10485=VECTOR('',#35890,10.);
#10486=VECTOR('',#35891,10.);
#10487=VECTOR('',#35892,10.);
#10488=VECTOR('',#35893,10.);
#10489=VECTOR('',#35894,10.);
#10490=VECTOR('',#35895,10.);
#10491=VECTOR('',#35896,10.);
#10492=VECTOR('',#35897,10.);
#10493=VECTOR('',#35898,10.);
#10494=VECTOR('',#35899,10.);
#10495=VECTOR('',#35900,10.);
#10496=VECTOR('',#35901,10.);
#10497=VECTOR('',#35902,10.);
#10498=VECTOR('',#35903,10.);
#10499=VECTOR('',#35904,10.);
#10500=VECTOR('',#35905,10.);
#10501=VECTOR('',#35906,10.);
#10502=VECTOR('',#35907,10.);
#10503=VECTOR('',#35908,10.);
#10504=VECTOR('',#35909,10.);
#10505=VECTOR('',#35912,10.);
#10506=VECTOR('',#35913,10.);
#10507=VECTOR('',#35914,10.);
#10508=VECTOR('',#35915,10.);
#10509=VECTOR('',#35916,10.);
#10510=VECTOR('',#35917,10.);
#10511=VECTOR('',#35918,10.);
#10512=VECTOR('',#35919,10.);
#10513=VECTOR('',#35920,10.);
#10514=VECTOR('',#35921,10.);
#10515=VECTOR('',#35922,10.);
#10516=VECTOR('',#35923,10.);
#10517=VECTOR('',#35924,10.);
#10518=VECTOR('',#35927,10.);
#10519=VECTOR('',#35928,10.);
#10520=VECTOR('',#35929,10.);
#10521=VECTOR('',#35930,10.);
#10522=VECTOR('',#35931,10.);
#10523=VECTOR('',#35932,10.);
#10524=VECTOR('',#35933,10.);
#10525=VECTOR('',#35934,10.);
#10526=VECTOR('',#35935,10.);
#10527=VECTOR('',#35936,10.);
#10528=VECTOR('',#35939,10.);
#10529=VECTOR('',#35940,10.);
#10530=VECTOR('',#35941,10.);
#10531=VECTOR('',#35942,10.);
#10532=VECTOR('',#35943,10.);
#10533=VECTOR('',#35944,10.);
#10534=VECTOR('',#35945,10.);
#10535=VECTOR('',#35946,10.);
#10536=VECTOR('',#35947,10.);
#10537=VECTOR('',#35948,10.);
#10538=VECTOR('',#35951,10.);
#10539=VECTOR('',#35952,10.);
#10540=VECTOR('',#35953,10.);
#10541=VECTOR('',#35958,10.);
#10542=VECTOR('',#35959,10.);
#10543=VECTOR('',#35960,10.);
#10544=VECTOR('',#35961,10.);
#10545=VECTOR('',#35962,10.);
#10546=VECTOR('',#35963,10.);
#10547=VECTOR('',#35964,10.);
#10548=VECTOR('',#35965,10.);
#10549=VECTOR('',#35966,10.);
#10550=VECTOR('',#35967,10.);
#10551=VECTOR('',#35968,10.);
#10552=VECTOR('',#35969,10.);
#10553=VECTOR('',#35970,10.);
#10554=VECTOR('',#35971,10.);
#10555=VECTOR('',#35972,10.);
#10556=VECTOR('',#35973,10.);
#10557=VECTOR('',#35974,10.);
#10558=VECTOR('',#35975,10.);
#10559=VECTOR('',#35976,10.);
#10560=VECTOR('',#35977,10.);
#10561=VECTOR('',#35980,10.);
#10562=VECTOR('',#35981,10.);
#10563=VECTOR('',#35982,10.);
#10564=VECTOR('',#35983,10.);
#10565=VECTOR('',#35984,10.);
#10566=VECTOR('',#35985,10.);
#10567=VECTOR('',#35986,10.);
#10568=VECTOR('',#35987,10.);
#10569=VECTOR('',#35988,10.);
#10570=VECTOR('',#35989,10.);
#10571=VECTOR('',#35992,10.);
#10572=VECTOR('',#35993,10.);
#10573=VECTOR('',#35994,10.);
#10574=VECTOR('',#35995,10.);
#10575=VECTOR('',#35996,10.);
#10576=VECTOR('',#35997,10.);
#10577=VECTOR('',#35998,10.);
#10578=VECTOR('',#35999,10.);
#10579=VECTOR('',#36000,10.);
#10580=VECTOR('',#36001,10.);
#10581=VECTOR('',#36002,10.);
#10582=VECTOR('',#36003,10.);
#10583=VECTOR('',#36006,10.);
#10584=VECTOR('',#36007,10.);
#10585=VECTOR('',#36008,10.);
#10586=VECTOR('',#36011,10.);
#10587=VECTOR('',#36012,10.);
#10588=VECTOR('',#36013,10.);
#10589=VECTOR('',#36016,10.);
#10590=VECTOR('',#36017,10.);
#10591=VECTOR('',#36022,10.);
#10592=VECTOR('',#36023,10.);
#10593=VECTOR('',#36024,10.);
#10594=VECTOR('',#36025,10.);
#10595=VECTOR('',#36026,10.);
#10596=VECTOR('',#36027,10.);
#10597=VECTOR('',#36028,10.);
#10598=VECTOR('',#36029,10.);
#10599=VECTOR('',#36030,10.);
#10600=VECTOR('',#36031,10.);
#10601=VECTOR('',#36032,10.);
#10602=VECTOR('',#36033,10.);
#10603=VECTOR('',#36034,10.);
#10604=VECTOR('',#36035,10.);
#10605=VECTOR('',#36036,10.);
#10606=VECTOR('',#36037,10.);
#10607=VECTOR('',#36038,10.);
#10608=VECTOR('',#36039,10.);
#10609=VECTOR('',#36040,10.);
#10610=VECTOR('',#36041,10.);
#10611=VECTOR('',#36046,10.);
#10612=VECTOR('',#36047,10.);
#10613=VECTOR('',#36048,10.);
#10614=VECTOR('',#36049,10.);
#10615=VECTOR('',#36050,10.);
#10616=VECTOR('',#36051,10.);
#10617=VECTOR('',#36054,10.);
#10618=VECTOR('',#36055,10.);
#10619=VECTOR('',#36056,10.);
#10620=VECTOR('',#36057,10.);
#10621=VECTOR('',#36058,10.);
#10622=VECTOR('',#36061,10.);
#10623=VECTOR('',#36062,10.);
#10624=VECTOR('',#36063,10.);
#10625=VECTOR('',#36066,10.);
#10626=VECTOR('',#36067,10.);
#10627=VECTOR('',#36068,10.);
#10628=VECTOR('',#36071,10.);
#10629=VECTOR('',#36072,10.);
#10630=VECTOR('',#36077,10.);
#10631=VECTOR('',#36078,10.);
#10632=VECTOR('',#36079,10.);
#10633=VECTOR('',#36080,10.);
#10634=VECTOR('',#36081,10.);
#10635=VECTOR('',#36082,10.);
#10636=VECTOR('',#36083,10.);
#10637=VECTOR('',#36084,10.);
#10638=VECTOR('',#36085,10.);
#10639=VECTOR('',#36086,10.);
#10640=VECTOR('',#36087,10.);
#10641=VECTOR('',#36088,10.);
#10642=VECTOR('',#36089,10.);
#10643=VECTOR('',#36090,10.);
#10644=VECTOR('',#36091,10.);
#10645=VECTOR('',#36092,10.);
#10646=VECTOR('',#36093,10.);
#10647=VECTOR('',#36094,10.);
#10648=VECTOR('',#36095,10.);
#10649=VECTOR('',#36096,10.);
#10650=VECTOR('',#36101,10.);
#10651=VECTOR('',#36102,10.);
#10652=VECTOR('',#36103,10.);
#10653=VECTOR('',#36104,10.);
#10654=VECTOR('',#36105,10.);
#10655=VECTOR('',#36106,10.);
#10656=VECTOR('',#36107,10.);
#10657=VECTOR('',#36108,10.);
#10658=VECTOR('',#36109,10.);
#10659=VECTOR('',#36110,10.);
#10660=VECTOR('',#36111,10.);
#10661=VECTOR('',#36112,10.);
#10662=VECTOR('',#36113,10.);
#10663=VECTOR('',#36114,10.);
#10664=VECTOR('',#36115,10.);
#10665=VECTOR('',#36116,10.);
#10666=VECTOR('',#36117,10.);
#10667=VECTOR('',#36118,10.);
#10668=VECTOR('',#36119,10.);
#10669=VECTOR('',#36120,10.);
#10670=VECTOR('',#36125,10.);
#10671=VECTOR('',#36126,10.);
#10672=VECTOR('',#36127,10.);
#10673=VECTOR('',#36128,10.);
#10674=VECTOR('',#36129,10.);
#10675=VECTOR('',#36130,10.);
#10676=VECTOR('',#36133,10.);
#10677=VECTOR('',#36134,10.);
#10678=VECTOR('',#36135,10.);
#10679=VECTOR('',#36136,10.);
#10680=VECTOR('',#36137,10.);
#10681=VECTOR('',#36140,10.);
#10682=VECTOR('',#36141,10.);
#10683=VECTOR('',#36142,10.);
#10684=VECTOR('',#36145,10.);
#10685=VECTOR('',#36146,10.);
#10686=VECTOR('',#36147,10.);
#10687=VECTOR('',#36150,10.);
#10688=VECTOR('',#36151,10.);
#10689=VECTOR('',#36156,10.);
#10690=VECTOR('',#36157,10.);
#10691=VECTOR('',#36158,10.);
#10692=VECTOR('',#36159,10.);
#10693=VECTOR('',#36160,10.);
#10694=VECTOR('',#36161,10.);
#10695=VECTOR('',#36162,10.);
#10696=VECTOR('',#36163,10.);
#10697=VECTOR('',#36164,10.);
#10698=VECTOR('',#36165,10.);
#10699=VECTOR('',#36166,10.);
#10700=VECTOR('',#36167,10.);
#10701=VECTOR('',#36168,10.);
#10702=VECTOR('',#36169,10.);
#10703=VECTOR('',#36170,10.);
#10704=VECTOR('',#36171,10.);
#10705=VECTOR('',#36172,10.);
#10706=VECTOR('',#36173,10.);
#10707=VECTOR('',#36174,10.);
#10708=VECTOR('',#36175,10.);
#10709=VECTOR('',#36178,10.);
#10710=VECTOR('',#36179,10.);
#10711=VECTOR('',#36180,10.);
#10712=VECTOR('',#36181,10.);
#10713=VECTOR('',#36182,10.);
#10714=VECTOR('',#36183,10.);
#10715=VECTOR('',#36184,10.);
#10716=VECTOR('',#36185,10.);
#10717=VECTOR('',#36186,10.);
#10718=VECTOR('',#36187,10.);
#10719=VECTOR('',#36190,10.);
#10720=VECTOR('',#36191,10.);
#10721=VECTOR('',#36192,10.);
#10722=VECTOR('',#36193,10.);
#10723=VECTOR('',#36194,10.);
#10724=VECTOR('',#36195,10.);
#10725=VECTOR('',#36196,10.);
#10726=VECTOR('',#36197,10.);
#10727=VECTOR('',#36198,10.);
#10728=VECTOR('',#36199,10.);
#10729=VECTOR('',#36200,10.);
#10730=VECTOR('',#36201,10.);
#10731=VECTOR('',#36204,10.);
#10732=VECTOR('',#36205,10.);
#10733=VECTOR('',#36206,10.);
#10734=VECTOR('',#36209,10.);
#10735=VECTOR('',#36210,10.);
#10736=VECTOR('',#36211,10.);
#10737=VECTOR('',#36214,10.);
#10738=VECTOR('',#36215,10.);
#10739=VECTOR('',#36220,10.);
#10740=VECTOR('',#36221,10.);
#10741=VECTOR('',#36222,10.);
#10742=VECTOR('',#36223,10.);
#10743=VECTOR('',#36224,10.);
#10744=VECTOR('',#36225,10.);
#10745=VECTOR('',#36226,10.);
#10746=VECTOR('',#36227,10.);
#10747=VECTOR('',#36228,10.);
#10748=VECTOR('',#36229,10.);
#10749=VECTOR('',#36230,10.);
#10750=VECTOR('',#36231,10.);
#10751=VECTOR('',#36232,10.);
#10752=VECTOR('',#36233,10.);
#10753=VECTOR('',#36234,10.);
#10754=VECTOR('',#36235,10.);
#10755=VECTOR('',#36236,10.);
#10756=VECTOR('',#36237,10.);
#10757=VECTOR('',#36238,10.);
#10758=VECTOR('',#36239,10.);
#10759=VECTOR('',#36242,10.);
#10760=VECTOR('',#36243,10.);
#10761=VECTOR('',#36244,10.);
#10762=VECTOR('',#36245,10.);
#10763=VECTOR('',#36246,10.);
#10764=VECTOR('',#36247,10.);
#10765=VECTOR('',#36248,10.);
#10766=VECTOR('',#36249,10.);
#10767=VECTOR('',#36250,10.);
#10768=VECTOR('',#36251,10.);
#10769=VECTOR('',#36252,10.);
#10770=VECTOR('',#36253,10.);
#10771=VECTOR('',#36254,10.);
#10772=VECTOR('',#36257,10.);
#10773=VECTOR('',#36258,10.);
#10774=VECTOR('',#36259,10.);
#10775=VECTOR('',#36260,10.);
#10776=VECTOR('',#36261,10.);
#10777=VECTOR('',#36262,10.);
#10778=VECTOR('',#36263,10.);
#10779=VECTOR('',#36264,10.);
#10780=VECTOR('',#36265,10.);
#10781=VECTOR('',#36266,10.);
#10782=VECTOR('',#36269,10.);
#10783=VECTOR('',#36270,10.);
#10784=VECTOR('',#36271,10.);
#10785=VECTOR('',#36272,10.);
#10786=VECTOR('',#36273,10.);
#10787=VECTOR('',#36274,10.);
#10788=VECTOR('',#36275,10.);
#10789=VECTOR('',#36276,10.);
#10790=VECTOR('',#36277,10.);
#10791=VECTOR('',#36278,10.);
#10792=VECTOR('',#36281,10.);
#10793=VECTOR('',#36282,10.);
#10794=VECTOR('',#36283,10.);
#10795=VECTOR('',#36288,10.);
#10796=VECTOR('',#36289,10.);
#10797=VECTOR('',#36290,10.);
#10798=VECTOR('',#36291,10.);
#10799=VECTOR('',#36292,10.);
#10800=VECTOR('',#36293,10.);
#10801=VECTOR('',#36294,10.);
#10802=VECTOR('',#36295,10.);
#10803=VECTOR('',#36296,10.);
#10804=VECTOR('',#36297,10.);
#10805=VECTOR('',#36298,10.);
#10806=VECTOR('',#36299,10.);
#10807=VECTOR('',#36300,10.);
#10808=VECTOR('',#36301,10.);
#10809=VECTOR('',#36302,10.);
#10810=VECTOR('',#36303,10.);
#10811=VECTOR('',#36304,10.);
#10812=VECTOR('',#36305,10.);
#10813=VECTOR('',#36306,10.);
#10814=VECTOR('',#36307,10.);
#10815=VECTOR('',#36312,10.);
#10816=VECTOR('',#36313,10.);
#10817=VECTOR('',#36314,10.);
#10818=VECTOR('',#36315,10.);
#10819=VECTOR('',#36318,10.);
#10820=VECTOR('',#36319,10.);
#10821=VECTOR('',#36320,10.);
#10822=VECTOR('',#36323,10.);
#10823=VECTOR('',#36324,10.);
#10824=VECTOR('',#36327,10.);
#10825=VECTOR('',#36328,10.);
#10826=VECTOR('',#36329,10.);
#10827=VECTOR('',#36330,10.);
#10828=VECTOR('',#36333,10.);
#10829=VECTOR('',#36334,10.);
#10830=VECTOR('',#36335,10.);
#10831=VECTOR('',#36338,10.);
#10832=VECTOR('',#36339,10.);
#10833=VECTOR('',#36340,10.);
#10834=VECTOR('',#36343,10.);
#10835=VECTOR('',#36344,10.);
#10836=VECTOR('',#36345,10.);
#10837=VECTOR('',#36348,10.);
#10838=VECTOR('',#36349,10.);
#10839=VECTOR('',#36350,10.);
#10840=VECTOR('',#36353,10.);
#10841=VECTOR('',#36354,10.);
#10842=VECTOR('',#36355,10.);
#10843=VECTOR('',#36358,9.99999999999999);
#10844=VECTOR('',#36359,10.);
#10845=VECTOR('',#36360,9.99999999999999);
#10846=VECTOR('',#36363,10.);
#10847=VECTOR('',#36364,10.);
#10848=VECTOR('',#36365,10.);
#10849=VECTOR('',#36368,10.);
#10850=VECTOR('',#36369,10.);
#10851=VECTOR('',#36370,10.);
#10852=VECTOR('',#36373,10.);
#10853=VECTOR('',#36374,10.);
#10854=VECTOR('',#36375,10.);
#10855=VECTOR('',#36378,10.);
#10856=VECTOR('',#36379,10.);
#10857=VECTOR('',#36388,10.);
#10858=VECTOR('',#36389,10.);
#10859=VECTOR('',#36390,10.);
#10860=VECTOR('',#36391,10.);
#10861=VECTOR('',#36394,10.);
#10862=VECTOR('',#36395,10.);
#10863=VECTOR('',#36396,10.);
#10864=VECTOR('',#36399,10.);
#10865=VECTOR('',#36400,10.);
#10866=VECTOR('',#36401,10.);
#10867=VECTOR('',#36404,10.);
#10868=VECTOR('',#36405,10.);
#10869=VECTOR('',#36410,10.);
#10870=VECTOR('',#36411,10.);
#10871=VECTOR('',#36412,10.);
#10872=VECTOR('',#36413,10.);
#10873=VECTOR('',#36416,10.);
#10874=VECTOR('',#36417,10.);
#10875=VECTOR('',#36418,10.);
#10876=VECTOR('',#36421,10.);
#10877=VECTOR('',#36422,10.);
#10878=VECTOR('',#36423,10.);
#10879=VECTOR('',#36426,10.);
#10880=VECTOR('',#36427,10.);
#10881=VECTOR('',#36432,10.);
#10882=VECTOR('',#36433,10.);
#10883=VECTOR('',#36434,10.);
#10884=VECTOR('',#36435,10.);
#10885=VECTOR('',#36438,10.);
#10886=VECTOR('',#36439,10.);
#10887=VECTOR('',#36440,10.);
#10888=VECTOR('',#36443,10.);
#10889=VECTOR('',#36444,10.);
#10890=VECTOR('',#36445,10.);
#10891=VECTOR('',#36448,10.);
#10892=VECTOR('',#36449,10.);
#10893=VECTOR('',#36454,10.);
#10894=VECTOR('',#36455,10.);
#10895=VECTOR('',#36456,10.);
#10896=VECTOR('',#36457,10.);
#10897=VECTOR('',#36460,10.);
#10898=VECTOR('',#36461,10.);
#10899=VECTOR('',#36462,10.);
#10900=VECTOR('',#36465,10.);
#10901=VECTOR('',#36466,10.);
#10902=VECTOR('',#36467,10.);
#10903=VECTOR('',#36470,10.);
#10904=VECTOR('',#36471,10.);
#10905=VECTOR('',#36476,10.);
#10906=VECTOR('',#36477,10.);
#10907=VECTOR('',#36478,10.);
#10908=VECTOR('',#36479,10.);
#10909=VECTOR('',#36482,10.);
#10910=VECTOR('',#36483,10.);
#10911=VECTOR('',#36484,10.);
#10912=VECTOR('',#36487,10.);
#10913=VECTOR('',#36488,10.);
#10914=VECTOR('',#36489,10.);
#10915=VECTOR('',#36492,10.);
#10916=VECTOR('',#36493,10.);
#10917=VECTOR('',#36498,10.);
#10918=VECTOR('',#36499,10.);
#10919=VECTOR('',#36500,10.);
#10920=VECTOR('',#36501,10.);
#10921=VECTOR('',#36504,10.);
#10922=VECTOR('',#36505,10.);
#10923=VECTOR('',#36506,10.);
#10924=VECTOR('',#36509,10.);
#10925=VECTOR('',#36510,10.);
#10926=VECTOR('',#36511,10.);
#10927=VECTOR('',#36514,10.);
#10928=VECTOR('',#36515,10.);
#10929=VECTOR('',#36520,10.);
#10930=VECTOR('',#36521,10.);
#10931=VECTOR('',#36522,10.);
#10932=VECTOR('',#36523,10.);
#10933=VECTOR('',#36526,10.);
#10934=VECTOR('',#36527,10.);
#10935=VECTOR('',#36528,10.);
#10936=VECTOR('',#36531,10.);
#10937=VECTOR('',#36532,10.);
#10938=VECTOR('',#36533,10.);
#10939=VECTOR('',#36536,10.);
#10940=VECTOR('',#36537,10.);
#10941=VECTOR('',#36542,10.);
#10942=VECTOR('',#36543,10.);
#10943=VECTOR('',#36544,10.);
#10944=VECTOR('',#36545,10.);
#10945=VECTOR('',#36548,10.);
#10946=VECTOR('',#36549,10.);
#10947=VECTOR('',#36550,10.);
#10948=VECTOR('',#36553,10.);
#10949=VECTOR('',#36554,10.);
#10950=VECTOR('',#36555,10.);
#10951=VECTOR('',#36558,10.);
#10952=VECTOR('',#36559,10.);
#10953=VECTOR('',#36564,10.);
#10954=VECTOR('',#36565,10.);
#10955=VECTOR('',#36566,10.);
#10956=VECTOR('',#36567,10.);
#10957=VECTOR('',#36570,10.);
#10958=VECTOR('',#36571,10.);
#10959=VECTOR('',#36572,10.);
#10960=VECTOR('',#36575,10.);
#10961=VECTOR('',#36576,10.);
#10962=VECTOR('',#36577,10.);
#10963=VECTOR('',#36580,10.);
#10964=VECTOR('',#36581,10.);
#10965=VECTOR('',#36586,10.);
#10966=VECTOR('',#36587,10.);
#10967=VECTOR('',#36588,10.);
#10968=VECTOR('',#36589,10.);
#10969=VECTOR('',#36592,10.);
#10970=VECTOR('',#36593,10.);
#10971=VECTOR('',#36594,10.);
#10972=VECTOR('',#36597,10.);
#10973=VECTOR('',#36598,10.);
#10974=VECTOR('',#36599,10.);
#10975=VECTOR('',#36602,10.);
#10976=VECTOR('',#36603,10.);
#10977=VECTOR('',#36608,10.);
#10978=VECTOR('',#36609,10.);
#10979=VECTOR('',#36610,10.);
#10980=VECTOR('',#36611,10.);
#10981=VECTOR('',#36614,10.);
#10982=VECTOR('',#36615,10.);
#10983=VECTOR('',#36616,10.);
#10984=VECTOR('',#36619,10.);
#10985=VECTOR('',#36620,10.);
#10986=VECTOR('',#36621,10.);
#10987=VECTOR('',#36624,10.);
#10988=VECTOR('',#36625,10.);
#10989=VECTOR('',#36630,10.);
#10990=VECTOR('',#36631,10.);
#10991=VECTOR('',#36632,10.);
#10992=VECTOR('',#36633,10.);
#10993=VECTOR('',#36636,10.);
#10994=VECTOR('',#36637,10.);
#10995=VECTOR('',#36638,10.);
#10996=VECTOR('',#36641,10.);
#10997=VECTOR('',#36642,10.);
#10998=VECTOR('',#36643,10.);
#10999=VECTOR('',#36646,10.);
#11000=VECTOR('',#36647,10.);
#11001=VECTOR('',#36652,10.);
#11002=VECTOR('',#36653,10.);
#11003=VECTOR('',#36654,10.);
#11004=VECTOR('',#36655,10.);
#11005=VECTOR('',#36658,10.);
#11006=VECTOR('',#36659,10.);
#11007=VECTOR('',#36660,10.);
#11008=VECTOR('',#36663,10.);
#11009=VECTOR('',#36664,10.);
#11010=VECTOR('',#36665,10.);
#11011=VECTOR('',#36668,10.);
#11012=VECTOR('',#36669,10.);
#11013=VECTOR('',#36674,10.);
#11014=VECTOR('',#36675,10.);
#11015=VECTOR('',#36676,10.);
#11016=VECTOR('',#36677,10.);
#11017=VECTOR('',#36680,10.);
#11018=VECTOR('',#36681,10.);
#11019=VECTOR('',#36682,10.);
#11020=VECTOR('',#36685,10.);
#11021=VECTOR('',#36686,10.);
#11022=VECTOR('',#36687,10.);
#11023=VECTOR('',#36690,10.);
#11024=VECTOR('',#36691,10.);
#11025=VECTOR('',#36696,10.);
#11026=VECTOR('',#36697,10.);
#11027=VECTOR('',#36698,10.);
#11028=VECTOR('',#36699,10.);
#11029=VECTOR('',#36702,10.);
#11030=VECTOR('',#36703,10.);
#11031=VECTOR('',#36704,10.);
#11032=VECTOR('',#36707,10.);
#11033=VECTOR('',#36708,10.);
#11034=VECTOR('',#36709,10.);
#11035=VECTOR('',#36712,10.);
#11036=VECTOR('',#36713,10.);
#11037=VECTOR('',#36718,10.);
#11038=VECTOR('',#36719,10.);
#11039=VECTOR('',#36720,10.);
#11040=VECTOR('',#36721,10.);
#11041=VECTOR('',#36724,10.);
#11042=VECTOR('',#36725,10.);
#11043=VECTOR('',#36726,10.);
#11044=VECTOR('',#36729,10.);
#11045=VECTOR('',#36730,10.);
#11046=VECTOR('',#36731,10.);
#11047=VECTOR('',#36734,10.);
#11048=VECTOR('',#36735,10.);
#11049=VECTOR('',#36740,10.);
#11050=VECTOR('',#36741,10.);
#11051=VECTOR('',#36742,10.);
#11052=VECTOR('',#36743,10.);
#11053=VECTOR('',#36746,10.);
#11054=VECTOR('',#36747,10.);
#11055=VECTOR('',#36748,10.);
#11056=VECTOR('',#36751,10.);
#11057=VECTOR('',#36752,10.);
#11058=VECTOR('',#36753,10.);
#11059=VECTOR('',#36756,10.);
#11060=VECTOR('',#36757,10.);
#11061=VECTOR('',#36762,10.);
#11062=VECTOR('',#36763,10.);
#11063=VECTOR('',#36764,10.);
#11064=VECTOR('',#36765,10.);
#11065=VECTOR('',#36768,10.);
#11066=VECTOR('',#36769,10.);
#11067=VECTOR('',#36770,10.);
#11068=VECTOR('',#36773,10.);
#11069=VECTOR('',#36774,10.);
#11070=VECTOR('',#36775,10.);
#11071=VECTOR('',#36778,10.);
#11072=VECTOR('',#36779,10.);
#11073=VECTOR('',#36784,10.);
#11074=VECTOR('',#36785,10.);
#11075=VECTOR('',#36786,10.);
#11076=VECTOR('',#36787,10.);
#11077=VECTOR('',#36790,10.);
#11078=VECTOR('',#36791,10.);
#11079=VECTOR('',#36792,10.);
#11080=VECTOR('',#36795,10.);
#11081=VECTOR('',#36796,10.);
#11082=VECTOR('',#36797,10.);
#11083=VECTOR('',#36800,10.);
#11084=VECTOR('',#36801,10.);
#11085=VECTOR('',#36806,10.);
#11086=VECTOR('',#36807,10.);
#11087=VECTOR('',#36808,10.);
#11088=VECTOR('',#36809,10.);
#11089=VECTOR('',#36812,10.);
#11090=VECTOR('',#36813,10.);
#11091=VECTOR('',#36814,10.);
#11092=VECTOR('',#36817,10.);
#11093=VECTOR('',#36818,10.);
#11094=VECTOR('',#36819,10.);
#11095=VECTOR('',#36822,10.);
#11096=VECTOR('',#36823,10.);
#11097=VECTOR('',#36828,10.);
#11098=VECTOR('',#36829,10.);
#11099=VECTOR('',#36830,10.);
#11100=VECTOR('',#36831,10.);
#11101=VECTOR('',#36834,10.);
#11102=VECTOR('',#36835,10.);
#11103=VECTOR('',#36836,10.);
#11104=VECTOR('',#36839,10.);
#11105=VECTOR('',#36840,10.);
#11106=VECTOR('',#36841,10.);
#11107=VECTOR('',#36844,10.);
#11108=VECTOR('',#36845,10.);
#11109=VECTOR('',#36850,10.);
#11110=VECTOR('',#36851,10.);
#11111=VECTOR('',#36852,10.);
#11112=VECTOR('',#36853,10.);
#11113=VECTOR('',#36856,10.);
#11114=VECTOR('',#36857,10.);
#11115=VECTOR('',#36858,10.);
#11116=VECTOR('',#36861,10.);
#11117=VECTOR('',#36862,10.);
#11118=VECTOR('',#36863,10.);
#11119=VECTOR('',#36866,10.);
#11120=VECTOR('',#36867,10.);
#11121=VECTOR('',#36872,10.);
#11122=VECTOR('',#36873,10.);
#11123=VECTOR('',#36874,10.);
#11124=VECTOR('',#36875,10.);
#11125=VECTOR('',#36878,10.);
#11126=VECTOR('',#36879,10.);
#11127=VECTOR('',#36880,10.);
#11128=VECTOR('',#36883,10.);
#11129=VECTOR('',#36884,10.);
#11130=VECTOR('',#36885,10.);
#11131=VECTOR('',#36888,10.);
#11132=VECTOR('',#36889,10.);
#11133=VECTOR('',#36894,10.);
#11134=VECTOR('',#36895,10.);
#11135=VECTOR('',#36896,10.);
#11136=VECTOR('',#36897,10.);
#11137=VECTOR('',#36900,10.);
#11138=VECTOR('',#36901,10.);
#11139=VECTOR('',#36902,10.);
#11140=VECTOR('',#36905,10.);
#11141=VECTOR('',#36906,10.);
#11142=VECTOR('',#36907,10.);
#11143=VECTOR('',#36910,10.);
#11144=VECTOR('',#36911,10.);
#11145=VECTOR('',#36916,10.);
#11146=VECTOR('',#36917,10.);
#11147=VECTOR('',#36918,10.);
#11148=VECTOR('',#36919,10.);
#11149=VECTOR('',#36922,10.);
#11150=VECTOR('',#36923,10.);
#11151=VECTOR('',#36924,10.);
#11152=VECTOR('',#36927,10.);
#11153=VECTOR('',#36928,10.);
#11154=VECTOR('',#36929,10.);
#11155=VECTOR('',#36932,10.);
#11156=VECTOR('',#36933,10.);
#11157=VECTOR('',#36938,10.);
#11158=VECTOR('',#36939,10.);
#11159=VECTOR('',#36940,10.);
#11160=VECTOR('',#36941,10.);
#11161=VECTOR('',#36944,10.);
#11162=VECTOR('',#36945,10.);
#11163=VECTOR('',#36946,10.);
#11164=VECTOR('',#36949,10.);
#11165=VECTOR('',#36950,10.);
#11166=VECTOR('',#36951,10.);
#11167=VECTOR('',#36954,10.);
#11168=VECTOR('',#36955,10.);
#11169=VECTOR('',#36960,10.);
#11170=VECTOR('',#36961,10.);
#11171=VECTOR('',#36962,10.);
#11172=VECTOR('',#36963,10.);
#11173=VECTOR('',#36966,10.);
#11174=VECTOR('',#36967,10.);
#11175=VECTOR('',#36968,10.);
#11176=VECTOR('',#36971,10.);
#11177=VECTOR('',#36972,10.);
#11178=VECTOR('',#36973,10.);
#11179=VECTOR('',#36976,10.);
#11180=VECTOR('',#36977,10.);
#11181=VECTOR('',#36982,10.);
#11182=VECTOR('',#36983,10.);
#11183=VECTOR('',#36984,10.);
#11184=VECTOR('',#36985,10.);
#11185=VECTOR('',#36988,10.);
#11186=VECTOR('',#36989,10.);
#11187=VECTOR('',#36990,10.);
#11188=VECTOR('',#36993,10.);
#11189=VECTOR('',#36994,10.);
#11190=VECTOR('',#36995,10.);
#11191=VECTOR('',#36998,10.);
#11192=VECTOR('',#36999,10.);
#11193=VECTOR('',#37004,10.);
#11194=VECTOR('',#37005,10.);
#11195=VECTOR('',#37006,10.);
#11196=VECTOR('',#37007,10.);
#11197=VECTOR('',#37010,10.);
#11198=VECTOR('',#37011,10.);
#11199=VECTOR('',#37012,10.);
#11200=VECTOR('',#37015,10.);
#11201=VECTOR('',#37016,10.);
#11202=VECTOR('',#37017,10.);
#11203=VECTOR('',#37020,10.);
#11204=VECTOR('',#37021,10.);
#11205=VECTOR('',#37026,10.);
#11206=VECTOR('',#37027,10.);
#11207=VECTOR('',#37028,10.);
#11208=VECTOR('',#37029,10.);
#11209=VECTOR('',#37032,10.);
#11210=VECTOR('',#37033,10.);
#11211=VECTOR('',#37034,10.);
#11212=VECTOR('',#37037,10.);
#11213=VECTOR('',#37038,10.);
#11214=VECTOR('',#37039,10.);
#11215=VECTOR('',#37042,10.);
#11216=VECTOR('',#37043,10.);
#11217=VECTOR('',#37048,10.);
#11218=VECTOR('',#37049,10.);
#11219=VECTOR('',#37050,10.);
#11220=VECTOR('',#37051,10.);
#11221=VECTOR('',#37054,10.);
#11222=VECTOR('',#37055,10.);
#11223=VECTOR('',#37056,10.);
#11224=VECTOR('',#37059,10.);
#11225=VECTOR('',#37060,10.);
#11226=VECTOR('',#37061,10.);
#11227=VECTOR('',#37064,10.);
#11228=VECTOR('',#37065,10.);
#11229=VECTOR('',#37070,10.);
#11230=VECTOR('',#37071,10.);
#11231=VECTOR('',#37072,10.);
#11232=VECTOR('',#37073,10.);
#11233=VECTOR('',#37076,10.);
#11234=VECTOR('',#37077,10.);
#11235=VECTOR('',#37078,10.);
#11236=VECTOR('',#37081,10.);
#11237=VECTOR('',#37082,10.);
#11238=VECTOR('',#37083,10.);
#11239=VECTOR('',#37086,10.);
#11240=VECTOR('',#37087,10.);
#11241=VECTOR('',#37092,10.);
#11242=VECTOR('',#37093,10.);
#11243=VECTOR('',#37094,10.);
#11244=VECTOR('',#37095,10.);
#11245=VECTOR('',#37098,10.);
#11246=VECTOR('',#37099,10.);
#11247=VECTOR('',#37100,10.);
#11248=VECTOR('',#37103,10.);
#11249=VECTOR('',#37104,10.);
#11250=VECTOR('',#37105,10.);
#11251=VECTOR('',#37108,10.);
#11252=VECTOR('',#37109,10.);
#11253=VECTOR('',#37114,10.);
#11254=VECTOR('',#37115,10.);
#11255=VECTOR('',#37116,10.);
#11256=VECTOR('',#37117,10.);
#11257=VECTOR('',#37120,10.);
#11258=VECTOR('',#37121,10.);
#11259=VECTOR('',#37122,10.);
#11260=VECTOR('',#37125,10.);
#11261=VECTOR('',#37126,10.);
#11262=VECTOR('',#37127,10.);
#11263=VECTOR('',#37130,10.);
#11264=VECTOR('',#37131,10.);
#11265=VECTOR('',#37136,10.);
#11266=VECTOR('',#37137,10.);
#11267=VECTOR('',#37138,10.);
#11268=VECTOR('',#37139,10.);
#11269=VECTOR('',#37142,10.);
#11270=VECTOR('',#37143,10.);
#11271=VECTOR('',#37144,10.);
#11272=VECTOR('',#37147,10.);
#11273=VECTOR('',#37148,10.);
#11274=VECTOR('',#37149,10.);
#11275=VECTOR('',#37152,10.);
#11276=VECTOR('',#37153,10.);
#11277=VECTOR('',#37158,10.);
#11278=VECTOR('',#37159,10.);
#11279=VECTOR('',#37160,10.);
#11280=VECTOR('',#37161,10.);
#11281=VECTOR('',#37164,10.);
#11282=VECTOR('',#37165,10.);
#11283=VECTOR('',#37166,10.);
#11284=VECTOR('',#37169,10.);
#11285=VECTOR('',#37170,10.);
#11286=VECTOR('',#37171,10.);
#11287=VECTOR('',#37174,10.);
#11288=VECTOR('',#37175,10.);
#11289=VECTOR('',#37180,10.);
#11290=VECTOR('',#37181,10.);
#11291=VECTOR('',#37182,10.);
#11292=VECTOR('',#37183,10.);
#11293=VECTOR('',#37186,10.);
#11294=VECTOR('',#37187,10.);
#11295=VECTOR('',#37188,10.);
#11296=VECTOR('',#37191,10.);
#11297=VECTOR('',#37192,10.);
#11298=VECTOR('',#37193,10.);
#11299=VECTOR('',#37196,10.);
#11300=VECTOR('',#37197,10.);
#11301=VECTOR('',#37202,10.);
#11302=VECTOR('',#37203,10.);
#11303=VECTOR('',#37204,10.);
#11304=VECTOR('',#37205,10.);
#11305=VECTOR('',#37208,10.);
#11306=VECTOR('',#37209,10.);
#11307=VECTOR('',#37210,10.);
#11308=VECTOR('',#37213,10.);
#11309=VECTOR('',#37214,10.);
#11310=VECTOR('',#37215,10.);
#11311=VECTOR('',#37218,10.);
#11312=VECTOR('',#37219,10.);
#11313=VECTOR('',#37224,10.);
#11314=VECTOR('',#37225,10.);
#11315=VECTOR('',#37226,10.);
#11316=VECTOR('',#37227,10.);
#11317=VECTOR('',#37230,10.);
#11318=VECTOR('',#37231,10.);
#11319=VECTOR('',#37232,10.);
#11320=VECTOR('',#37235,10.);
#11321=VECTOR('',#37236,10.);
#11322=VECTOR('',#37237,10.);
#11323=VECTOR('',#37240,10.);
#11324=VECTOR('',#37241,10.);
#11325=VECTOR('',#37246,10.);
#11326=VECTOR('',#37247,10.);
#11327=VECTOR('',#37248,10.);
#11328=VECTOR('',#37249,10.);
#11329=VECTOR('',#37252,10.);
#11330=VECTOR('',#37253,10.);
#11331=VECTOR('',#37254,10.);
#11332=VECTOR('',#37257,10.);
#11333=VECTOR('',#37258,10.);
#11334=VECTOR('',#37259,10.);
#11335=VECTOR('',#37262,10.);
#11336=VECTOR('',#37263,10.);
#11337=VECTOR('',#37268,10.);
#11338=VECTOR('',#37269,10.);
#11339=VECTOR('',#37270,10.);
#11340=VECTOR('',#37271,10.);
#11341=VECTOR('',#37274,10.);
#11342=VECTOR('',#37275,10.);
#11343=VECTOR('',#37276,10.);
#11344=VECTOR('',#37279,10.);
#11345=VECTOR('',#37280,10.);
#11346=VECTOR('',#37281,10.);
#11347=VECTOR('',#37284,10.);
#11348=VECTOR('',#37285,10.);
#11349=VECTOR('',#37290,10.);
#11350=VECTOR('',#37291,10.);
#11351=VECTOR('',#37292,10.);
#11352=VECTOR('',#37293,10.);
#11353=VECTOR('',#37296,10.);
#11354=VECTOR('',#37297,10.);
#11355=VECTOR('',#37298,10.);
#11356=VECTOR('',#37301,10.);
#11357=VECTOR('',#37302,10.);
#11358=VECTOR('',#37303,10.);
#11359=VECTOR('',#37306,10.);
#11360=VECTOR('',#37307,10.);
#11361=VECTOR('',#37312,10.);
#11362=VECTOR('',#37313,10.);
#11363=VECTOR('',#37314,10.);
#11364=VECTOR('',#37315,10.);
#11365=VECTOR('',#37318,10.);
#11366=VECTOR('',#37319,10.);
#11367=VECTOR('',#37320,10.);
#11368=VECTOR('',#37323,10.);
#11369=VECTOR('',#37324,10.);
#11370=VECTOR('',#37325,10.);
#11371=VECTOR('',#37328,10.);
#11372=VECTOR('',#37329,10.);
#11373=VECTOR('',#37334,10.);
#11374=VECTOR('',#37335,10.);
#11375=VECTOR('',#37336,10.);
#11376=VECTOR('',#37337,10.);
#11377=VECTOR('',#37340,10.);
#11378=VECTOR('',#37341,10.);
#11379=VECTOR('',#37342,10.);
#11380=VECTOR('',#37345,10.);
#11381=VECTOR('',#37346,10.);
#11382=VECTOR('',#37347,10.);
#11383=VECTOR('',#37350,10.);
#11384=VECTOR('',#37351,10.);
#11385=VECTOR('',#37356,10.);
#11386=VECTOR('',#37357,10.);
#11387=VECTOR('',#37358,10.);
#11388=VECTOR('',#37359,10.);
#11389=VECTOR('',#37362,10.);
#11390=VECTOR('',#37363,10.);
#11391=VECTOR('',#37364,10.);
#11392=VECTOR('',#37367,10.);
#11393=VECTOR('',#37368,10.);
#11394=VECTOR('',#37369,10.);
#11395=VECTOR('',#37372,10.);
#11396=VECTOR('',#37373,10.);
#11397=VECTOR('',#37378,10.);
#11398=VECTOR('',#37379,10.);
#11399=VECTOR('',#37380,10.);
#11400=VECTOR('',#37381,10.);
#11401=VECTOR('',#37384,10.);
#11402=VECTOR('',#37385,10.);
#11403=VECTOR('',#37386,10.);
#11404=VECTOR('',#37389,10.);
#11405=VECTOR('',#37390,10.);
#11406=VECTOR('',#37391,10.);
#11407=VECTOR('',#37394,10.);
#11408=VECTOR('',#37395,10.);
#11409=VECTOR('',#37400,10.);
#11410=VECTOR('',#37401,10.);
#11411=VECTOR('',#37402,10.);
#11412=VECTOR('',#37403,10.);
#11413=VECTOR('',#37406,10.);
#11414=VECTOR('',#37407,10.);
#11415=VECTOR('',#37408,10.);
#11416=VECTOR('',#37411,10.);
#11417=VECTOR('',#37412,10.);
#11418=VECTOR('',#37413,10.);
#11419=VECTOR('',#37416,10.);
#11420=VECTOR('',#37417,10.);
#11421=VECTOR('',#37422,10.);
#11422=VECTOR('',#37423,10.);
#11423=VECTOR('',#37424,10.);
#11424=VECTOR('',#37425,10.);
#11425=VECTOR('',#37428,10.);
#11426=VECTOR('',#37429,10.);
#11427=VECTOR('',#37430,10.);
#11428=VECTOR('',#37433,10.);
#11429=VECTOR('',#37434,10.);
#11430=VECTOR('',#37435,10.);
#11431=VECTOR('',#37438,10.);
#11432=VECTOR('',#37439,10.);
#11433=VECTOR('',#37444,10.);
#11434=VECTOR('',#37445,10.);
#11435=VECTOR('',#37446,10.);
#11436=VECTOR('',#37447,10.);
#11437=VECTOR('',#37450,10.);
#11438=VECTOR('',#37451,10.);
#11439=VECTOR('',#37452,10.);
#11440=VECTOR('',#37455,10.);
#11441=VECTOR('',#37456,10.);
#11442=VECTOR('',#37457,10.);
#11443=VECTOR('',#37460,10.);
#11444=VECTOR('',#37461,10.);
#11445=VECTOR('',#37466,10.);
#11446=VECTOR('',#37467,10.);
#11447=VECTOR('',#37468,10.);
#11448=VECTOR('',#37469,10.);
#11449=VECTOR('',#37472,10.);
#11450=VECTOR('',#37473,10.);
#11451=VECTOR('',#37474,10.);
#11452=VECTOR('',#37477,10.);
#11453=VECTOR('',#37478,10.);
#11454=VECTOR('',#37479,10.);
#11455=VECTOR('',#37482,10.);
#11456=VECTOR('',#37483,10.);
#11457=VECTOR('',#37488,10.);
#11458=VECTOR('',#37489,10.);
#11459=VECTOR('',#37490,10.);
#11460=VECTOR('',#37491,10.);
#11461=VECTOR('',#37494,10.);
#11462=VECTOR('',#37495,10.);
#11463=VECTOR('',#37496,10.);
#11464=VECTOR('',#37499,10.);
#11465=VECTOR('',#37500,10.);
#11466=VECTOR('',#37501,10.);
#11467=VECTOR('',#37504,10.);
#11468=VECTOR('',#37505,10.);
#11469=VECTOR('',#37510,10.);
#11470=VECTOR('',#37511,10.);
#11471=VECTOR('',#37512,10.);
#11472=VECTOR('',#37513,10.);
#11473=VECTOR('',#37516,10.);
#11474=VECTOR('',#37517,10.);
#11475=VECTOR('',#37518,10.);
#11476=VECTOR('',#37521,10.);
#11477=VECTOR('',#37522,10.);
#11478=VECTOR('',#37523,10.);
#11479=VECTOR('',#37526,10.);
#11480=VECTOR('',#37527,10.);
#11481=VECTOR('',#37532,10.);
#11482=VECTOR('',#37533,10.);
#11483=VECTOR('',#37534,10.);
#11484=VECTOR('',#37535,10.);
#11485=VECTOR('',#37538,10.);
#11486=VECTOR('',#37539,10.);
#11487=VECTOR('',#37540,10.);
#11488=VECTOR('',#37543,10.);
#11489=VECTOR('',#37544,10.);
#11490=VECTOR('',#37545,10.);
#11491=VECTOR('',#37548,10.);
#11492=VECTOR('',#37549,10.);
#11493=VECTOR('',#37554,10.);
#11494=VECTOR('',#37555,10.);
#11495=VECTOR('',#37556,10.);
#11496=VECTOR('',#37557,10.);
#11497=VECTOR('',#37560,10.);
#11498=VECTOR('',#37561,10.);
#11499=VECTOR('',#37562,10.);
#11500=VECTOR('',#37565,10.);
#11501=VECTOR('',#37566,10.);
#11502=VECTOR('',#37567,10.);
#11503=VECTOR('',#37570,10.);
#11504=VECTOR('',#37571,10.);
#11505=VECTOR('',#37576,10.);
#11506=VECTOR('',#37577,10.);
#11507=VECTOR('',#37578,10.);
#11508=VECTOR('',#37579,10.);
#11509=VECTOR('',#37582,10.);
#11510=VECTOR('',#37583,10.);
#11511=VECTOR('',#37584,10.);
#11512=VECTOR('',#37587,10.);
#11513=VECTOR('',#37588,10.);
#11514=VECTOR('',#37589,10.);
#11515=VECTOR('',#37592,10.);
#11516=VECTOR('',#37593,10.);
#11517=VECTOR('',#37598,10.);
#11518=VECTOR('',#37599,10.);
#11519=VECTOR('',#37600,10.);
#11520=VECTOR('',#37601,10.);
#11521=VECTOR('',#37604,10.);
#11522=VECTOR('',#37605,10.);
#11523=VECTOR('',#37606,10.);
#11524=VECTOR('',#37609,10.);
#11525=VECTOR('',#37610,10.);
#11526=VECTOR('',#37611,10.);
#11527=VECTOR('',#37614,10.);
#11528=VECTOR('',#37615,10.);
#11529=VECTOR('',#37620,10.);
#11530=VECTOR('',#37621,10.);
#11531=VECTOR('',#37622,10.);
#11532=VECTOR('',#37623,10.);
#11533=VECTOR('',#37626,10.);
#11534=VECTOR('',#37627,10.);
#11535=VECTOR('',#37628,10.);
#11536=VECTOR('',#37631,10.);
#11537=VECTOR('',#37632,10.);
#11538=VECTOR('',#37633,10.);
#11539=VECTOR('',#37636,10.);
#11540=VECTOR('',#37637,10.);
#11541=VECTOR('',#37642,10.);
#11542=VECTOR('',#37643,10.);
#11543=VECTOR('',#37644,10.);
#11544=VECTOR('',#37645,10.);
#11545=VECTOR('',#37648,10.);
#11546=VECTOR('',#37649,10.);
#11547=VECTOR('',#37650,10.);
#11548=VECTOR('',#37653,10.);
#11549=VECTOR('',#37654,10.);
#11550=VECTOR('',#37655,10.);
#11551=VECTOR('',#37658,10.);
#11552=VECTOR('',#37659,10.);
#11553=VECTOR('',#37664,10.);
#11554=VECTOR('',#37665,10.);
#11555=VECTOR('',#37666,10.);
#11556=VECTOR('',#37667,10.);
#11557=VECTOR('',#37670,10.);
#11558=VECTOR('',#37671,10.);
#11559=VECTOR('',#37672,10.);
#11560=VECTOR('',#37675,10.);
#11561=VECTOR('',#37676,10.);
#11562=VECTOR('',#37677,10.);
#11563=VECTOR('',#37680,10.);
#11564=VECTOR('',#37681,10.);
#11565=VECTOR('',#37686,10.);
#11566=VECTOR('',#37687,10.);
#11567=VECTOR('',#37688,10.);
#11568=VECTOR('',#37689,10.);
#11569=VECTOR('',#37692,10.);
#11570=VECTOR('',#37693,10.);
#11571=VECTOR('',#37694,10.);
#11572=VECTOR('',#37697,10.);
#11573=VECTOR('',#37698,10.);
#11574=VECTOR('',#37699,10.);
#11575=VECTOR('',#37702,10.);
#11576=VECTOR('',#37703,10.);
#11577=VECTOR('',#37708,10.);
#11578=VECTOR('',#37709,10.);
#11579=VECTOR('',#37710,10.);
#11580=VECTOR('',#37711,10.);
#11581=VECTOR('',#37714,10.);
#11582=VECTOR('',#37715,10.);
#11583=VECTOR('',#37716,10.);
#11584=VECTOR('',#37719,10.);
#11585=VECTOR('',#37720,10.);
#11586=VECTOR('',#37721,10.);
#11587=VECTOR('',#37724,10.);
#11588=VECTOR('',#37725,10.);
#11589=VECTOR('',#37730,10.);
#11590=VECTOR('',#37731,10.);
#11591=VECTOR('',#37732,10.);
#11592=VECTOR('',#37733,10.);
#11593=VECTOR('',#37736,10.);
#11594=VECTOR('',#37737,10.);
#11595=VECTOR('',#37738,10.);
#11596=VECTOR('',#37741,10.);
#11597=VECTOR('',#37742,10.);
#11598=VECTOR('',#37743,10.);
#11599=VECTOR('',#37746,10.);
#11600=VECTOR('',#37747,10.);
#11601=VECTOR('',#37752,10.);
#11602=VECTOR('',#37753,10.);
#11603=VECTOR('',#37754,10.);
#11604=VECTOR('',#37755,10.);
#11605=VECTOR('',#37758,10.);
#11606=VECTOR('',#37759,10.);
#11607=VECTOR('',#37760,10.);
#11608=VECTOR('',#37763,10.);
#11609=VECTOR('',#37764,10.);
#11610=VECTOR('',#37765,10.);
#11611=VECTOR('',#37768,10.);
#11612=VECTOR('',#37769,10.);
#11613=VECTOR('',#37774,10.);
#11614=VECTOR('',#37775,10.);
#11615=VECTOR('',#37776,10.);
#11616=VECTOR('',#37777,10.);
#11617=VECTOR('',#37780,10.);
#11618=VECTOR('',#37781,10.);
#11619=VECTOR('',#37782,10.);
#11620=VECTOR('',#37785,10.);
#11621=VECTOR('',#37786,10.);
#11622=VECTOR('',#37787,10.);
#11623=VECTOR('',#37790,10.);
#11624=VECTOR('',#37791,10.);
#11625=VECTOR('',#37796,10.);
#11626=VECTOR('',#37797,10.);
#11627=VECTOR('',#37798,10.);
#11628=VECTOR('',#37799,10.);
#11629=VECTOR('',#37802,10.);
#11630=VECTOR('',#37803,10.);
#11631=VECTOR('',#37804,10.);
#11632=VECTOR('',#37807,10.);
#11633=VECTOR('',#37808,10.);
#11634=VECTOR('',#37809,10.);
#11635=VECTOR('',#37812,10.);
#11636=VECTOR('',#37813,10.);
#11637=VECTOR('',#37818,10.);
#11638=VECTOR('',#37819,10.);
#11639=VECTOR('',#37820,10.);
#11640=VECTOR('',#37821,10.);
#11641=VECTOR('',#37824,10.);
#11642=VECTOR('',#37825,10.);
#11643=VECTOR('',#37826,10.);
#11644=VECTOR('',#37829,10.);
#11645=VECTOR('',#37830,10.);
#11646=VECTOR('',#37831,10.);
#11647=VECTOR('',#37834,10.);
#11648=VECTOR('',#37835,10.);
#11649=VECTOR('',#37840,10.);
#11650=VECTOR('',#37841,10.);
#11651=VECTOR('',#37842,10.);
#11652=VECTOR('',#37843,10.);
#11653=VECTOR('',#37846,10.);
#11654=VECTOR('',#37847,10.);
#11655=VECTOR('',#37848,10.);
#11656=VECTOR('',#37851,10.);
#11657=VECTOR('',#37852,10.);
#11658=VECTOR('',#37853,10.);
#11659=VECTOR('',#37856,10.);
#11660=VECTOR('',#37857,10.);
#11661=VECTOR('',#37862,10.);
#11662=VECTOR('',#37863,10.);
#11663=VECTOR('',#37864,10.);
#11664=VECTOR('',#37865,10.);
#11665=VECTOR('',#37868,10.);
#11666=VECTOR('',#37869,10.);
#11667=VECTOR('',#37870,10.);
#11668=VECTOR('',#37873,10.);
#11669=VECTOR('',#37874,10.);
#11670=VECTOR('',#37875,10.);
#11671=VECTOR('',#37878,10.);
#11672=VECTOR('',#37879,10.);
#11673=VECTOR('',#37884,10.);
#11674=VECTOR('',#37885,10.);
#11675=VECTOR('',#37886,10.);
#11676=VECTOR('',#37887,10.);
#11677=VECTOR('',#37890,10.);
#11678=VECTOR('',#37891,10.);
#11679=VECTOR('',#37892,10.);
#11680=VECTOR('',#37895,10.);
#11681=VECTOR('',#37896,10.);
#11682=VECTOR('',#37897,10.);
#11683=VECTOR('',#37900,10.);
#11684=VECTOR('',#37901,10.);
#11685=VECTOR('',#37906,10.);
#11686=VECTOR('',#37907,10.);
#11687=VECTOR('',#37908,10.);
#11688=VECTOR('',#37909,10.);
#11689=VECTOR('',#37912,10.);
#11690=VECTOR('',#37913,10.);
#11691=VECTOR('',#37914,10.);
#11692=VECTOR('',#37917,10.);
#11693=VECTOR('',#37918,10.);
#11694=VECTOR('',#37919,10.);
#11695=VECTOR('',#37922,10.);
#11696=VECTOR('',#37923,10.);
#11697=VECTOR('',#37928,10.);
#11698=VECTOR('',#37929,10.);
#11699=VECTOR('',#37930,10.);
#11700=VECTOR('',#37931,10.);
#11701=VECTOR('',#37934,10.);
#11702=VECTOR('',#37935,10.);
#11703=VECTOR('',#37936,10.);
#11704=VECTOR('',#37939,10.);
#11705=VECTOR('',#37940,10.);
#11706=VECTOR('',#37941,10.);
#11707=VECTOR('',#37944,10.);
#11708=VECTOR('',#37945,10.);
#11709=VECTOR('',#37950,10.);
#11710=VECTOR('',#37951,10.);
#11711=VECTOR('',#37952,10.);
#11712=VECTOR('',#37953,10.);
#11713=VECTOR('',#37956,10.);
#11714=VECTOR('',#37957,10.);
#11715=VECTOR('',#37958,10.);
#11716=VECTOR('',#37961,10.);
#11717=VECTOR('',#37962,10.);
#11718=VECTOR('',#37963,10.);
#11719=VECTOR('',#37966,10.);
#11720=VECTOR('',#37967,10.);
#11721=VECTOR('',#37972,10.);
#11722=VECTOR('',#37973,10.);
#11723=VECTOR('',#37974,10.);
#11724=VECTOR('',#37975,10.);
#11725=VECTOR('',#37978,10.);
#11726=VECTOR('',#37979,10.);
#11727=VECTOR('',#37980,10.);
#11728=VECTOR('',#37983,10.);
#11729=VECTOR('',#37984,10.);
#11730=VECTOR('',#37985,10.);
#11731=VECTOR('',#37988,10.);
#11732=VECTOR('',#37989,10.);
#11733=VECTOR('',#37994,10.);
#11734=VECTOR('',#37995,10.);
#11735=VECTOR('',#37996,10.);
#11736=VECTOR('',#37997,10.);
#11737=VECTOR('',#38000,10.);
#11738=VECTOR('',#38001,10.);
#11739=VECTOR('',#38002,10.);
#11740=VECTOR('',#38005,10.);
#11741=VECTOR('',#38006,10.);
#11742=VECTOR('',#38007,10.);
#11743=VECTOR('',#38010,10.);
#11744=VECTOR('',#38011,10.);
#11745=VECTOR('',#38016,10.);
#11746=VECTOR('',#38017,10.);
#11747=VECTOR('',#38018,10.);
#11748=VECTOR('',#38019,10.);
#11749=VECTOR('',#38022,10.);
#11750=VECTOR('',#38023,10.);
#11751=VECTOR('',#38024,10.);
#11752=VECTOR('',#38027,10.);
#11753=VECTOR('',#38028,10.);
#11754=VECTOR('',#38029,10.);
#11755=VECTOR('',#38032,10.);
#11756=VECTOR('',#38033,10.);
#11757=VECTOR('',#38038,10.);
#11758=VECTOR('',#38039,10.);
#11759=VECTOR('',#38040,10.);
#11760=VECTOR('',#38041,10.);
#11761=VECTOR('',#38044,10.);
#11762=VECTOR('',#38045,10.);
#11763=VECTOR('',#38046,10.);
#11764=VECTOR('',#38049,10.);
#11765=VECTOR('',#38050,10.);
#11766=VECTOR('',#38051,10.);
#11767=VECTOR('',#38054,10.);
#11768=VECTOR('',#38055,10.);
#11769=VECTOR('',#38060,10.);
#11770=VECTOR('',#38061,10.);
#11771=VECTOR('',#38062,10.);
#11772=VECTOR('',#38063,10.);
#11773=VECTOR('',#38066,10.);
#11774=VECTOR('',#38067,10.);
#11775=VECTOR('',#38068,10.);
#11776=VECTOR('',#38071,10.);
#11777=VECTOR('',#38072,10.);
#11778=VECTOR('',#38073,10.);
#11779=VECTOR('',#38076,10.);
#11780=VECTOR('',#38077,10.);
#11781=VECTOR('',#38082,10.);
#11782=VECTOR('',#38083,10.);
#11783=VECTOR('',#38084,10.);
#11784=VECTOR('',#38085,10.);
#11785=VECTOR('',#38088,10.);
#11786=VECTOR('',#38089,10.);
#11787=VECTOR('',#38090,10.);
#11788=VECTOR('',#38093,10.);
#11789=VECTOR('',#38094,10.);
#11790=VECTOR('',#38095,10.);
#11791=VECTOR('',#38098,10.);
#11792=VECTOR('',#38099,10.);
#11793=VECTOR('',#38104,10.);
#11794=VECTOR('',#38105,10.);
#11795=VECTOR('',#38106,10.);
#11796=VECTOR('',#38107,10.);
#11797=VECTOR('',#38110,10.);
#11798=VECTOR('',#38111,10.);
#11799=VECTOR('',#38112,10.);
#11800=VECTOR('',#38115,10.);
#11801=VECTOR('',#38116,10.);
#11802=VECTOR('',#38117,10.);
#11803=VECTOR('',#38120,10.);
#11804=VECTOR('',#38121,10.);
#11805=VECTOR('',#38126,10.);
#11806=VECTOR('',#38127,10.);
#11807=VECTOR('',#38128,10.);
#11808=VECTOR('',#38129,10.);
#11809=VECTOR('',#38132,10.);
#11810=VECTOR('',#38133,10.);
#11811=VECTOR('',#38134,10.);
#11812=VECTOR('',#38137,10.);
#11813=VECTOR('',#38138,10.);
#11814=VECTOR('',#38139,10.);
#11815=VECTOR('',#38142,10.);
#11816=VECTOR('',#38143,10.);
#11817=VECTOR('',#38148,10.);
#11818=VECTOR('',#38149,10.);
#11819=VECTOR('',#38150,10.);
#11820=VECTOR('',#38151,10.);
#11821=VECTOR('',#38154,10.);
#11822=VECTOR('',#38155,10.);
#11823=VECTOR('',#38156,10.);
#11824=VECTOR('',#38159,10.);
#11825=VECTOR('',#38160,10.);
#11826=VECTOR('',#38161,10.);
#11827=VECTOR('',#38164,10.);
#11828=VECTOR('',#38165,10.);
#11829=VECTOR('',#38170,10.);
#11830=VECTOR('',#38171,10.);
#11831=VECTOR('',#38172,10.);
#11832=VECTOR('',#38173,10.);
#11833=VECTOR('',#38176,10.);
#11834=VECTOR('',#38177,10.);
#11835=VECTOR('',#38178,10.);
#11836=VECTOR('',#38181,10.);
#11837=VECTOR('',#38182,10.);
#11838=VECTOR('',#38183,10.);
#11839=VECTOR('',#38186,10.);
#11840=VECTOR('',#38187,10.);
#11841=VECTOR('',#38192,10.);
#11842=VECTOR('',#38193,10.);
#11843=VECTOR('',#38194,10.);
#11844=VECTOR('',#38195,10.);
#11845=VECTOR('',#38198,10.);
#11846=VECTOR('',#38199,10.);
#11847=VECTOR('',#38200,10.);
#11848=VECTOR('',#38203,10.);
#11849=VECTOR('',#38204,10.);
#11850=VECTOR('',#38205,10.);
#11851=VECTOR('',#38208,10.);
#11852=VECTOR('',#38209,10.);
#11853=VECTOR('',#38214,10.);
#11854=VECTOR('',#38215,10.);
#11855=VECTOR('',#38216,10.);
#11856=VECTOR('',#38217,10.);
#11857=VECTOR('',#38220,10.);
#11858=VECTOR('',#38221,10.);
#11859=VECTOR('',#38222,10.);
#11860=VECTOR('',#38225,10.);
#11861=VECTOR('',#38226,10.);
#11862=VECTOR('',#38227,10.);
#11863=VECTOR('',#38230,10.);
#11864=VECTOR('',#38231,10.);
#11865=VECTOR('',#38236,10.);
#11866=VECTOR('',#38237,10.);
#11867=VECTOR('',#38238,10.);
#11868=VECTOR('',#38239,10.);
#11869=VECTOR('',#38242,10.);
#11870=VECTOR('',#38243,10.);
#11871=VECTOR('',#38244,10.);
#11872=VECTOR('',#38247,10.);
#11873=VECTOR('',#38248,10.);
#11874=VECTOR('',#38249,10.);
#11875=VECTOR('',#38252,10.);
#11876=VECTOR('',#38253,10.);
#11877=VECTOR('',#38260,1.1);
#11878=VECTOR('',#38267,1.1);
#11879=VECTOR('',#38272,10.);
#11880=VECTOR('',#38273,10.);
#11881=VECTOR('',#38274,10.);
#11882=VECTOR('',#38275,10.);
#11883=VECTOR('',#38282,10.);
#11884=VECTOR('',#38285,10.);
#11885=VECTOR('',#38286,10.);
#11886=VECTOR('',#38287,10.);
#11887=VECTOR('',#38294,10.);
#11888=VECTOR('',#38297,10.);
#11889=VECTOR('',#38298,10.);
#11890=VECTOR('',#38299,10.);
#11891=VECTOR('',#38306,10.);
#11892=VECTOR('',#38309,10.);
#11893=VECTOR('',#38310,10.);
#11894=VECTOR('',#38311,10.);
#12916=CIRCLE('',#33264,1.1);
#12917=CIRCLE('',#33265,1.1);
#12918=CIRCLE('',#33267,1.1);
#12919=CIRCLE('',#33268,1.1);
#12920=CIRCLE('',#33271,0.799999999999998);
#12921=CIRCLE('',#33272,0.799999999999998);
#12922=CIRCLE('',#33275,0.800000000000018);
#12923=CIRCLE('',#33276,0.800000000000018);
#12924=CIRCLE('',#33279,0.800000000000025);
#12925=CIRCLE('',#33280,0.800000000000025);
#12926=CIRCLE('',#33283,0.799999999999996);
#12927=CIRCLE('',#33284,0.799999999999996);
#13849=VERTEX_POINT('',#69957);
#13850=VERTEX_POINT('',#69958);
#13851=VERTEX_POINT('',#69962);
#13852=VERTEX_POINT('',#69964);
#13853=VERTEX_POINT('',#69975);
#13854=VERTEX_POINT('',#69979);
#13855=VERTEX_POINT('',#69990);
#13856=VERTEX_POINT('',#69994);
#13857=VERTEX_POINT('',#70005);
#13858=VERTEX_POINT('',#70009);
#13859=VERTEX_POINT('',#70020);
#13860=VERTEX_POINT('',#70024);
#13861=VERTEX_POINT('',#70035);
#13862=VERTEX_POINT('',#70039);
#13863=VERTEX_POINT('',#70050);
#13864=VERTEX_POINT('',#70054);
#13865=VERTEX_POINT('',#70077);
#13866=VERTEX_POINT('',#70078);
#13867=VERTEX_POINT('',#70082);
#13868=VERTEX_POINT('',#70084);
#13869=VERTEX_POINT('',#70095);
#13870=VERTEX_POINT('',#70099);
#13871=VERTEX_POINT('',#70110);
#13872=VERTEX_POINT('',#70114);
#13873=VERTEX_POINT('',#70125);
#13874=VERTEX_POINT('',#70129);
#13875=VERTEX_POINT('',#70140);
#13876=VERTEX_POINT('',#70144);
#13877=VERTEX_POINT('',#70155);
#13878=VERTEX_POINT('',#70159);
#13879=VERTEX_POINT('',#70170);
#13880=VERTEX_POINT('',#70174);
#13881=VERTEX_POINT('',#70185);
#13882=VERTEX_POINT('',#70189);
#13883=VERTEX_POINT('',#70200);
#13884=VERTEX_POINT('',#70204);
#13885=VERTEX_POINT('',#70215);
#13886=VERTEX_POINT('',#70219);
#13887=VERTEX_POINT('',#70230);
#13888=VERTEX_POINT('',#70234);
#13889=VERTEX_POINT('',#70253);
#13890=VERTEX_POINT('',#70254);
#13891=VERTEX_POINT('',#70256);
#13892=VERTEX_POINT('',#70258);
#13893=VERTEX_POINT('',#70262);
#13894=VERTEX_POINT('',#70264);
#13895=VERTEX_POINT('',#70271);
#13896=VERTEX_POINT('',#70272);
#13897=VERTEX_POINT('',#70274);
#13898=VERTEX_POINT('',#70276);
#13899=VERTEX_POINT('',#70280);
#13900=VERTEX_POINT('',#70282);
#13901=VERTEX_POINT('',#70286);
#13902=VERTEX_POINT('',#70288);
#13903=VERTEX_POINT('',#70292);
#13904=VERTEX_POINT('',#70294);
#13905=VERTEX_POINT('',#70298);
#13906=VERTEX_POINT('',#70300);
#13907=VERTEX_POINT('',#70304);
#13908=VERTEX_POINT('',#70306);
#13909=VERTEX_POINT('',#70310);
#13910=VERTEX_POINT('',#70312);
#13911=VERTEX_POINT('',#70316);
#13912=VERTEX_POINT('',#70318);
#13913=VERTEX_POINT('',#70322);
#13914=VERTEX_POINT('',#70324);
#13915=VERTEX_POINT('',#70328);
#13916=VERTEX_POINT('',#70330);
#13917=VERTEX_POINT('',#70345);
#13918=VERTEX_POINT('',#70346);
#13919=VERTEX_POINT('',#70350);
#13920=VERTEX_POINT('',#70352);
#13921=VERTEX_POINT('',#70363);
#13922=VERTEX_POINT('',#70367);
#13923=VERTEX_POINT('',#70378);
#13924=VERTEX_POINT('',#70382);
#13925=VERTEX_POINT('',#70393);
#13926=VERTEX_POINT('',#70397);
#13927=VERTEX_POINT('',#70408);
#13928=VERTEX_POINT('',#70412);
#13929=VERTEX_POINT('',#70423);
#13930=VERTEX_POINT('',#70427);
#13931=VERTEX_POINT('',#70438);
#13932=VERTEX_POINT('',#70442);
#13933=VERTEX_POINT('',#70465);
#13934=VERTEX_POINT('',#70466);
#13935=VERTEX_POINT('',#70470);
#13936=VERTEX_POINT('',#70472);
#13937=VERTEX_POINT('',#70483);
#13938=VERTEX_POINT('',#70487);
#13939=VERTEX_POINT('',#70498);
#13940=VERTEX_POINT('',#70502);
#13941=VERTEX_POINT('',#70513);
#13942=VERTEX_POINT('',#70517);
#13943=VERTEX_POINT('',#70528);
#13944=VERTEX_POINT('',#70532);
#13945=VERTEX_POINT('',#70543);
#13946=VERTEX_POINT('',#70547);
#13947=VERTEX_POINT('',#70558);
#13948=VERTEX_POINT('',#70562);
#13949=VERTEX_POINT('',#70573);
#13950=VERTEX_POINT('',#70577);
#13951=VERTEX_POINT('',#70588);
#13952=VERTEX_POINT('',#70592);
#13953=VERTEX_POINT('',#70603);
#13954=VERTEX_POINT('',#70607);
#13955=VERTEX_POINT('',#70618);
#13956=VERTEX_POINT('',#70622);
#13957=VERTEX_POINT('',#70646);
#13958=VERTEX_POINT('',#70647);
#13959=VERTEX_POINT('',#70651);
#13960=VERTEX_POINT('',#70653);
#13961=VERTEX_POINT('',#70664);
#13962=VERTEX_POINT('',#70668);
#13963=VERTEX_POINT('',#70679);
#13964=VERTEX_POINT('',#70683);
#13965=VERTEX_POINT('',#70694);
#13966=VERTEX_POINT('',#70698);
#13967=VERTEX_POINT('',#70709);
#13968=VERTEX_POINT('',#70713);
#13969=VERTEX_POINT('',#70724);
#13970=VERTEX_POINT('',#70728);
#13971=VERTEX_POINT('',#70739);
#13972=VERTEX_POINT('',#70743);
#13973=VERTEX_POINT('',#70754);
#13974=VERTEX_POINT('',#70758);
#13975=VERTEX_POINT('',#70769);
#13976=VERTEX_POINT('',#70773);
#13977=VERTEX_POINT('',#70784);
#13978=VERTEX_POINT('',#70788);
#13979=VERTEX_POINT('',#70799);
#13980=VERTEX_POINT('',#70803);
#13981=VERTEX_POINT('',#70814);
#13982=VERTEX_POINT('',#70818);
#13983=VERTEX_POINT('',#70824);
#13984=VERTEX_POINT('',#70826);
#13985=VERTEX_POINT('',#70835);
#13986=VERTEX_POINT('',#70839);
#13987=VERTEX_POINT('',#70850);
#13988=VERTEX_POINT('',#70854);
#13989=VERTEX_POINT('',#70865);
#13990=VERTEX_POINT('',#70869);
#13991=VERTEX_POINT('',#70880);
#13992=VERTEX_POINT('',#70884);
#13993=VERTEX_POINT('',#70895);
#13994=VERTEX_POINT('',#70899);
#13995=VERTEX_POINT('',#70910);
#13996=VERTEX_POINT('',#70914);
#13997=VERTEX_POINT('',#70925);
#13998=VERTEX_POINT('',#70929);
#13999=VERTEX_POINT('',#70935);
#14000=VERTEX_POINT('',#70937);
#14001=VERTEX_POINT('',#70946);
#14002=VERTEX_POINT('',#70950);
#14003=VERTEX_POINT('',#70961);
#14004=VERTEX_POINT('',#70965);
#14005=VERTEX_POINT('',#70976);
#14006=VERTEX_POINT('',#70980);
#14007=VERTEX_POINT('',#70991);
#14008=VERTEX_POINT('',#70995);
#14009=VERTEX_POINT('',#71006);
#14010=VERTEX_POINT('',#71010);
#14011=VERTEX_POINT('',#71021);
#14012=VERTEX_POINT('',#71025);
#14013=VERTEX_POINT('',#71036);
#14014=VERTEX_POINT('',#71040);
#14015=VERTEX_POINT('',#71046);
#14016=VERTEX_POINT('',#71048);
#14017=VERTEX_POINT('',#71071);
#14018=VERTEX_POINT('',#71072);
#14019=VERTEX_POINT('',#71076);
#14020=VERTEX_POINT('',#71078);
#14021=VERTEX_POINT('',#71089);
#14022=VERTEX_POINT('',#71093);
#14023=VERTEX_POINT('',#71104);
#14024=VERTEX_POINT('',#71108);
#14025=VERTEX_POINT('',#71119);
#14026=VERTEX_POINT('',#71123);
#14027=VERTEX_POINT('',#71134);
#14028=VERTEX_POINT('',#71138);
#14029=VERTEX_POINT('',#71149);
#14030=VERTEX_POINT('',#71153);
#14031=VERTEX_POINT('',#71164);
#14032=VERTEX_POINT('',#71168);
#14033=VERTEX_POINT('',#71191);
#14034=VERTEX_POINT('',#71192);
#14035=VERTEX_POINT('',#71196);
#14036=VERTEX_POINT('',#71198);
#14037=VERTEX_POINT('',#71209);
#14038=VERTEX_POINT('',#71213);
#14039=VERTEX_POINT('',#71224);
#14040=VERTEX_POINT('',#71228);
#14041=VERTEX_POINT('',#71239);
#14042=VERTEX_POINT('',#71243);
#14043=VERTEX_POINT('',#71254);
#14044=VERTEX_POINT('',#71258);
#14045=VERTEX_POINT('',#71269);
#14046=VERTEX_POINT('',#71273);
#14047=VERTEX_POINT('',#71284);
#14048=VERTEX_POINT('',#71288);
#14049=VERTEX_POINT('',#71299);
#14050=VERTEX_POINT('',#71303);
#14051=VERTEX_POINT('',#71314);
#14052=VERTEX_POINT('',#71318);
#14053=VERTEX_POINT('',#71329);
#14054=VERTEX_POINT('',#71333);
#14055=VERTEX_POINT('',#71344);
#14056=VERTEX_POINT('',#71348);
#14057=VERTEX_POINT('',#71372);
#14058=VERTEX_POINT('',#71373);
#14059=VERTEX_POINT('',#71377);
#14060=VERTEX_POINT('',#71379);
#14061=VERTEX_POINT('',#71390);
#14062=VERTEX_POINT('',#71394);
#14063=VERTEX_POINT('',#71405);
#14064=VERTEX_POINT('',#71409);
#14065=VERTEX_POINT('',#71420);
#14066=VERTEX_POINT('',#71424);
#14067=VERTEX_POINT('',#71435);
#14068=VERTEX_POINT('',#71439);
#14069=VERTEX_POINT('',#71450);
#14070=VERTEX_POINT('',#71454);
#14071=VERTEX_POINT('',#71465);
#14072=VERTEX_POINT('',#71469);
#14073=VERTEX_POINT('',#71480);
#14074=VERTEX_POINT('',#71484);
#14075=VERTEX_POINT('',#71495);
#14076=VERTEX_POINT('',#71499);
#14077=VERTEX_POINT('',#71505);
#14078=VERTEX_POINT('',#71507);
#14079=VERTEX_POINT('',#71516);
#14080=VERTEX_POINT('',#71520);
#14081=VERTEX_POINT('',#71531);
#14082=VERTEX_POINT('',#71535);
#14083=VERTEX_POINT('',#71546);
#14084=VERTEX_POINT('',#71550);
#14085=VERTEX_POINT('',#71561);
#14086=VERTEX_POINT('',#71565);
#14087=VERTEX_POINT('',#71576);
#14088=VERTEX_POINT('',#71580);
#14089=VERTEX_POINT('',#71591);
#14090=VERTEX_POINT('',#71595);
#14091=VERTEX_POINT('',#71606);
#14092=VERTEX_POINT('',#71610);
#14093=VERTEX_POINT('',#71621);
#14094=VERTEX_POINT('',#71625);
#14095=VERTEX_POINT('',#71636);
#14096=VERTEX_POINT('',#71640);
#14097=VERTEX_POINT('',#71646);
#14098=VERTEX_POINT('',#71648);
#14099=VERTEX_POINT('',#71652);
#14100=VERTEX_POINT('',#71654);
#14101=VERTEX_POINT('',#71668);
#14102=VERTEX_POINT('',#71669);
#14103=VERTEX_POINT('',#71673);
#14104=VERTEX_POINT('',#71675);
#14105=VERTEX_POINT('',#71686);
#14106=VERTEX_POINT('',#71690);
#14107=VERTEX_POINT('',#71701);
#14108=VERTEX_POINT('',#71705);
#14109=VERTEX_POINT('',#71716);
#14110=VERTEX_POINT('',#71720);
#14111=VERTEX_POINT('',#71731);
#14112=VERTEX_POINT('',#71735);
#14113=VERTEX_POINT('',#71746);
#14114=VERTEX_POINT('',#71750);
#14115=VERTEX_POINT('',#71761);
#14116=VERTEX_POINT('',#71765);
#14117=VERTEX_POINT('',#71788);
#14118=VERTEX_POINT('',#71789);
#14119=VERTEX_POINT('',#71793);
#14120=VERTEX_POINT('',#71795);
#14121=VERTEX_POINT('',#71806);
#14122=VERTEX_POINT('',#71810);
#14123=VERTEX_POINT('',#71821);
#14124=VERTEX_POINT('',#71825);
#14125=VERTEX_POINT('',#71836);
#14126=VERTEX_POINT('',#71840);
#14127=VERTEX_POINT('',#71851);
#14128=VERTEX_POINT('',#71855);
#14129=VERTEX_POINT('',#71866);
#14130=VERTEX_POINT('',#71870);
#14131=VERTEX_POINT('',#71881);
#14132=VERTEX_POINT('',#71885);
#14133=VERTEX_POINT('',#71896);
#14134=VERTEX_POINT('',#71900);
#14135=VERTEX_POINT('',#71911);
#14136=VERTEX_POINT('',#71915);
#14137=VERTEX_POINT('',#71926);
#14138=VERTEX_POINT('',#71930);
#14139=VERTEX_POINT('',#71941);
#14140=VERTEX_POINT('',#71945);
#14141=VERTEX_POINT('',#71964);
#14142=VERTEX_POINT('',#71965);
#14143=VERTEX_POINT('',#71967);
#14144=VERTEX_POINT('',#71969);
#14145=VERTEX_POINT('',#71978);
#14146=VERTEX_POINT('',#71982);
#14147=VERTEX_POINT('',#71993);
#14148=VERTEX_POINT('',#71997);
#14149=VERTEX_POINT('',#72003);
#14150=VERTEX_POINT('',#72005);
#14151=VERTEX_POINT('',#72014);
#14152=VERTEX_POINT('',#72018);
#14153=VERTEX_POINT('',#72029);
#14154=VERTEX_POINT('',#72033);
#14155=VERTEX_POINT('',#72039);
#14156=VERTEX_POINT('',#72041);
#14157=VERTEX_POINT('',#72045);
#14158=VERTEX_POINT('',#72047);
#14159=VERTEX_POINT('',#72061);
#14160=VERTEX_POINT('',#72062);
#14161=VERTEX_POINT('',#72066);
#14162=VERTEX_POINT('',#72068);
#14163=VERTEX_POINT('',#72079);
#14164=VERTEX_POINT('',#72083);
#14165=VERTEX_POINT('',#72094);
#14166=VERTEX_POINT('',#72098);
#14167=VERTEX_POINT('',#72109);
#14168=VERTEX_POINT('',#72113);
#14169=VERTEX_POINT('',#72124);
#14170=VERTEX_POINT('',#72128);
#14171=VERTEX_POINT('',#72139);
#14172=VERTEX_POINT('',#72143);
#14173=VERTEX_POINT('',#72154);
#14174=VERTEX_POINT('',#72158);
#14175=VERTEX_POINT('',#72181);
#14176=VERTEX_POINT('',#72182);
#14177=VERTEX_POINT('',#72186);
#14178=VERTEX_POINT('',#72188);
#14179=VERTEX_POINT('',#72199);
#14180=VERTEX_POINT('',#72203);
#14181=VERTEX_POINT('',#72214);
#14182=VERTEX_POINT('',#72218);
#14183=VERTEX_POINT('',#72229);
#14184=VERTEX_POINT('',#72233);
#14185=VERTEX_POINT('',#72244);
#14186=VERTEX_POINT('',#72248);
#14187=VERTEX_POINT('',#72259);
#14188=VERTEX_POINT('',#72263);
#14189=VERTEX_POINT('',#72274);
#14190=VERTEX_POINT('',#72278);
#14191=VERTEX_POINT('',#72289);
#14192=VERTEX_POINT('',#72293);
#14193=VERTEX_POINT('',#72304);
#14194=VERTEX_POINT('',#72308);
#14195=VERTEX_POINT('',#72319);
#14196=VERTEX_POINT('',#72323);
#14197=VERTEX_POINT('',#72334);
#14198=VERTEX_POINT('',#72338);
#14199=VERTEX_POINT('',#72363);
#14200=VERTEX_POINT('',#72364);
#14201=VERTEX_POINT('',#72368);
#14202=VERTEX_POINT('',#72370);
#14203=VERTEX_POINT('',#72381);
#14204=VERTEX_POINT('',#72385);
#14205=VERTEX_POINT('',#72396);
#14206=VERTEX_POINT('',#72400);
#14207=VERTEX_POINT('',#72411);
#14208=VERTEX_POINT('',#72415);
#14209=VERTEX_POINT('',#72426);
#14210=VERTEX_POINT('',#72430);
#14211=VERTEX_POINT('',#72441);
#14212=VERTEX_POINT('',#72445);
#14213=VERTEX_POINT('',#72456);
#14214=VERTEX_POINT('',#72460);
#14215=VERTEX_POINT('',#72483);
#14216=VERTEX_POINT('',#72484);
#14217=VERTEX_POINT('',#72488);
#14218=VERTEX_POINT('',#72490);
#14219=VERTEX_POINT('',#72501);
#14220=VERTEX_POINT('',#72505);
#14221=VERTEX_POINT('',#72516);
#14222=VERTEX_POINT('',#72520);
#14223=VERTEX_POINT('',#72531);
#14224=VERTEX_POINT('',#72535);
#14225=VERTEX_POINT('',#72546);
#14226=VERTEX_POINT('',#72550);
#14227=VERTEX_POINT('',#72561);
#14228=VERTEX_POINT('',#72565);
#14229=VERTEX_POINT('',#72576);
#14230=VERTEX_POINT('',#72580);
#14231=VERTEX_POINT('',#72591);
#14232=VERTEX_POINT('',#72595);
#14233=VERTEX_POINT('',#72606);
#14234=VERTEX_POINT('',#72610);
#14235=VERTEX_POINT('',#72621);
#14236=VERTEX_POINT('',#72625);
#14237=VERTEX_POINT('',#72636);
#14238=VERTEX_POINT('',#72640);
#14239=VERTEX_POINT('',#72659);
#14240=VERTEX_POINT('',#72660);
#14241=VERTEX_POINT('',#72662);
#14242=VERTEX_POINT('',#72664);
#14243=VERTEX_POINT('',#72673);
#14244=VERTEX_POINT('',#72677);
#14245=VERTEX_POINT('',#72688);
#14246=VERTEX_POINT('',#72692);
#14247=VERTEX_POINT('',#72698);
#14248=VERTEX_POINT('',#72700);
#14249=VERTEX_POINT('',#72709);
#14250=VERTEX_POINT('',#72713);
#14251=VERTEX_POINT('',#72724);
#14252=VERTEX_POINT('',#72728);
#14253=VERTEX_POINT('',#72734);
#14254=VERTEX_POINT('',#72736);
#14255=VERTEX_POINT('',#72740);
#14256=VERTEX_POINT('',#72742);
#14257=VERTEX_POINT('',#72756);
#14258=VERTEX_POINT('',#72757);
#14259=VERTEX_POINT('',#72761);
#14260=VERTEX_POINT('',#72763);
#14261=VERTEX_POINT('',#72774);
#14262=VERTEX_POINT('',#72778);
#14263=VERTEX_POINT('',#72789);
#14264=VERTEX_POINT('',#72793);
#14265=VERTEX_POINT('',#72804);
#14266=VERTEX_POINT('',#72808);
#14267=VERTEX_POINT('',#72819);
#14268=VERTEX_POINT('',#72823);
#14269=VERTEX_POINT('',#72834);
#14270=VERTEX_POINT('',#72838);
#14271=VERTEX_POINT('',#72849);
#14272=VERTEX_POINT('',#72853);
#14273=VERTEX_POINT('',#72876);
#14274=VERTEX_POINT('',#72877);
#14275=VERTEX_POINT('',#72881);
#14276=VERTEX_POINT('',#72883);
#14277=VERTEX_POINT('',#72894);
#14278=VERTEX_POINT('',#72898);
#14279=VERTEX_POINT('',#72909);
#14280=VERTEX_POINT('',#72913);
#14281=VERTEX_POINT('',#72924);
#14282=VERTEX_POINT('',#72928);
#14283=VERTEX_POINT('',#72939);
#14284=VERTEX_POINT('',#72943);
#14285=VERTEX_POINT('',#72954);
#14286=VERTEX_POINT('',#72958);
#14287=VERTEX_POINT('',#72969);
#14288=VERTEX_POINT('',#72973);
#14289=VERTEX_POINT('',#72984);
#14290=VERTEX_POINT('',#72988);
#14291=VERTEX_POINT('',#72999);
#14292=VERTEX_POINT('',#73003);
#14293=VERTEX_POINT('',#73014);
#14294=VERTEX_POINT('',#73018);
#14295=VERTEX_POINT('',#73029);
#14296=VERTEX_POINT('',#73033);
#14297=VERTEX_POINT('',#73057);
#14298=VERTEX_POINT('',#73058);
#14299=VERTEX_POINT('',#73062);
#14300=VERTEX_POINT('',#73064);
#14301=VERTEX_POINT('',#73075);
#14302=VERTEX_POINT('',#73079);
#14303=VERTEX_POINT('',#73090);
#14304=VERTEX_POINT('',#73094);
#14305=VERTEX_POINT('',#73105);
#14306=VERTEX_POINT('',#73109);
#14307=VERTEX_POINT('',#73120);
#14308=VERTEX_POINT('',#73124);
#14309=VERTEX_POINT('',#73135);
#14310=VERTEX_POINT('',#73139);
#14311=VERTEX_POINT('',#73150);
#14312=VERTEX_POINT('',#73154);
#14313=VERTEX_POINT('',#73165);
#14314=VERTEX_POINT('',#73169);
#14315=VERTEX_POINT('',#73180);
#14316=VERTEX_POINT('',#73184);
#14317=VERTEX_POINT('',#73190);
#14318=VERTEX_POINT('',#73192);
#14319=VERTEX_POINT('',#73201);
#14320=VERTEX_POINT('',#73205);
#14321=VERTEX_POINT('',#73216);
#14322=VERTEX_POINT('',#73220);
#14323=VERTEX_POINT('',#73231);
#14324=VERTEX_POINT('',#73235);
#14325=VERTEX_POINT('',#73246);
#14326=VERTEX_POINT('',#73250);
#14327=VERTEX_POINT('',#73261);
#14328=VERTEX_POINT('',#73265);
#14329=VERTEX_POINT('',#73276);
#14330=VERTEX_POINT('',#73280);
#14331=VERTEX_POINT('',#73291);
#14332=VERTEX_POINT('',#73295);
#14333=VERTEX_POINT('',#73306);
#14334=VERTEX_POINT('',#73310);
#14335=VERTEX_POINT('',#73321);
#14336=VERTEX_POINT('',#73325);
#14337=VERTEX_POINT('',#73331);
#14338=VERTEX_POINT('',#73333);
#14339=VERTEX_POINT('',#73337);
#14340=VERTEX_POINT('',#73339);
#14341=VERTEX_POINT('',#73353);
#14342=VERTEX_POINT('',#73354);
#14343=VERTEX_POINT('',#73358);
#14344=VERTEX_POINT('',#73360);
#14345=VERTEX_POINT('',#73371);
#14346=VERTEX_POINT('',#73375);
#14347=VERTEX_POINT('',#73386);
#14348=VERTEX_POINT('',#73390);
#14349=VERTEX_POINT('',#73401);
#14350=VERTEX_POINT('',#73405);
#14351=VERTEX_POINT('',#73416);
#14352=VERTEX_POINT('',#73420);
#14353=VERTEX_POINT('',#73431);
#14354=VERTEX_POINT('',#73435);
#14355=VERTEX_POINT('',#73446);
#14356=VERTEX_POINT('',#73450);
#14357=VERTEX_POINT('',#73473);
#14358=VERTEX_POINT('',#73474);
#14359=VERTEX_POINT('',#73478);
#14360=VERTEX_POINT('',#73480);
#14361=VERTEX_POINT('',#73491);
#14362=VERTEX_POINT('',#73495);
#14363=VERTEX_POINT('',#73506);
#14364=VERTEX_POINT('',#73510);
#14365=VERTEX_POINT('',#73521);
#14366=VERTEX_POINT('',#73525);
#14367=VERTEX_POINT('',#73536);
#14368=VERTEX_POINT('',#73540);
#14369=VERTEX_POINT('',#73551);
#14370=VERTEX_POINT('',#73555);
#14371=VERTEX_POINT('',#73566);
#14372=VERTEX_POINT('',#73570);
#14373=VERTEX_POINT('',#73581);
#14374=VERTEX_POINT('',#73585);
#14375=VERTEX_POINT('',#73596);
#14376=VERTEX_POINT('',#73600);
#14377=VERTEX_POINT('',#73611);
#14378=VERTEX_POINT('',#73615);
#14379=VERTEX_POINT('',#73626);
#14380=VERTEX_POINT('',#73630);
#14381=VERTEX_POINT('',#73654);
#14382=VERTEX_POINT('',#73655);
#14383=VERTEX_POINT('',#73659);
#14384=VERTEX_POINT('',#73661);
#14385=VERTEX_POINT('',#73672);
#14386=VERTEX_POINT('',#73676);
#14387=VERTEX_POINT('',#73687);
#14388=VERTEX_POINT('',#73691);
#14389=VERTEX_POINT('',#73702);
#14390=VERTEX_POINT('',#73706);
#14391=VERTEX_POINT('',#73717);
#14392=VERTEX_POINT('',#73721);
#14393=VERTEX_POINT('',#73732);
#14394=VERTEX_POINT('',#73736);
#14395=VERTEX_POINT('',#73747);
#14396=VERTEX_POINT('',#73751);
#14397=VERTEX_POINT('',#73762);
#14398=VERTEX_POINT('',#73766);
#14399=VERTEX_POINT('',#73777);
#14400=VERTEX_POINT('',#73781);
#14401=VERTEX_POINT('',#73792);
#14402=VERTEX_POINT('',#73796);
#14403=VERTEX_POINT('',#73807);
#14404=VERTEX_POINT('',#73811);
#14405=VERTEX_POINT('',#73822);
#14406=VERTEX_POINT('',#73826);
#14407=VERTEX_POINT('',#73832);
#14408=VERTEX_POINT('',#73834);
#14409=VERTEX_POINT('',#73843);
#14410=VERTEX_POINT('',#73847);
#14411=VERTEX_POINT('',#73858);
#14412=VERTEX_POINT('',#73862);
#14413=VERTEX_POINT('',#73873);
#14414=VERTEX_POINT('',#73877);
#14415=VERTEX_POINT('',#73888);
#14416=VERTEX_POINT('',#73892);
#14417=VERTEX_POINT('',#73903);
#14418=VERTEX_POINT('',#73907);
#14419=VERTEX_POINT('',#73918);
#14420=VERTEX_POINT('',#73922);
#14421=VERTEX_POINT('',#73933);
#14422=VERTEX_POINT('',#73937);
#14423=VERTEX_POINT('',#73943);
#14424=VERTEX_POINT('',#73945);
#14425=VERTEX_POINT('',#73954);
#14426=VERTEX_POINT('',#73958);
#14427=VERTEX_POINT('',#73969);
#14428=VERTEX_POINT('',#73973);
#14429=VERTEX_POINT('',#73984);
#14430=VERTEX_POINT('',#73988);
#14431=VERTEX_POINT('',#73999);
#14432=VERTEX_POINT('',#74003);
#14433=VERTEX_POINT('',#74014);
#14434=VERTEX_POINT('',#74018);
#14435=VERTEX_POINT('',#74029);
#14436=VERTEX_POINT('',#74033);
#14437=VERTEX_POINT('',#74044);
#14438=VERTEX_POINT('',#74048);
#14439=VERTEX_POINT('',#74054);
#14440=VERTEX_POINT('',#74056);
#14441=VERTEX_POINT('',#74079);
#14442=VERTEX_POINT('',#74080);
#14443=VERTEX_POINT('',#74084);
#14444=VERTEX_POINT('',#74086);
#14445=VERTEX_POINT('',#74097);
#14446=VERTEX_POINT('',#74101);
#14447=VERTEX_POINT('',#74112);
#14448=VERTEX_POINT('',#74116);
#14449=VERTEX_POINT('',#74127);
#14450=VERTEX_POINT('',#74131);
#14451=VERTEX_POINT('',#74142);
#14452=VERTEX_POINT('',#74146);
#14453=VERTEX_POINT('',#74157);
#14454=VERTEX_POINT('',#74161);
#14455=VERTEX_POINT('',#74172);
#14456=VERTEX_POINT('',#74176);
#14457=VERTEX_POINT('',#74199);
#14458=VERTEX_POINT('',#74200);
#14459=VERTEX_POINT('',#74204);
#14460=VERTEX_POINT('',#74206);
#14461=VERTEX_POINT('',#74217);
#14462=VERTEX_POINT('',#74221);
#14463=VERTEX_POINT('',#74232);
#14464=VERTEX_POINT('',#74236);
#14465=VERTEX_POINT('',#74247);
#14466=VERTEX_POINT('',#74251);
#14467=VERTEX_POINT('',#74262);
#14468=VERTEX_POINT('',#74266);
#14469=VERTEX_POINT('',#74277);
#14470=VERTEX_POINT('',#74281);
#14471=VERTEX_POINT('',#74292);
#14472=VERTEX_POINT('',#74296);
#14473=VERTEX_POINT('',#74307);
#14474=VERTEX_POINT('',#74311);
#14475=VERTEX_POINT('',#74322);
#14476=VERTEX_POINT('',#74326);
#14477=VERTEX_POINT('',#74337);
#14478=VERTEX_POINT('',#74341);
#14479=VERTEX_POINT('',#74352);
#14480=VERTEX_POINT('',#74356);
#14481=VERTEX_POINT('',#74375);
#14482=VERTEX_POINT('',#74376);
#14483=VERTEX_POINT('',#74378);
#14484=VERTEX_POINT('',#74380);
#14485=VERTEX_POINT('',#74384);
#14486=VERTEX_POINT('',#74386);
#14487=VERTEX_POINT('',#74393);
#14488=VERTEX_POINT('',#74394);
#14489=VERTEX_POINT('',#74396);
#14490=VERTEX_POINT('',#74398);
#14491=VERTEX_POINT('',#74402);
#14492=VERTEX_POINT('',#74404);
#14493=VERTEX_POINT('',#74408);
#14494=VERTEX_POINT('',#74410);
#14495=VERTEX_POINT('',#74414);
#14496=VERTEX_POINT('',#74416);
#14497=VERTEX_POINT('',#74420);
#14498=VERTEX_POINT('',#74422);
#14499=VERTEX_POINT('',#74426);
#14500=VERTEX_POINT('',#74428);
#14501=VERTEX_POINT('',#74432);
#14502=VERTEX_POINT('',#74434);
#14503=VERTEX_POINT('',#74438);
#14504=VERTEX_POINT('',#74440);
#14505=VERTEX_POINT('',#74444);
#14506=VERTEX_POINT('',#74446);
#14507=VERTEX_POINT('',#74450);
#14508=VERTEX_POINT('',#74452);
#14509=VERTEX_POINT('',#74462);
#14510=VERTEX_POINT('',#74463);
#14511=VERTEX_POINT('',#74465);
#14512=VERTEX_POINT('',#74467);
#14513=VERTEX_POINT('',#74471);
#14514=VERTEX_POINT('',#74473);
#14515=VERTEX_POINT('',#74477);
#14516=VERTEX_POINT('',#74479);
#14517=VERTEX_POINT('',#74487);
#14518=VERTEX_POINT('',#74488);
#14519=VERTEX_POINT('',#74490);
#14520=VERTEX_POINT('',#74492);
#14521=VERTEX_POINT('',#74496);
#14522=VERTEX_POINT('',#74498);
#14523=VERTEX_POINT('',#74502);
#14524=VERTEX_POINT('',#74504);
#14525=VERTEX_POINT('',#74512);
#14526=VERTEX_POINT('',#74513);
#14527=VERTEX_POINT('',#74515);
#14528=VERTEX_POINT('',#74517);
#14529=VERTEX_POINT('',#74521);
#14530=VERTEX_POINT('',#74523);
#14531=VERTEX_POINT('',#74527);
#14532=VERTEX_POINT('',#74529);
#14533=VERTEX_POINT('',#74537);
#14534=VERTEX_POINT('',#74538);
#14535=VERTEX_POINT('',#74540);
#14536=VERTEX_POINT('',#74542);
#14537=VERTEX_POINT('',#74546);
#14538=VERTEX_POINT('',#74548);
#14539=VERTEX_POINT('',#74552);
#14540=VERTEX_POINT('',#74554);
#14541=VERTEX_POINT('',#74562);
#14542=VERTEX_POINT('',#74563);
#14543=VERTEX_POINT('',#74565);
#14544=VERTEX_POINT('',#74567);
#14545=VERTEX_POINT('',#74571);
#14546=VERTEX_POINT('',#74573);
#14547=VERTEX_POINT('',#74577);
#14548=VERTEX_POINT('',#74579);
#14549=VERTEX_POINT('',#74587);
#14550=VERTEX_POINT('',#74588);
#14551=VERTEX_POINT('',#74590);
#14552=VERTEX_POINT('',#74592);
#14553=VERTEX_POINT('',#74596);
#14554=VERTEX_POINT('',#74598);
#14555=VERTEX_POINT('',#74602);
#14556=VERTEX_POINT('',#74604);
#14557=VERTEX_POINT('',#74612);
#14558=VERTEX_POINT('',#74613);
#14559=VERTEX_POINT('',#74615);
#14560=VERTEX_POINT('',#74617);
#14561=VERTEX_POINT('',#74621);
#14562=VERTEX_POINT('',#74623);
#14563=VERTEX_POINT('',#74627);
#14564=VERTEX_POINT('',#74629);
#14565=VERTEX_POINT('',#74637);
#14566=VERTEX_POINT('',#74638);
#14567=VERTEX_POINT('',#74640);
#14568=VERTEX_POINT('',#74642);
#14569=VERTEX_POINT('',#74646);
#14570=VERTEX_POINT('',#74648);
#14571=VERTEX_POINT('',#74652);
#14572=VERTEX_POINT('',#74654);
#14573=VERTEX_POINT('',#74662);
#14574=VERTEX_POINT('',#74663);
#14575=VERTEX_POINT('',#74665);
#14576=VERTEX_POINT('',#74667);
#14577=VERTEX_POINT('',#74671);
#14578=VERTEX_POINT('',#74673);
#14579=VERTEX_POINT('',#74677);
#14580=VERTEX_POINT('',#74679);
#14581=VERTEX_POINT('',#74687);
#14582=VERTEX_POINT('',#74688);
#14583=VERTEX_POINT('',#74690);
#14584=VERTEX_POINT('',#74692);
#14585=VERTEX_POINT('',#74696);
#14586=VERTEX_POINT('',#74698);
#14587=VERTEX_POINT('',#74702);
#14588=VERTEX_POINT('',#74704);
#14589=VERTEX_POINT('',#74712);
#14590=VERTEX_POINT('',#74713);
#14591=VERTEX_POINT('',#74715);
#14592=VERTEX_POINT('',#74717);
#14593=VERTEX_POINT('',#74721);
#14594=VERTEX_POINT('',#74723);
#14595=VERTEX_POINT('',#74727);
#14596=VERTEX_POINT('',#74729);
#14597=VERTEX_POINT('',#74737);
#14598=VERTEX_POINT('',#74738);
#14599=VERTEX_POINT('',#74740);
#14600=VERTEX_POINT('',#74742);
#14601=VERTEX_POINT('',#74746);
#14602=VERTEX_POINT('',#74748);
#14603=VERTEX_POINT('',#74752);
#14604=VERTEX_POINT('',#74754);
#14605=VERTEX_POINT('',#74762);
#14606=VERTEX_POINT('',#74763);
#14607=VERTEX_POINT('',#74765);
#14608=VERTEX_POINT('',#74767);
#14609=VERTEX_POINT('',#74771);
#14610=VERTEX_POINT('',#74773);
#14611=VERTEX_POINT('',#74777);
#14612=VERTEX_POINT('',#74779);
#14613=VERTEX_POINT('',#74787);
#14614=VERTEX_POINT('',#74788);
#14615=VERTEX_POINT('',#74790);
#14616=VERTEX_POINT('',#74792);
#14617=VERTEX_POINT('',#74796);
#14618=VERTEX_POINT('',#74798);
#14619=VERTEX_POINT('',#74802);
#14620=VERTEX_POINT('',#74804);
#14621=VERTEX_POINT('',#74812);
#14622=VERTEX_POINT('',#74813);
#14623=VERTEX_POINT('',#74815);
#14624=VERTEX_POINT('',#74817);
#14625=VERTEX_POINT('',#74821);
#14626=VERTEX_POINT('',#74823);
#14627=VERTEX_POINT('',#74827);
#14628=VERTEX_POINT('',#74829);
#14629=VERTEX_POINT('',#74837);
#14630=VERTEX_POINT('',#74838);
#14631=VERTEX_POINT('',#74840);
#14632=VERTEX_POINT('',#74842);
#14633=VERTEX_POINT('',#74846);
#14634=VERTEX_POINT('',#74848);
#14635=VERTEX_POINT('',#74852);
#14636=VERTEX_POINT('',#74854);
#14637=VERTEX_POINT('',#74862);
#14638=VERTEX_POINT('',#74863);
#14639=VERTEX_POINT('',#74865);
#14640=VERTEX_POINT('',#74867);
#14641=VERTEX_POINT('',#74871);
#14642=VERTEX_POINT('',#74873);
#14643=VERTEX_POINT('',#74877);
#14644=VERTEX_POINT('',#74879);
#14645=VERTEX_POINT('',#74887);
#14646=VERTEX_POINT('',#74888);
#14647=VERTEX_POINT('',#74890);
#14648=VERTEX_POINT('',#74892);
#14649=VERTEX_POINT('',#74896);
#14650=VERTEX_POINT('',#74898);
#14651=VERTEX_POINT('',#74902);
#14652=VERTEX_POINT('',#74904);
#14653=VERTEX_POINT('',#74912);
#14654=VERTEX_POINT('',#74913);
#14655=VERTEX_POINT('',#74915);
#14656=VERTEX_POINT('',#74917);
#14657=VERTEX_POINT('',#74921);
#14658=VERTEX_POINT('',#74923);
#14659=VERTEX_POINT('',#74927);
#14660=VERTEX_POINT('',#74929);
#14661=VERTEX_POINT('',#74937);
#14662=VERTEX_POINT('',#74938);
#14663=VERTEX_POINT('',#74940);
#14664=VERTEX_POINT('',#74942);
#14665=VERTEX_POINT('',#74946);
#14666=VERTEX_POINT('',#74948);
#14667=VERTEX_POINT('',#74952);
#14668=VERTEX_POINT('',#74954);
#14669=VERTEX_POINT('',#74962);
#14670=VERTEX_POINT('',#74963);
#14671=VERTEX_POINT('',#74965);
#14672=VERTEX_POINT('',#74967);
#14673=VERTEX_POINT('',#74971);
#14674=VERTEX_POINT('',#74973);
#14675=VERTEX_POINT('',#74977);
#14676=VERTEX_POINT('',#74979);
#14677=VERTEX_POINT('',#74987);
#14678=VERTEX_POINT('',#74988);
#14679=VERTEX_POINT('',#74990);
#14680=VERTEX_POINT('',#74992);
#14681=VERTEX_POINT('',#74996);
#14682=VERTEX_POINT('',#74998);
#14683=VERTEX_POINT('',#75002);
#14684=VERTEX_POINT('',#75004);
#14685=VERTEX_POINT('',#75012);
#14686=VERTEX_POINT('',#75013);
#14687=VERTEX_POINT('',#75015);
#14688=VERTEX_POINT('',#75017);
#14689=VERTEX_POINT('',#75021);
#14690=VERTEX_POINT('',#75023);
#14691=VERTEX_POINT('',#75027);
#14692=VERTEX_POINT('',#75029);
#14693=VERTEX_POINT('',#75037);
#14694=VERTEX_POINT('',#75038);
#14695=VERTEX_POINT('',#75040);
#14696=VERTEX_POINT('',#75042);
#14697=VERTEX_POINT('',#75046);
#14698=VERTEX_POINT('',#75048);
#14699=VERTEX_POINT('',#75052);
#14700=VERTEX_POINT('',#75054);
#14701=VERTEX_POINT('',#75062);
#14702=VERTEX_POINT('',#75063);
#14703=VERTEX_POINT('',#75065);
#14704=VERTEX_POINT('',#75067);
#14705=VERTEX_POINT('',#75071);
#14706=VERTEX_POINT('',#75073);
#14707=VERTEX_POINT('',#75077);
#14708=VERTEX_POINT('',#75079);
#14709=VERTEX_POINT('',#75087);
#14710=VERTEX_POINT('',#75088);
#14711=VERTEX_POINT('',#75090);
#14712=VERTEX_POINT('',#75092);
#14713=VERTEX_POINT('',#75096);
#14714=VERTEX_POINT('',#75098);
#14715=VERTEX_POINT('',#75102);
#14716=VERTEX_POINT('',#75104);
#14717=VERTEX_POINT('',#75112);
#14718=VERTEX_POINT('',#75113);
#14719=VERTEX_POINT('',#75115);
#14720=VERTEX_POINT('',#75117);
#14721=VERTEX_POINT('',#75121);
#14722=VERTEX_POINT('',#75123);
#14723=VERTEX_POINT('',#75127);
#14724=VERTEX_POINT('',#75129);
#14725=VERTEX_POINT('',#75137);
#14726=VERTEX_POINT('',#75138);
#14727=VERTEX_POINT('',#75140);
#14728=VERTEX_POINT('',#75142);
#14729=VERTEX_POINT('',#75146);
#14730=VERTEX_POINT('',#75148);
#14731=VERTEX_POINT('',#75152);
#14732=VERTEX_POINT('',#75154);
#14733=VERTEX_POINT('',#75162);
#14734=VERTEX_POINT('',#75163);
#14735=VERTEX_POINT('',#75165);
#14736=VERTEX_POINT('',#75167);
#14737=VERTEX_POINT('',#75171);
#14738=VERTEX_POINT('',#75173);
#14739=VERTEX_POINT('',#75177);
#14740=VERTEX_POINT('',#75179);
#14741=VERTEX_POINT('',#75187);
#14742=VERTEX_POINT('',#75188);
#14743=VERTEX_POINT('',#75190);
#14744=VERTEX_POINT('',#75192);
#14745=VERTEX_POINT('',#75196);
#14746=VERTEX_POINT('',#75198);
#14747=VERTEX_POINT('',#75202);
#14748=VERTEX_POINT('',#75204);
#14749=VERTEX_POINT('',#75212);
#14750=VERTEX_POINT('',#75213);
#14751=VERTEX_POINT('',#75215);
#14752=VERTEX_POINT('',#75217);
#14753=VERTEX_POINT('',#75221);
#14754=VERTEX_POINT('',#75223);
#14755=VERTEX_POINT('',#75227);
#14756=VERTEX_POINT('',#75229);
#14757=VERTEX_POINT('',#75237);
#14758=VERTEX_POINT('',#75238);
#14759=VERTEX_POINT('',#75240);
#14760=VERTEX_POINT('',#75242);
#14761=VERTEX_POINT('',#75246);
#14762=VERTEX_POINT('',#75248);
#14763=VERTEX_POINT('',#75252);
#14764=VERTEX_POINT('',#75254);
#14765=VERTEX_POINT('',#75262);
#14766=VERTEX_POINT('',#75263);
#14767=VERTEX_POINT('',#75265);
#14768=VERTEX_POINT('',#75267);
#14769=VERTEX_POINT('',#75271);
#14770=VERTEX_POINT('',#75273);
#14771=VERTEX_POINT('',#75277);
#14772=VERTEX_POINT('',#75279);
#14773=VERTEX_POINT('',#75287);
#14774=VERTEX_POINT('',#75288);
#14775=VERTEX_POINT('',#75290);
#14776=VERTEX_POINT('',#75292);
#14777=VERTEX_POINT('',#75296);
#14778=VERTEX_POINT('',#75298);
#14779=VERTEX_POINT('',#75302);
#14780=VERTEX_POINT('',#75304);
#14781=VERTEX_POINT('',#75312);
#14782=VERTEX_POINT('',#75313);
#14783=VERTEX_POINT('',#75315);
#14784=VERTEX_POINT('',#75317);
#14785=VERTEX_POINT('',#75321);
#14786=VERTEX_POINT('',#75323);
#14787=VERTEX_POINT('',#75327);
#14788=VERTEX_POINT('',#75329);
#14789=VERTEX_POINT('',#75337);
#14790=VERTEX_POINT('',#75338);
#14791=VERTEX_POINT('',#75340);
#14792=VERTEX_POINT('',#75342);
#14793=VERTEX_POINT('',#75346);
#14794=VERTEX_POINT('',#75348);
#14795=VERTEX_POINT('',#75352);
#14796=VERTEX_POINT('',#75354);
#14797=VERTEX_POINT('',#75362);
#14798=VERTEX_POINT('',#75363);
#14799=VERTEX_POINT('',#75365);
#14800=VERTEX_POINT('',#75367);
#14801=VERTEX_POINT('',#75371);
#14802=VERTEX_POINT('',#75373);
#14803=VERTEX_POINT('',#75377);
#14804=VERTEX_POINT('',#75379);
#14805=VERTEX_POINT('',#75387);
#14806=VERTEX_POINT('',#75388);
#14807=VERTEX_POINT('',#75390);
#14808=VERTEX_POINT('',#75392);
#14809=VERTEX_POINT('',#75396);
#14810=VERTEX_POINT('',#75398);
#14811=VERTEX_POINT('',#75402);
#14812=VERTEX_POINT('',#75404);
#14813=VERTEX_POINT('',#75412);
#14814=VERTEX_POINT('',#75413);
#14815=VERTEX_POINT('',#75415);
#14816=VERTEX_POINT('',#75417);
#14817=VERTEX_POINT('',#75421);
#14818=VERTEX_POINT('',#75423);
#14819=VERTEX_POINT('',#75427);
#14820=VERTEX_POINT('',#75429);
#14821=VERTEX_POINT('',#75437);
#14822=VERTEX_POINT('',#75438);
#14823=VERTEX_POINT('',#75440);
#14824=VERTEX_POINT('',#75442);
#14825=VERTEX_POINT('',#75446);
#14826=VERTEX_POINT('',#75448);
#14827=VERTEX_POINT('',#75452);
#14828=VERTEX_POINT('',#75454);
#14829=VERTEX_POINT('',#75462);
#14830=VERTEX_POINT('',#75463);
#14831=VERTEX_POINT('',#75465);
#14832=VERTEX_POINT('',#75467);
#14833=VERTEX_POINT('',#75471);
#14834=VERTEX_POINT('',#75473);
#14835=VERTEX_POINT('',#75477);
#14836=VERTEX_POINT('',#75479);
#14837=VERTEX_POINT('',#75487);
#14838=VERTEX_POINT('',#75488);
#14839=VERTEX_POINT('',#75490);
#14840=VERTEX_POINT('',#75492);
#14841=VERTEX_POINT('',#75496);
#14842=VERTEX_POINT('',#75498);
#14843=VERTEX_POINT('',#75502);
#14844=VERTEX_POINT('',#75504);
#14845=VERTEX_POINT('',#75512);
#14846=VERTEX_POINT('',#75513);
#14847=VERTEX_POINT('',#75515);
#14848=VERTEX_POINT('',#75517);
#14849=VERTEX_POINT('',#75521);
#14850=VERTEX_POINT('',#75523);
#14851=VERTEX_POINT('',#75527);
#14852=VERTEX_POINT('',#75529);
#14853=VERTEX_POINT('',#75537);
#14854=VERTEX_POINT('',#75538);
#14855=VERTEX_POINT('',#75540);
#14856=VERTEX_POINT('',#75542);
#14857=VERTEX_POINT('',#75546);
#14858=VERTEX_POINT('',#75548);
#14859=VERTEX_POINT('',#75552);
#14860=VERTEX_POINT('',#75554);
#14861=VERTEX_POINT('',#75562);
#14862=VERTEX_POINT('',#75563);
#14863=VERTEX_POINT('',#75565);
#14864=VERTEX_POINT('',#75567);
#14865=VERTEX_POINT('',#75571);
#14866=VERTEX_POINT('',#75573);
#14867=VERTEX_POINT('',#75577);
#14868=VERTEX_POINT('',#75579);
#14869=VERTEX_POINT('',#75587);
#14870=VERTEX_POINT('',#75588);
#14871=VERTEX_POINT('',#75590);
#14872=VERTEX_POINT('',#75592);
#14873=VERTEX_POINT('',#75596);
#14874=VERTEX_POINT('',#75598);
#14875=VERTEX_POINT('',#75602);
#14876=VERTEX_POINT('',#75604);
#14877=VERTEX_POINT('',#75612);
#14878=VERTEX_POINT('',#75613);
#14879=VERTEX_POINT('',#75615);
#14880=VERTEX_POINT('',#75617);
#14881=VERTEX_POINT('',#75621);
#14882=VERTEX_POINT('',#75623);
#14883=VERTEX_POINT('',#75627);
#14884=VERTEX_POINT('',#75629);
#14885=VERTEX_POINT('',#75637);
#14886=VERTEX_POINT('',#75638);
#14887=VERTEX_POINT('',#75640);
#14888=VERTEX_POINT('',#75642);
#14889=VERTEX_POINT('',#75646);
#14890=VERTEX_POINT('',#75648);
#14891=VERTEX_POINT('',#75652);
#14892=VERTEX_POINT('',#75654);
#14893=VERTEX_POINT('',#75662);
#14894=VERTEX_POINT('',#75663);
#14895=VERTEX_POINT('',#75665);
#14896=VERTEX_POINT('',#75667);
#14897=VERTEX_POINT('',#75671);
#14898=VERTEX_POINT('',#75673);
#14899=VERTEX_POINT('',#75677);
#14900=VERTEX_POINT('',#75679);
#14901=VERTEX_POINT('',#75687);
#14902=VERTEX_POINT('',#75688);
#14903=VERTEX_POINT('',#75690);
#14904=VERTEX_POINT('',#75692);
#14905=VERTEX_POINT('',#75696);
#14906=VERTEX_POINT('',#75698);
#14907=VERTEX_POINT('',#75702);
#14908=VERTEX_POINT('',#75704);
#14909=VERTEX_POINT('',#75712);
#14910=VERTEX_POINT('',#75713);
#14911=VERTEX_POINT('',#75715);
#14912=VERTEX_POINT('',#75717);
#14913=VERTEX_POINT('',#75721);
#14914=VERTEX_POINT('',#75723);
#14915=VERTEX_POINT('',#75727);
#14916=VERTEX_POINT('',#75729);
#14917=VERTEX_POINT('',#75737);
#14918=VERTEX_POINT('',#75738);
#14919=VERTEX_POINT('',#75740);
#14920=VERTEX_POINT('',#75742);
#14921=VERTEX_POINT('',#75746);
#14922=VERTEX_POINT('',#75748);
#14923=VERTEX_POINT('',#75752);
#14924=VERTEX_POINT('',#75754);
#14925=VERTEX_POINT('',#75762);
#14926=VERTEX_POINT('',#75763);
#14927=VERTEX_POINT('',#75765);
#14928=VERTEX_POINT('',#75767);
#14929=VERTEX_POINT('',#75771);
#14930=VERTEX_POINT('',#75773);
#14931=VERTEX_POINT('',#75777);
#14932=VERTEX_POINT('',#75779);
#14933=VERTEX_POINT('',#75787);
#14934=VERTEX_POINT('',#75788);
#14935=VERTEX_POINT('',#75790);
#14936=VERTEX_POINT('',#75792);
#14937=VERTEX_POINT('',#75796);
#14938=VERTEX_POINT('',#75798);
#14939=VERTEX_POINT('',#75802);
#14940=VERTEX_POINT('',#75804);
#14941=VERTEX_POINT('',#75812);
#14942=VERTEX_POINT('',#75813);
#14943=VERTEX_POINT('',#75815);
#14944=VERTEX_POINT('',#75817);
#14945=VERTEX_POINT('',#75821);
#14946=VERTEX_POINT('',#75823);
#14947=VERTEX_POINT('',#75827);
#14948=VERTEX_POINT('',#75829);
#14949=VERTEX_POINT('',#75837);
#14950=VERTEX_POINT('',#75838);
#14951=VERTEX_POINT('',#75840);
#14952=VERTEX_POINT('',#75842);
#14953=VERTEX_POINT('',#75846);
#14954=VERTEX_POINT('',#75848);
#14955=VERTEX_POINT('',#75852);
#14956=VERTEX_POINT('',#75854);
#14957=VERTEX_POINT('',#75862);
#14958=VERTEX_POINT('',#75863);
#14959=VERTEX_POINT('',#75865);
#14960=VERTEX_POINT('',#75867);
#14961=VERTEX_POINT('',#75871);
#14962=VERTEX_POINT('',#75873);
#14963=VERTEX_POINT('',#75877);
#14964=VERTEX_POINT('',#75879);
#14965=VERTEX_POINT('',#75887);
#14966=VERTEX_POINT('',#75888);
#14967=VERTEX_POINT('',#75890);
#14968=VERTEX_POINT('',#75892);
#14969=VERTEX_POINT('',#75896);
#14970=VERTEX_POINT('',#75898);
#14971=VERTEX_POINT('',#75902);
#14972=VERTEX_POINT('',#75904);
#14973=VERTEX_POINT('',#75912);
#14974=VERTEX_POINT('',#75913);
#14975=VERTEX_POINT('',#75915);
#14976=VERTEX_POINT('',#75917);
#14977=VERTEX_POINT('',#75921);
#14978=VERTEX_POINT('',#75923);
#14979=VERTEX_POINT('',#75927);
#14980=VERTEX_POINT('',#75929);
#14981=VERTEX_POINT('',#75937);
#14982=VERTEX_POINT('',#75938);
#14983=VERTEX_POINT('',#75940);
#14984=VERTEX_POINT('',#75942);
#14985=VERTEX_POINT('',#75946);
#14986=VERTEX_POINT('',#75948);
#14987=VERTEX_POINT('',#75952);
#14988=VERTEX_POINT('',#75954);
#14989=VERTEX_POINT('',#75962);
#14990=VERTEX_POINT('',#75963);
#14991=VERTEX_POINT('',#75965);
#14992=VERTEX_POINT('',#75967);
#14993=VERTEX_POINT('',#75971);
#14994=VERTEX_POINT('',#75973);
#14995=VERTEX_POINT('',#75977);
#14996=VERTEX_POINT('',#75979);
#14997=VERTEX_POINT('',#75987);
#14998=VERTEX_POINT('',#75988);
#14999=VERTEX_POINT('',#75990);
#15000=VERTEX_POINT('',#75992);
#15001=VERTEX_POINT('',#75996);
#15002=VERTEX_POINT('',#75998);
#15003=VERTEX_POINT('',#76002);
#15004=VERTEX_POINT('',#76004);
#15005=VERTEX_POINT('',#76012);
#15006=VERTEX_POINT('',#76013);
#15007=VERTEX_POINT('',#76015);
#15008=VERTEX_POINT('',#76017);
#15009=VERTEX_POINT('',#76021);
#15010=VERTEX_POINT('',#76023);
#15011=VERTEX_POINT('',#76027);
#15012=VERTEX_POINT('',#76029);
#15013=VERTEX_POINT('',#76037);
#15014=VERTEX_POINT('',#76038);
#15015=VERTEX_POINT('',#76040);
#15016=VERTEX_POINT('',#76042);
#15017=VERTEX_POINT('',#76046);
#15018=VERTEX_POINT('',#76048);
#15019=VERTEX_POINT('',#76052);
#15020=VERTEX_POINT('',#76054);
#15021=VERTEX_POINT('',#76062);
#15022=VERTEX_POINT('',#76063);
#15023=VERTEX_POINT('',#76065);
#15024=VERTEX_POINT('',#76067);
#15025=VERTEX_POINT('',#76071);
#15026=VERTEX_POINT('',#76073);
#15027=VERTEX_POINT('',#76077);
#15028=VERTEX_POINT('',#76079);
#15029=VERTEX_POINT('',#76087);
#15030=VERTEX_POINT('',#76088);
#15031=VERTEX_POINT('',#76090);
#15032=VERTEX_POINT('',#76092);
#15033=VERTEX_POINT('',#76096);
#15034=VERTEX_POINT('',#76098);
#15035=VERTEX_POINT('',#76102);
#15036=VERTEX_POINT('',#76104);
#15037=VERTEX_POINT('',#76112);
#15038=VERTEX_POINT('',#76113);
#15039=VERTEX_POINT('',#76115);
#15040=VERTEX_POINT('',#76117);
#15041=VERTEX_POINT('',#76121);
#15042=VERTEX_POINT('',#76123);
#15043=VERTEX_POINT('',#76127);
#15044=VERTEX_POINT('',#76129);
#15045=VERTEX_POINT('',#76137);
#15046=VERTEX_POINT('',#76138);
#15047=VERTEX_POINT('',#76140);
#15048=VERTEX_POINT('',#76142);
#15049=VERTEX_POINT('',#76146);
#15050=VERTEX_POINT('',#76148);
#15051=VERTEX_POINT('',#76152);
#15052=VERTEX_POINT('',#76154);
#15053=VERTEX_POINT('',#76162);
#15054=VERTEX_POINT('',#76163);
#15055=VERTEX_POINT('',#76165);
#15056=VERTEX_POINT('',#76167);
#15057=VERTEX_POINT('',#76171);
#15058=VERTEX_POINT('',#76173);
#15059=VERTEX_POINT('',#76177);
#15060=VERTEX_POINT('',#76179);
#15061=VERTEX_POINT('',#76187);
#15062=VERTEX_POINT('',#76188);
#15063=VERTEX_POINT('',#76190);
#15064=VERTEX_POINT('',#76192);
#15065=VERTEX_POINT('',#76196);
#15066=VERTEX_POINT('',#76198);
#15067=VERTEX_POINT('',#76202);
#15068=VERTEX_POINT('',#76204);
#15069=VERTEX_POINT('',#76212);
#15070=VERTEX_POINT('',#76213);
#15071=VERTEX_POINT('',#76215);
#15072=VERTEX_POINT('',#76217);
#15073=VERTEX_POINT('',#76221);
#15074=VERTEX_POINT('',#76223);
#15075=VERTEX_POINT('',#76227);
#15076=VERTEX_POINT('',#76229);
#15077=VERTEX_POINT('',#76237);
#15078=VERTEX_POINT('',#76238);
#15079=VERTEX_POINT('',#76240);
#15080=VERTEX_POINT('',#76242);
#15081=VERTEX_POINT('',#76246);
#15082=VERTEX_POINT('',#76248);
#15083=VERTEX_POINT('',#76252);
#15084=VERTEX_POINT('',#76254);
#15085=VERTEX_POINT('',#76262);
#15086=VERTEX_POINT('',#76263);
#15087=VERTEX_POINT('',#76265);
#15088=VERTEX_POINT('',#76267);
#15089=VERTEX_POINT('',#76271);
#15090=VERTEX_POINT('',#76273);
#15091=VERTEX_POINT('',#76277);
#15092=VERTEX_POINT('',#76279);
#15093=VERTEX_POINT('',#76287);
#15094=VERTEX_POINT('',#76288);
#15095=VERTEX_POINT('',#76290);
#15096=VERTEX_POINT('',#76292);
#15097=VERTEX_POINT('',#76296);
#15098=VERTEX_POINT('',#76298);
#15099=VERTEX_POINT('',#76302);
#15100=VERTEX_POINT('',#76304);
#15101=VERTEX_POINT('',#76312);
#15102=VERTEX_POINT('',#76313);
#15103=VERTEX_POINT('',#76315);
#15104=VERTEX_POINT('',#76317);
#15105=VERTEX_POINT('',#76321);
#15106=VERTEX_POINT('',#76323);
#15107=VERTEX_POINT('',#76327);
#15108=VERTEX_POINT('',#76329);
#15109=VERTEX_POINT('',#76337);
#15110=VERTEX_POINT('',#76338);
#15111=VERTEX_POINT('',#76340);
#15112=VERTEX_POINT('',#76342);
#15113=VERTEX_POINT('',#76346);
#15114=VERTEX_POINT('',#76348);
#15115=VERTEX_POINT('',#76352);
#15116=VERTEX_POINT('',#76354);
#15117=VERTEX_POINT('',#76362);
#15118=VERTEX_POINT('',#76363);
#15119=VERTEX_POINT('',#76365);
#15120=VERTEX_POINT('',#76367);
#15121=VERTEX_POINT('',#76371);
#15122=VERTEX_POINT('',#76373);
#15123=VERTEX_POINT('',#76377);
#15124=VERTEX_POINT('',#76379);
#15125=VERTEX_POINT('',#76387);
#15126=VERTEX_POINT('',#76388);
#15127=VERTEX_POINT('',#76390);
#15128=VERTEX_POINT('',#76392);
#15129=VERTEX_POINT('',#76396);
#15130=VERTEX_POINT('',#76398);
#15131=VERTEX_POINT('',#76402);
#15132=VERTEX_POINT('',#76404);
#15133=VERTEX_POINT('',#76412);
#15134=VERTEX_POINT('',#76413);
#15135=VERTEX_POINT('',#76415);
#15136=VERTEX_POINT('',#76417);
#15137=VERTEX_POINT('',#76421);
#15138=VERTEX_POINT('',#76423);
#15139=VERTEX_POINT('',#76427);
#15140=VERTEX_POINT('',#76429);
#15141=VERTEX_POINT('',#76437);
#15142=VERTEX_POINT('',#76438);
#15143=VERTEX_POINT('',#76440);
#15144=VERTEX_POINT('',#76442);
#15145=VERTEX_POINT('',#76446);
#15146=VERTEX_POINT('',#76448);
#15147=VERTEX_POINT('',#76452);
#15148=VERTEX_POINT('',#76454);
#15149=VERTEX_POINT('',#76462);
#15150=VERTEX_POINT('',#76463);
#15151=VERTEX_POINT('',#76465);
#15152=VERTEX_POINT('',#76467);
#15153=VERTEX_POINT('',#76471);
#15154=VERTEX_POINT('',#76473);
#15155=VERTEX_POINT('',#76477);
#15156=VERTEX_POINT('',#76479);
#15157=VERTEX_POINT('',#76487);
#15158=VERTEX_POINT('',#76488);
#15159=VERTEX_POINT('',#76490);
#15160=VERTEX_POINT('',#76492);
#15161=VERTEX_POINT('',#76496);
#15162=VERTEX_POINT('',#76498);
#15163=VERTEX_POINT('',#76502);
#15164=VERTEX_POINT('',#76504);
#15165=VERTEX_POINT('',#76512);
#15166=VERTEX_POINT('',#76513);
#15167=VERTEX_POINT('',#76515);
#15168=VERTEX_POINT('',#76517);
#15169=VERTEX_POINT('',#76521);
#15170=VERTEX_POINT('',#76523);
#15171=VERTEX_POINT('',#76527);
#15172=VERTEX_POINT('',#76529);
#15173=VERTEX_POINT('',#76537);
#15174=VERTEX_POINT('',#76538);
#15175=VERTEX_POINT('',#76540);
#15176=VERTEX_POINT('',#76542);
#15177=VERTEX_POINT('',#76546);
#15178=VERTEX_POINT('',#76548);
#15179=VERTEX_POINT('',#76552);
#15180=VERTEX_POINT('',#76554);
#15181=VERTEX_POINT('',#76562);
#15182=VERTEX_POINT('',#76563);
#15183=VERTEX_POINT('',#76565);
#15184=VERTEX_POINT('',#76567);
#15185=VERTEX_POINT('',#76571);
#15186=VERTEX_POINT('',#76573);
#15187=VERTEX_POINT('',#76577);
#15188=VERTEX_POINT('',#76579);
#15189=VERTEX_POINT('',#76587);
#15190=VERTEX_POINT('',#76589);
#15191=VERTEX_POINT('',#76593);
#15192=VERTEX_POINT('',#76595);
#15193=VERTEX_POINT('',#76599);
#15194=VERTEX_POINT('',#76600);
#15195=VERTEX_POINT('',#76602);
#15196=VERTEX_POINT('',#76604);
#15197=VERTEX_POINT('',#76608);
#15198=VERTEX_POINT('',#76610);
#15199=VERTEX_POINT('',#76614);
#15200=VERTEX_POINT('',#76616);
#15201=VERTEX_POINT('',#76620);
#15202=VERTEX_POINT('',#76622);
#15203=VERTEX_POINT('',#76626);
#15204=VERTEX_POINT('',#76628);
#15205=VERTEX_POINT('',#76632);
#15206=VERTEX_POINT('',#76634);
#15207=VERTEX_POINT('',#76638);
#15208=VERTEX_POINT('',#76640);
#17242=EDGE_CURVE('',#13849,#13850,#820,.T.);
#17243=EDGE_CURVE('',#13849,#13851,#7586,.T.);
#17244=EDGE_CURVE('',#13851,#13852,#821,.T.);
#17245=EDGE_CURVE('',#13850,#13852,#7587,.T.);
#17246=EDGE_CURVE('',#13853,#13849,#822,.T.);
#17247=EDGE_CURVE('',#13853,#13854,#7588,.T.);
#17248=EDGE_CURVE('',#13854,#13851,#823,.T.);
#17249=EDGE_CURVE('',#13855,#13853,#824,.T.);
#17250=EDGE_CURVE('',#13855,#13856,#7589,.T.);
#17251=EDGE_CURVE('',#13856,#13854,#825,.T.);
#17252=EDGE_CURVE('',#13857,#13855,#826,.T.);
#17253=EDGE_CURVE('',#13857,#13858,#7590,.T.);
#17254=EDGE_CURVE('',#13858,#13856,#827,.T.);
#17255=EDGE_CURVE('',#13859,#13857,#828,.T.);
#17256=EDGE_CURVE('',#13859,#13860,#7591,.T.);
#17257=EDGE_CURVE('',#13860,#13858,#829,.T.);
#17258=EDGE_CURVE('',#13861,#13859,#830,.T.);
#17259=EDGE_CURVE('',#13861,#13862,#7592,.T.);
#17260=EDGE_CURVE('',#13862,#13860,#831,.T.);
#17261=EDGE_CURVE('',#13863,#13861,#832,.T.);
#17262=EDGE_CURVE('',#13863,#13864,#7593,.T.);
#17263=EDGE_CURVE('',#13864,#13862,#833,.T.);
#17264=EDGE_CURVE('',#13850,#13863,#834,.T.);
#17265=EDGE_CURVE('',#13852,#13864,#835,.T.);
#17266=EDGE_CURVE('',#13865,#13866,#836,.T.);
#17267=EDGE_CURVE('',#13865,#13867,#7594,.T.);
#17268=EDGE_CURVE('',#13867,#13868,#837,.T.);
#17269=EDGE_CURVE('',#13866,#13868,#7595,.T.);
#17270=EDGE_CURVE('',#13869,#13865,#838,.T.);
#17271=EDGE_CURVE('',#13869,#13870,#7596,.T.);
#17272=EDGE_CURVE('',#13870,#13867,#839,.T.);
#17273=EDGE_CURVE('',#13871,#13869,#840,.T.);
#17274=EDGE_CURVE('',#13871,#13872,#7597,.T.);
#17275=EDGE_CURVE('',#13872,#13870,#841,.T.);
#17276=EDGE_CURVE('',#13873,#13871,#842,.T.);
#17277=EDGE_CURVE('',#13873,#13874,#7598,.T.);
#17278=EDGE_CURVE('',#13874,#13872,#843,.T.);
#17279=EDGE_CURVE('',#13875,#13873,#844,.T.);
#17280=EDGE_CURVE('',#13875,#13876,#7599,.T.);
#17281=EDGE_CURVE('',#13876,#13874,#845,.T.);
#17282=EDGE_CURVE('',#13877,#13875,#846,.T.);
#17283=EDGE_CURVE('',#13877,#13878,#7600,.T.);
#17284=EDGE_CURVE('',#13878,#13876,#847,.T.);
#17285=EDGE_CURVE('',#13879,#13877,#848,.T.);
#17286=EDGE_CURVE('',#13879,#13880,#7601,.T.);
#17287=EDGE_CURVE('',#13880,#13878,#849,.T.);
#17288=EDGE_CURVE('',#13881,#13879,#850,.T.);
#17289=EDGE_CURVE('',#13881,#13882,#7602,.T.);
#17290=EDGE_CURVE('',#13882,#13880,#851,.T.);
#17291=EDGE_CURVE('',#13883,#13881,#852,.T.);
#17292=EDGE_CURVE('',#13883,#13884,#7603,.T.);
#17293=EDGE_CURVE('',#13884,#13882,#853,.T.);
#17294=EDGE_CURVE('',#13885,#13883,#854,.T.);
#17295=EDGE_CURVE('',#13885,#13886,#7604,.T.);
#17296=EDGE_CURVE('',#13886,#13884,#855,.T.);
#17297=EDGE_CURVE('',#13887,#13885,#856,.T.);
#17298=EDGE_CURVE('',#13887,#13888,#7605,.T.);
#17299=EDGE_CURVE('',#13888,#13886,#857,.T.);
#17300=EDGE_CURVE('',#13866,#13887,#858,.T.);
#17301=EDGE_CURVE('',#13868,#13888,#859,.T.);
#17302=EDGE_CURVE('',#13889,#13890,#7606,.T.);
#17303=EDGE_CURVE('',#13889,#13891,#7607,.T.);
#17304=EDGE_CURVE('',#13891,#13892,#7608,.T.);
#17305=EDGE_CURVE('',#13890,#13892,#7609,.T.);
#17306=EDGE_CURVE('',#13893,#13889,#7610,.T.);
#17307=EDGE_CURVE('',#13893,#13894,#7611,.T.);
#17308=EDGE_CURVE('',#13894,#13891,#7612,.T.);
#17309=EDGE_CURVE('',#13890,#13893,#7613,.T.);
#17310=EDGE_CURVE('',#13892,#13894,#7614,.T.);
#17311=EDGE_CURVE('',#13895,#13896,#7615,.T.);
#17312=EDGE_CURVE('',#13895,#13897,#7616,.T.);
#17313=EDGE_CURVE('',#13897,#13898,#7617,.T.);
#17314=EDGE_CURVE('',#13896,#13898,#7618,.T.);
#17315=EDGE_CURVE('',#13899,#13895,#7619,.T.);
#17316=EDGE_CURVE('',#13899,#13900,#7620,.T.);
#17317=EDGE_CURVE('',#13900,#13897,#7621,.T.);
#17318=EDGE_CURVE('',#13901,#13899,#7622,.T.);
#17319=EDGE_CURVE('',#13901,#13902,#7623,.T.);
#17320=EDGE_CURVE('',#13902,#13900,#7624,.T.);
#17321=EDGE_CURVE('',#13903,#13901,#7625,.T.);
#17322=EDGE_CURVE('',#13903,#13904,#7626,.T.);
#17323=EDGE_CURVE('',#13904,#13902,#7627,.T.);
#17324=EDGE_CURVE('',#13905,#13903,#7628,.T.);
#17325=EDGE_CURVE('',#13905,#13906,#7629,.T.);
#17326=EDGE_CURVE('',#13906,#13904,#7630,.T.);
#17327=EDGE_CURVE('',#13907,#13905,#7631,.T.);
#17328=EDGE_CURVE('',#13907,#13908,#7632,.T.);
#17329=EDGE_CURVE('',#13908,#13906,#7633,.T.);
#17330=EDGE_CURVE('',#13909,#13907,#7634,.T.);
#17331=EDGE_CURVE('',#13909,#13910,#7635,.T.);
#17332=EDGE_CURVE('',#13910,#13908,#7636,.T.);
#17333=EDGE_CURVE('',#13911,#13909,#7637,.T.);
#17334=EDGE_CURVE('',#13911,#13912,#7638,.T.);
#17335=EDGE_CURVE('',#13912,#13910,#7639,.T.);
#17336=EDGE_CURVE('',#13913,#13911,#7640,.T.);
#17337=EDGE_CURVE('',#13913,#13914,#7641,.T.);
#17338=EDGE_CURVE('',#13914,#13912,#7642,.T.);
#17339=EDGE_CURVE('',#13915,#13913,#7643,.T.);
#17340=EDGE_CURVE('',#13915,#13916,#7644,.T.);
#17341=EDGE_CURVE('',#13916,#13914,#7645,.T.);
#17342=EDGE_CURVE('',#13896,#13915,#7646,.T.);
#17343=EDGE_CURVE('',#13898,#13916,#7647,.T.);
#17344=EDGE_CURVE('',#13917,#13918,#860,.T.);
#17345=EDGE_CURVE('',#13917,#13919,#7648,.T.);
#17346=EDGE_CURVE('',#13919,#13920,#861,.T.);
#17347=EDGE_CURVE('',#13918,#13920,#7649,.T.);
#17348=EDGE_CURVE('',#13921,#13917,#862,.T.);
#17349=EDGE_CURVE('',#13921,#13922,#7650,.T.);
#17350=EDGE_CURVE('',#13922,#13919,#863,.T.);
#17351=EDGE_CURVE('',#13923,#13921,#864,.T.);
#17352=EDGE_CURVE('',#13923,#13924,#7651,.T.);
#17353=EDGE_CURVE('',#13924,#13922,#865,.T.);
#17354=EDGE_CURVE('',#13925,#13923,#866,.T.);
#17355=EDGE_CURVE('',#13925,#13926,#7652,.T.);
#17356=EDGE_CURVE('',#13926,#13924,#867,.T.);
#17357=EDGE_CURVE('',#13927,#13925,#868,.T.);
#17358=EDGE_CURVE('',#13927,#13928,#7653,.T.);
#17359=EDGE_CURVE('',#13928,#13926,#869,.T.);
#17360=EDGE_CURVE('',#13929,#13927,#870,.T.);
#17361=EDGE_CURVE('',#13929,#13930,#7654,.T.);
#17362=EDGE_CURVE('',#13930,#13928,#871,.T.);
#17363=EDGE_CURVE('',#13931,#13929,#872,.T.);
#17364=EDGE_CURVE('',#13931,#13932,#7655,.T.);
#17365=EDGE_CURVE('',#13932,#13930,#873,.T.);
#17366=EDGE_CURVE('',#13918,#13931,#874,.T.);
#17367=EDGE_CURVE('',#13920,#13932,#875,.T.);
#17368=EDGE_CURVE('',#13933,#13934,#876,.T.);
#17369=EDGE_CURVE('',#13933,#13935,#7656,.T.);
#17370=EDGE_CURVE('',#13935,#13936,#877,.T.);
#17371=EDGE_CURVE('',#13934,#13936,#7657,.T.);
#17372=EDGE_CURVE('',#13937,#13933,#878,.T.);
#17373=EDGE_CURVE('',#13937,#13938,#7658,.T.);
#17374=EDGE_CURVE('',#13938,#13935,#879,.T.);
#17375=EDGE_CURVE('',#13939,#13937,#880,.T.);
#17376=EDGE_CURVE('',#13939,#13940,#7659,.T.);
#17377=EDGE_CURVE('',#13940,#13938,#881,.T.);
#17378=EDGE_CURVE('',#13941,#13939,#882,.T.);
#17379=EDGE_CURVE('',#13941,#13942,#7660,.T.);
#17380=EDGE_CURVE('',#13942,#13940,#883,.T.);
#17381=EDGE_CURVE('',#13943,#13941,#884,.T.);
#17382=EDGE_CURVE('',#13943,#13944,#7661,.T.);
#17383=EDGE_CURVE('',#13944,#13942,#885,.T.);
#17384=EDGE_CURVE('',#13945,#13943,#886,.T.);
#17385=EDGE_CURVE('',#13945,#13946,#7662,.T.);
#17386=EDGE_CURVE('',#13946,#13944,#887,.T.);
#17387=EDGE_CURVE('',#13947,#13945,#888,.T.);
#17388=EDGE_CURVE('',#13947,#13948,#7663,.T.);
#17389=EDGE_CURVE('',#13948,#13946,#889,.T.);
#17390=EDGE_CURVE('',#13949,#13947,#890,.T.);
#17391=EDGE_CURVE('',#13949,#13950,#7664,.T.);
#17392=EDGE_CURVE('',#13950,#13948,#891,.T.);
#17393=EDGE_CURVE('',#13951,#13949,#892,.T.);
#17394=EDGE_CURVE('',#13951,#13952,#7665,.T.);
#17395=EDGE_CURVE('',#13952,#13950,#893,.T.);
#17396=EDGE_CURVE('',#13953,#13951,#894,.T.);
#17397=EDGE_CURVE('',#13953,#13954,#7666,.T.);
#17398=EDGE_CURVE('',#13954,#13952,#895,.T.);
#17399=EDGE_CURVE('',#13955,#13953,#896,.T.);
#17400=EDGE_CURVE('',#13955,#13956,#7667,.T.);
#17401=EDGE_CURVE('',#13956,#13954,#897,.T.);
#17402=EDGE_CURVE('',#13934,#13955,#898,.T.);
#17403=EDGE_CURVE('',#13936,#13956,#899,.T.);
#17404=EDGE_CURVE('',#13957,#13958,#900,.T.);
#17405=EDGE_CURVE('',#13957,#13959,#7668,.T.);
#17406=EDGE_CURVE('',#13959,#13960,#901,.T.);
#17407=EDGE_CURVE('',#13958,#13960,#7669,.T.);
#17408=EDGE_CURVE('',#13961,#13957,#902,.T.);
#17409=EDGE_CURVE('',#13961,#13962,#7670,.T.);
#17410=EDGE_CURVE('',#13962,#13959,#903,.T.);
#17411=EDGE_CURVE('',#13963,#13961,#904,.T.);
#17412=EDGE_CURVE('',#13963,#13964,#7671,.T.);
#17413=EDGE_CURVE('',#13964,#13962,#905,.T.);
#17414=EDGE_CURVE('',#13965,#13963,#906,.T.);
#17415=EDGE_CURVE('',#13965,#13966,#7672,.T.);
#17416=EDGE_CURVE('',#13966,#13964,#907,.T.);
#17417=EDGE_CURVE('',#13967,#13965,#908,.T.);
#17418=EDGE_CURVE('',#13967,#13968,#7673,.T.);
#17419=EDGE_CURVE('',#13968,#13966,#909,.T.);
#17420=EDGE_CURVE('',#13969,#13967,#910,.T.);
#17421=EDGE_CURVE('',#13969,#13970,#7674,.T.);
#17422=EDGE_CURVE('',#13970,#13968,#911,.T.);
#17423=EDGE_CURVE('',#13971,#13969,#912,.T.);
#17424=EDGE_CURVE('',#13971,#13972,#7675,.T.);
#17425=EDGE_CURVE('',#13972,#13970,#913,.T.);
#17426=EDGE_CURVE('',#13973,#13971,#914,.T.);
#17427=EDGE_CURVE('',#13973,#13974,#7676,.T.);
#17428=EDGE_CURVE('',#13974,#13972,#915,.T.);
#17429=EDGE_CURVE('',#13975,#13973,#916,.T.);
#17430=EDGE_CURVE('',#13975,#13976,#7677,.T.);
#17431=EDGE_CURVE('',#13976,#13974,#917,.T.);
#17432=EDGE_CURVE('',#13977,#13975,#918,.T.);
#17433=EDGE_CURVE('',#13977,#13978,#7678,.T.);
#17434=EDGE_CURVE('',#13978,#13976,#919,.T.);
#17435=EDGE_CURVE('',#13979,#13977,#920,.T.);
#17436=EDGE_CURVE('',#13979,#13980,#7679,.T.);
#17437=EDGE_CURVE('',#13980,#13978,#921,.T.);
#17438=EDGE_CURVE('',#13981,#13979,#922,.T.);
#17439=EDGE_CURVE('',#13981,#13982,#7680,.T.);
#17440=EDGE_CURVE('',#13982,#13980,#923,.T.);
#17441=EDGE_CURVE('',#13983,#13981,#7681,.T.);
#17442=EDGE_CURVE('',#13983,#13984,#7682,.T.);
#17443=EDGE_CURVE('',#13984,#13982,#7683,.T.);
#17444=EDGE_CURVE('',#13985,#13983,#924,.T.);
#17445=EDGE_CURVE('',#13985,#13986,#7684,.T.);
#17446=EDGE_CURVE('',#13986,#13984,#925,.T.);
#17447=EDGE_CURVE('',#13987,#13985,#926,.T.);
#17448=EDGE_CURVE('',#13987,#13988,#7685,.T.);
#17449=EDGE_CURVE('',#13988,#13986,#927,.T.);
#17450=EDGE_CURVE('',#13989,#13987,#928,.T.);
#17451=EDGE_CURVE('',#13989,#13990,#7686,.T.);
#17452=EDGE_CURVE('',#13990,#13988,#929,.T.);
#17453=EDGE_CURVE('',#13991,#13989,#930,.T.);
#17454=EDGE_CURVE('',#13991,#13992,#7687,.T.);
#17455=EDGE_CURVE('',#13992,#13990,#931,.T.);
#17456=EDGE_CURVE('',#13993,#13991,#932,.T.);
#17457=EDGE_CURVE('',#13993,#13994,#7688,.T.);
#17458=EDGE_CURVE('',#13994,#13992,#933,.T.);
#17459=EDGE_CURVE('',#13995,#13993,#934,.T.);
#17460=EDGE_CURVE('',#13995,#13996,#7689,.T.);
#17461=EDGE_CURVE('',#13996,#13994,#935,.T.);
#17462=EDGE_CURVE('',#13997,#13995,#936,.T.);
#17463=EDGE_CURVE('',#13997,#13998,#7690,.T.);
#17464=EDGE_CURVE('',#13998,#13996,#937,.T.);
#17465=EDGE_CURVE('',#13999,#13997,#7691,.T.);
#17466=EDGE_CURVE('',#13999,#14000,#7692,.T.);
#17467=EDGE_CURVE('',#14000,#13998,#7693,.T.);
#17468=EDGE_CURVE('',#14001,#13999,#938,.T.);
#17469=EDGE_CURVE('',#14001,#14002,#7694,.T.);
#17470=EDGE_CURVE('',#14002,#14000,#939,.T.);
#17471=EDGE_CURVE('',#14003,#14001,#940,.T.);
#17472=EDGE_CURVE('',#14003,#14004,#7695,.T.);
#17473=EDGE_CURVE('',#14004,#14002,#941,.T.);
#17474=EDGE_CURVE('',#14005,#14003,#942,.T.);
#17475=EDGE_CURVE('',#14005,#14006,#7696,.T.);
#17476=EDGE_CURVE('',#14006,#14004,#943,.T.);
#17477=EDGE_CURVE('',#14007,#14005,#944,.T.);
#17478=EDGE_CURVE('',#14007,#14008,#7697,.T.);
#17479=EDGE_CURVE('',#14008,#14006,#945,.T.);
#17480=EDGE_CURVE('',#14009,#14007,#946,.T.);
#17481=EDGE_CURVE('',#14009,#14010,#7698,.T.);
#17482=EDGE_CURVE('',#14010,#14008,#947,.T.);
#17483=EDGE_CURVE('',#14011,#14009,#948,.T.);
#17484=EDGE_CURVE('',#14011,#14012,#7699,.T.);
#17485=EDGE_CURVE('',#14012,#14010,#949,.T.);
#17486=EDGE_CURVE('',#14013,#14011,#950,.T.);
#17487=EDGE_CURVE('',#14013,#14014,#7700,.T.);
#17488=EDGE_CURVE('',#14014,#14012,#951,.T.);
#17489=EDGE_CURVE('',#14015,#14013,#7701,.T.);
#17490=EDGE_CURVE('',#14015,#14016,#7702,.T.);
#17491=EDGE_CURVE('',#14016,#14014,#7703,.T.);
#17492=EDGE_CURVE('',#13958,#14015,#952,.T.);
#17493=EDGE_CURVE('',#13960,#14016,#953,.T.);
#17494=EDGE_CURVE('',#14017,#14018,#954,.T.);
#17495=EDGE_CURVE('',#14017,#14019,#7704,.T.);
#17496=EDGE_CURVE('',#14019,#14020,#955,.T.);
#17497=EDGE_CURVE('',#14018,#14020,#7705,.T.);
#17498=EDGE_CURVE('',#14021,#14017,#956,.T.);
#17499=EDGE_CURVE('',#14021,#14022,#7706,.T.);
#17500=EDGE_CURVE('',#14022,#14019,#957,.T.);
#17501=EDGE_CURVE('',#14023,#14021,#958,.T.);
#17502=EDGE_CURVE('',#14023,#14024,#7707,.T.);
#17503=EDGE_CURVE('',#14024,#14022,#959,.T.);
#17504=EDGE_CURVE('',#14025,#14023,#960,.T.);
#17505=EDGE_CURVE('',#14025,#14026,#7708,.T.);
#17506=EDGE_CURVE('',#14026,#14024,#961,.T.);
#17507=EDGE_CURVE('',#14027,#14025,#962,.T.);
#17508=EDGE_CURVE('',#14027,#14028,#7709,.T.);
#17509=EDGE_CURVE('',#14028,#14026,#963,.T.);
#17510=EDGE_CURVE('',#14029,#14027,#964,.T.);
#17511=EDGE_CURVE('',#14029,#14030,#7710,.T.);
#17512=EDGE_CURVE('',#14030,#14028,#965,.T.);
#17513=EDGE_CURVE('',#14031,#14029,#966,.T.);
#17514=EDGE_CURVE('',#14031,#14032,#7711,.T.);
#17515=EDGE_CURVE('',#14032,#14030,#967,.T.);
#17516=EDGE_CURVE('',#14018,#14031,#968,.T.);
#17517=EDGE_CURVE('',#14020,#14032,#969,.T.);
#17518=EDGE_CURVE('',#14033,#14034,#970,.T.);
#17519=EDGE_CURVE('',#14033,#14035,#7712,.T.);
#17520=EDGE_CURVE('',#14035,#14036,#971,.T.);
#17521=EDGE_CURVE('',#14034,#14036,#7713,.T.);
#17522=EDGE_CURVE('',#14037,#14033,#972,.T.);
#17523=EDGE_CURVE('',#14037,#14038,#7714,.T.);
#17524=EDGE_CURVE('',#14038,#14035,#973,.T.);
#17525=EDGE_CURVE('',#14039,#14037,#974,.T.);
#17526=EDGE_CURVE('',#14039,#14040,#7715,.T.);
#17527=EDGE_CURVE('',#14040,#14038,#975,.T.);
#17528=EDGE_CURVE('',#14041,#14039,#976,.T.);
#17529=EDGE_CURVE('',#14041,#14042,#7716,.T.);
#17530=EDGE_CURVE('',#14042,#14040,#977,.T.);
#17531=EDGE_CURVE('',#14043,#14041,#978,.T.);
#17532=EDGE_CURVE('',#14043,#14044,#7717,.T.);
#17533=EDGE_CURVE('',#14044,#14042,#979,.T.);
#17534=EDGE_CURVE('',#14045,#14043,#980,.T.);
#17535=EDGE_CURVE('',#14045,#14046,#7718,.T.);
#17536=EDGE_CURVE('',#14046,#14044,#981,.T.);
#17537=EDGE_CURVE('',#14047,#14045,#982,.T.);
#17538=EDGE_CURVE('',#14047,#14048,#7719,.T.);
#17539=EDGE_CURVE('',#14048,#14046,#983,.T.);
#17540=EDGE_CURVE('',#14049,#14047,#984,.T.);
#17541=EDGE_CURVE('',#14049,#14050,#7720,.T.);
#17542=EDGE_CURVE('',#14050,#14048,#985,.T.);
#17543=EDGE_CURVE('',#14051,#14049,#986,.T.);
#17544=EDGE_CURVE('',#14051,#14052,#7721,.T.);
#17545=EDGE_CURVE('',#14052,#14050,#987,.T.);
#17546=EDGE_CURVE('',#14053,#14051,#988,.T.);
#17547=EDGE_CURVE('',#14053,#14054,#7722,.T.);
#17548=EDGE_CURVE('',#14054,#14052,#989,.T.);
#17549=EDGE_CURVE('',#14055,#14053,#990,.T.);
#17550=EDGE_CURVE('',#14055,#14056,#7723,.T.);
#17551=EDGE_CURVE('',#14056,#14054,#991,.T.);
#17552=EDGE_CURVE('',#14034,#14055,#992,.T.);
#17553=EDGE_CURVE('',#14036,#14056,#993,.T.);
#17554=EDGE_CURVE('',#14057,#14058,#994,.T.);
#17555=EDGE_CURVE('',#14057,#14059,#7724,.T.);
#17556=EDGE_CURVE('',#14059,#14060,#995,.T.);
#17557=EDGE_CURVE('',#14058,#14060,#7725,.T.);
#17558=EDGE_CURVE('',#14061,#14057,#996,.T.);
#17559=EDGE_CURVE('',#14061,#14062,#7726,.T.);
#17560=EDGE_CURVE('',#14062,#14059,#997,.T.);
#17561=EDGE_CURVE('',#14063,#14061,#998,.T.);
#17562=EDGE_CURVE('',#14063,#14064,#7727,.T.);
#17563=EDGE_CURVE('',#14064,#14062,#999,.T.);
#17564=EDGE_CURVE('',#14065,#14063,#1000,.T.);
#17565=EDGE_CURVE('',#14065,#14066,#7728,.T.);
#17566=EDGE_CURVE('',#14066,#14064,#1001,.T.);
#17567=EDGE_CURVE('',#14067,#14065,#1002,.T.);
#17568=EDGE_CURVE('',#14067,#14068,#7729,.T.);
#17569=EDGE_CURVE('',#14068,#14066,#1003,.T.);
#17570=EDGE_CURVE('',#14069,#14067,#1004,.T.);
#17571=EDGE_CURVE('',#14069,#14070,#7730,.T.);
#17572=EDGE_CURVE('',#14070,#14068,#1005,.T.);
#17573=EDGE_CURVE('',#14071,#14069,#1006,.T.);
#17574=EDGE_CURVE('',#14071,#14072,#7731,.T.);
#17575=EDGE_CURVE('',#14072,#14070,#1007,.T.);
#17576=EDGE_CURVE('',#14073,#14071,#1008,.T.);
#17577=EDGE_CURVE('',#14073,#14074,#7732,.T.);
#17578=EDGE_CURVE('',#14074,#14072,#1009,.T.);
#17579=EDGE_CURVE('',#14075,#14073,#1010,.T.);
#17580=EDGE_CURVE('',#14075,#14076,#7733,.T.);
#17581=EDGE_CURVE('',#14076,#14074,#1011,.T.);
#17582=EDGE_CURVE('',#14077,#14075,#7734,.T.);
#17583=EDGE_CURVE('',#14077,#14078,#7735,.T.);
#17584=EDGE_CURVE('',#14078,#14076,#7736,.T.);
#17585=EDGE_CURVE('',#14079,#14077,#1012,.T.);
#17586=EDGE_CURVE('',#14079,#14080,#7737,.T.);
#17587=EDGE_CURVE('',#14080,#14078,#1013,.T.);
#17588=EDGE_CURVE('',#14081,#14079,#1014,.T.);
#17589=EDGE_CURVE('',#14081,#14082,#7738,.T.);
#17590=EDGE_CURVE('',#14082,#14080,#1015,.T.);
#17591=EDGE_CURVE('',#14083,#14081,#1016,.T.);
#17592=EDGE_CURVE('',#14083,#14084,#7739,.T.);
#17593=EDGE_CURVE('',#14084,#14082,#1017,.T.);
#17594=EDGE_CURVE('',#14085,#14083,#1018,.T.);
#17595=EDGE_CURVE('',#14085,#14086,#7740,.T.);
#17596=EDGE_CURVE('',#14086,#14084,#1019,.T.);
#17597=EDGE_CURVE('',#14087,#14085,#1020,.T.);
#17598=EDGE_CURVE('',#14087,#14088,#7741,.T.);
#17599=EDGE_CURVE('',#14088,#14086,#1021,.T.);
#17600=EDGE_CURVE('',#14089,#14087,#1022,.T.);
#17601=EDGE_CURVE('',#14089,#14090,#7742,.T.);
#17602=EDGE_CURVE('',#14090,#14088,#1023,.T.);
#17603=EDGE_CURVE('',#14091,#14089,#1024,.T.);
#17604=EDGE_CURVE('',#14091,#14092,#7743,.T.);
#17605=EDGE_CURVE('',#14092,#14090,#1025,.T.);
#17606=EDGE_CURVE('',#14093,#14091,#1026,.T.);
#17607=EDGE_CURVE('',#14093,#14094,#7744,.T.);
#17608=EDGE_CURVE('',#14094,#14092,#1027,.T.);
#17609=EDGE_CURVE('',#14095,#14093,#1028,.T.);
#17610=EDGE_CURVE('',#14095,#14096,#7745,.T.);
#17611=EDGE_CURVE('',#14096,#14094,#1029,.T.);
#17612=EDGE_CURVE('',#14097,#14095,#7746,.T.);
#17613=EDGE_CURVE('',#14097,#14098,#7747,.T.);
#17614=EDGE_CURVE('',#14098,#14096,#7748,.T.);
#17615=EDGE_CURVE('',#14099,#14097,#7749,.T.);
#17616=EDGE_CURVE('',#14099,#14100,#7750,.T.);
#17617=EDGE_CURVE('',#14100,#14098,#7751,.T.);
#17618=EDGE_CURVE('',#14058,#14099,#7752,.T.);
#17619=EDGE_CURVE('',#14060,#14100,#7753,.T.);
#17620=EDGE_CURVE('',#14101,#14102,#1030,.T.);
#17621=EDGE_CURVE('',#14101,#14103,#7754,.T.);
#17622=EDGE_CURVE('',#14103,#14104,#1031,.T.);
#17623=EDGE_CURVE('',#14102,#14104,#7755,.T.);
#17624=EDGE_CURVE('',#14105,#14101,#1032,.T.);
#17625=EDGE_CURVE('',#14105,#14106,#7756,.T.);
#17626=EDGE_CURVE('',#14106,#14103,#1033,.T.);
#17627=EDGE_CURVE('',#14107,#14105,#1034,.T.);
#17628=EDGE_CURVE('',#14107,#14108,#7757,.T.);
#17629=EDGE_CURVE('',#14108,#14106,#1035,.T.);
#17630=EDGE_CURVE('',#14109,#14107,#1036,.T.);
#17631=EDGE_CURVE('',#14109,#14110,#7758,.T.);
#17632=EDGE_CURVE('',#14110,#14108,#1037,.T.);
#17633=EDGE_CURVE('',#14111,#14109,#1038,.T.);
#17634=EDGE_CURVE('',#14111,#14112,#7759,.T.);
#17635=EDGE_CURVE('',#14112,#14110,#1039,.T.);
#17636=EDGE_CURVE('',#14113,#14111,#1040,.T.);
#17637=EDGE_CURVE('',#14113,#14114,#7760,.T.);
#17638=EDGE_CURVE('',#14114,#14112,#1041,.T.);
#17639=EDGE_CURVE('',#14115,#14113,#1042,.T.);
#17640=EDGE_CURVE('',#14115,#14116,#7761,.T.);
#17641=EDGE_CURVE('',#14116,#14114,#1043,.T.);
#17642=EDGE_CURVE('',#14102,#14115,#1044,.T.);
#17643=EDGE_CURVE('',#14104,#14116,#1045,.T.);
#17644=EDGE_CURVE('',#14117,#14118,#1046,.T.);
#17645=EDGE_CURVE('',#14117,#14119,#7762,.T.);
#17646=EDGE_CURVE('',#14119,#14120,#1047,.T.);
#17647=EDGE_CURVE('',#14118,#14120,#7763,.T.);
#17648=EDGE_CURVE('',#14121,#14117,#1048,.T.);
#17649=EDGE_CURVE('',#14121,#14122,#7764,.T.);
#17650=EDGE_CURVE('',#14122,#14119,#1049,.T.);
#17651=EDGE_CURVE('',#14123,#14121,#1050,.T.);
#17652=EDGE_CURVE('',#14123,#14124,#7765,.T.);
#17653=EDGE_CURVE('',#14124,#14122,#1051,.T.);
#17654=EDGE_CURVE('',#14125,#14123,#1052,.T.);
#17655=EDGE_CURVE('',#14125,#14126,#7766,.T.);
#17656=EDGE_CURVE('',#14126,#14124,#1053,.T.);
#17657=EDGE_CURVE('',#14127,#14125,#1054,.T.);
#17658=EDGE_CURVE('',#14127,#14128,#7767,.T.);
#17659=EDGE_CURVE('',#14128,#14126,#1055,.T.);
#17660=EDGE_CURVE('',#14129,#14127,#1056,.T.);
#17661=EDGE_CURVE('',#14129,#14130,#7768,.T.);
#17662=EDGE_CURVE('',#14130,#14128,#1057,.T.);
#17663=EDGE_CURVE('',#14131,#14129,#1058,.T.);
#17664=EDGE_CURVE('',#14131,#14132,#7769,.T.);
#17665=EDGE_CURVE('',#14132,#14130,#1059,.T.);
#17666=EDGE_CURVE('',#14133,#14131,#1060,.T.);
#17667=EDGE_CURVE('',#14133,#14134,#7770,.T.);
#17668=EDGE_CURVE('',#14134,#14132,#1061,.T.);
#17669=EDGE_CURVE('',#14135,#14133,#1062,.T.);
#17670=EDGE_CURVE('',#14135,#14136,#7771,.T.);
#17671=EDGE_CURVE('',#14136,#14134,#1063,.T.);
#17672=EDGE_CURVE('',#14137,#14135,#1064,.T.);
#17673=EDGE_CURVE('',#14137,#14138,#7772,.T.);
#17674=EDGE_CURVE('',#14138,#14136,#1065,.T.);
#17675=EDGE_CURVE('',#14139,#14137,#1066,.T.);
#17676=EDGE_CURVE('',#14139,#14140,#7773,.T.);
#17677=EDGE_CURVE('',#14140,#14138,#1067,.T.);
#17678=EDGE_CURVE('',#14118,#14139,#1068,.T.);
#17679=EDGE_CURVE('',#14120,#14140,#1069,.T.);
#17680=EDGE_CURVE('',#14141,#14142,#7774,.T.);
#17681=EDGE_CURVE('',#14141,#14143,#7775,.T.);
#17682=EDGE_CURVE('',#14143,#14144,#7776,.T.);
#17683=EDGE_CURVE('',#14142,#14144,#7777,.T.);
#17684=EDGE_CURVE('',#14145,#14141,#1070,.T.);
#17685=EDGE_CURVE('',#14145,#14146,#7778,.T.);
#17686=EDGE_CURVE('',#14146,#14143,#1071,.T.);
#17687=EDGE_CURVE('',#14147,#14145,#1072,.T.);
#17688=EDGE_CURVE('',#14147,#14148,#7779,.T.);
#17689=EDGE_CURVE('',#14148,#14146,#1073,.T.);
#17690=EDGE_CURVE('',#14149,#14147,#7780,.T.);
#17691=EDGE_CURVE('',#14149,#14150,#7781,.T.);
#17692=EDGE_CURVE('',#14150,#14148,#7782,.T.);
#17693=EDGE_CURVE('',#14151,#14149,#1074,.T.);
#17694=EDGE_CURVE('',#14151,#14152,#7783,.T.);
#17695=EDGE_CURVE('',#14152,#14150,#1075,.T.);
#17696=EDGE_CURVE('',#14153,#14151,#1076,.T.);
#17697=EDGE_CURVE('',#14153,#14154,#7784,.T.);
#17698=EDGE_CURVE('',#14154,#14152,#1077,.T.);
#17699=EDGE_CURVE('',#14155,#14153,#7785,.T.);
#17700=EDGE_CURVE('',#14155,#14156,#7786,.T.);
#17701=EDGE_CURVE('',#14156,#14154,#7787,.T.);
#17702=EDGE_CURVE('',#14157,#14155,#7788,.T.);
#17703=EDGE_CURVE('',#14157,#14158,#7789,.T.);
#17704=EDGE_CURVE('',#14158,#14156,#7790,.T.);
#17705=EDGE_CURVE('',#14142,#14157,#7791,.T.);
#17706=EDGE_CURVE('',#14144,#14158,#7792,.T.);
#17707=EDGE_CURVE('',#14159,#14160,#1078,.T.);
#17708=EDGE_CURVE('',#14159,#14161,#7793,.T.);
#17709=EDGE_CURVE('',#14161,#14162,#1079,.T.);
#17710=EDGE_CURVE('',#14160,#14162,#7794,.T.);
#17711=EDGE_CURVE('',#14163,#14159,#1080,.T.);
#17712=EDGE_CURVE('',#14163,#14164,#7795,.T.);
#17713=EDGE_CURVE('',#14164,#14161,#1081,.T.);
#17714=EDGE_CURVE('',#14165,#14163,#1082,.T.);
#17715=EDGE_CURVE('',#14165,#14166,#7796,.T.);
#17716=EDGE_CURVE('',#14166,#14164,#1083,.T.);
#17717=EDGE_CURVE('',#14167,#14165,#1084,.T.);
#17718=EDGE_CURVE('',#14167,#14168,#7797,.T.);
#17719=EDGE_CURVE('',#14168,#14166,#1085,.T.);
#17720=EDGE_CURVE('',#14169,#14167,#1086,.T.);
#17721=EDGE_CURVE('',#14169,#14170,#7798,.T.);
#17722=EDGE_CURVE('',#14170,#14168,#1087,.T.);
#17723=EDGE_CURVE('',#14171,#14169,#1088,.T.);
#17724=EDGE_CURVE('',#14171,#14172,#7799,.T.);
#17725=EDGE_CURVE('',#14172,#14170,#1089,.T.);
#17726=EDGE_CURVE('',#14173,#14171,#1090,.T.);
#17727=EDGE_CURVE('',#14173,#14174,#7800,.T.);
#17728=EDGE_CURVE('',#14174,#14172,#1091,.T.);
#17729=EDGE_CURVE('',#14160,#14173,#1092,.T.);
#17730=EDGE_CURVE('',#14162,#14174,#1093,.T.);
#17731=EDGE_CURVE('',#14175,#14176,#1094,.T.);
#17732=EDGE_CURVE('',#14175,#14177,#7801,.T.);
#17733=EDGE_CURVE('',#14177,#14178,#1095,.T.);
#17734=EDGE_CURVE('',#14176,#14178,#7802,.T.);
#17735=EDGE_CURVE('',#14179,#14175,#1096,.T.);
#17736=EDGE_CURVE('',#14179,#14180,#7803,.T.);
#17737=EDGE_CURVE('',#14180,#14177,#1097,.T.);
#17738=EDGE_CURVE('',#14181,#14179,#1098,.T.);
#17739=EDGE_CURVE('',#14181,#14182,#7804,.T.);
#17740=EDGE_CURVE('',#14182,#14180,#1099,.T.);
#17741=EDGE_CURVE('',#14183,#14181,#1100,.T.);
#17742=EDGE_CURVE('',#14183,#14184,#7805,.T.);
#17743=EDGE_CURVE('',#14184,#14182,#1101,.T.);
#17744=EDGE_CURVE('',#14185,#14183,#1102,.T.);
#17745=EDGE_CURVE('',#14185,#14186,#7806,.T.);
#17746=EDGE_CURVE('',#14186,#14184,#1103,.T.);
#17747=EDGE_CURVE('',#14187,#14185,#1104,.T.);
#17748=EDGE_CURVE('',#14187,#14188,#7807,.T.);
#17749=EDGE_CURVE('',#14188,#14186,#1105,.T.);
#17750=EDGE_CURVE('',#14189,#14187,#1106,.T.);
#17751=EDGE_CURVE('',#14189,#14190,#7808,.T.);
#17752=EDGE_CURVE('',#14190,#14188,#1107,.T.);
#17753=EDGE_CURVE('',#14191,#14189,#1108,.T.);
#17754=EDGE_CURVE('',#14191,#14192,#7809,.T.);
#17755=EDGE_CURVE('',#14192,#14190,#1109,.T.);
#17756=EDGE_CURVE('',#14193,#14191,#1110,.T.);
#17757=EDGE_CURVE('',#14193,#14194,#7810,.T.);
#17758=EDGE_CURVE('',#14194,#14192,#1111,.T.);
#17759=EDGE_CURVE('',#14195,#14193,#1112,.T.);
#17760=EDGE_CURVE('',#14195,#14196,#7811,.T.);
#17761=EDGE_CURVE('',#14196,#14194,#1113,.T.);
#17762=EDGE_CURVE('',#14197,#14195,#1114,.T.);
#17763=EDGE_CURVE('',#14197,#14198,#7812,.T.);
#17764=EDGE_CURVE('',#14198,#14196,#1115,.T.);
#17765=EDGE_CURVE('',#14176,#14197,#1116,.T.);
#17766=EDGE_CURVE('',#14178,#14198,#1117,.T.);
#17767=EDGE_CURVE('',#14199,#14200,#1118,.T.);
#17768=EDGE_CURVE('',#14199,#14201,#7813,.T.);
#17769=EDGE_CURVE('',#14201,#14202,#1119,.T.);
#17770=EDGE_CURVE('',#14200,#14202,#7814,.T.);
#17771=EDGE_CURVE('',#14203,#14199,#1120,.T.);
#17772=EDGE_CURVE('',#14203,#14204,#7815,.T.);
#17773=EDGE_CURVE('',#14204,#14201,#1121,.T.);
#17774=EDGE_CURVE('',#14205,#14203,#1122,.T.);
#17775=EDGE_CURVE('',#14205,#14206,#7816,.T.);
#17776=EDGE_CURVE('',#14206,#14204,#1123,.T.);
#17777=EDGE_CURVE('',#14207,#14205,#1124,.T.);
#17778=EDGE_CURVE('',#14207,#14208,#7817,.T.);
#17779=EDGE_CURVE('',#14208,#14206,#1125,.T.);
#17780=EDGE_CURVE('',#14209,#14207,#1126,.T.);
#17781=EDGE_CURVE('',#14209,#14210,#7818,.T.);
#17782=EDGE_CURVE('',#14210,#14208,#1127,.T.);
#17783=EDGE_CURVE('',#14211,#14209,#1128,.T.);
#17784=EDGE_CURVE('',#14211,#14212,#7819,.T.);
#17785=EDGE_CURVE('',#14212,#14210,#1129,.T.);
#17786=EDGE_CURVE('',#14213,#14211,#1130,.T.);
#17787=EDGE_CURVE('',#14213,#14214,#7820,.T.);
#17788=EDGE_CURVE('',#14214,#14212,#1131,.T.);
#17789=EDGE_CURVE('',#14200,#14213,#1132,.T.);
#17790=EDGE_CURVE('',#14202,#14214,#1133,.T.);
#17791=EDGE_CURVE('',#14215,#14216,#1134,.T.);
#17792=EDGE_CURVE('',#14215,#14217,#7821,.T.);
#17793=EDGE_CURVE('',#14217,#14218,#1135,.T.);
#17794=EDGE_CURVE('',#14216,#14218,#7822,.T.);
#17795=EDGE_CURVE('',#14219,#14215,#1136,.T.);
#17796=EDGE_CURVE('',#14219,#14220,#7823,.T.);
#17797=EDGE_CURVE('',#14220,#14217,#1137,.T.);
#17798=EDGE_CURVE('',#14221,#14219,#1138,.T.);
#17799=EDGE_CURVE('',#14221,#14222,#7824,.T.);
#17800=EDGE_CURVE('',#14222,#14220,#1139,.T.);
#17801=EDGE_CURVE('',#14223,#14221,#1140,.T.);
#17802=EDGE_CURVE('',#14223,#14224,#7825,.T.);
#17803=EDGE_CURVE('',#14224,#14222,#1141,.T.);
#17804=EDGE_CURVE('',#14225,#14223,#1142,.T.);
#17805=EDGE_CURVE('',#14225,#14226,#7826,.T.);
#17806=EDGE_CURVE('',#14226,#14224,#1143,.T.);
#17807=EDGE_CURVE('',#14227,#14225,#1144,.T.);
#17808=EDGE_CURVE('',#14227,#14228,#7827,.T.);
#17809=EDGE_CURVE('',#14228,#14226,#1145,.T.);
#17810=EDGE_CURVE('',#14229,#14227,#1146,.T.);
#17811=EDGE_CURVE('',#14229,#14230,#7828,.T.);
#17812=EDGE_CURVE('',#14230,#14228,#1147,.T.);
#17813=EDGE_CURVE('',#14231,#14229,#1148,.T.);
#17814=EDGE_CURVE('',#14231,#14232,#7829,.T.);
#17815=EDGE_CURVE('',#14232,#14230,#1149,.T.);
#17816=EDGE_CURVE('',#14233,#14231,#1150,.T.);
#17817=EDGE_CURVE('',#14233,#14234,#7830,.T.);
#17818=EDGE_CURVE('',#14234,#14232,#1151,.T.);
#17819=EDGE_CURVE('',#14235,#14233,#1152,.T.);
#17820=EDGE_CURVE('',#14235,#14236,#7831,.T.);
#17821=EDGE_CURVE('',#14236,#14234,#1153,.T.);
#17822=EDGE_CURVE('',#14237,#14235,#1154,.T.);
#17823=EDGE_CURVE('',#14237,#14238,#7832,.T.);
#17824=EDGE_CURVE('',#14238,#14236,#1155,.T.);
#17825=EDGE_CURVE('',#14216,#14237,#1156,.T.);
#17826=EDGE_CURVE('',#14218,#14238,#1157,.T.);
#17827=EDGE_CURVE('',#14239,#14240,#7833,.T.);
#17828=EDGE_CURVE('',#14239,#14241,#7834,.T.);
#17829=EDGE_CURVE('',#14241,#14242,#7835,.T.);
#17830=EDGE_CURVE('',#14240,#14242,#7836,.T.);
#17831=EDGE_CURVE('',#14243,#14239,#1158,.T.);
#17832=EDGE_CURVE('',#14243,#14244,#7837,.T.);
#17833=EDGE_CURVE('',#14244,#14241,#1159,.T.);
#17834=EDGE_CURVE('',#14245,#14243,#1160,.T.);
#17835=EDGE_CURVE('',#14245,#14246,#7838,.T.);
#17836=EDGE_CURVE('',#14246,#14244,#1161,.T.);
#17837=EDGE_CURVE('',#14247,#14245,#7839,.T.);
#17838=EDGE_CURVE('',#14247,#14248,#7840,.T.);
#17839=EDGE_CURVE('',#14248,#14246,#7841,.T.);
#17840=EDGE_CURVE('',#14249,#14247,#1162,.T.);
#17841=EDGE_CURVE('',#14249,#14250,#7842,.T.);
#17842=EDGE_CURVE('',#14250,#14248,#1163,.T.);
#17843=EDGE_CURVE('',#14251,#14249,#1164,.T.);
#17844=EDGE_CURVE('',#14251,#14252,#7843,.T.);
#17845=EDGE_CURVE('',#14252,#14250,#1165,.T.);
#17846=EDGE_CURVE('',#14253,#14251,#7844,.T.);
#17847=EDGE_CURVE('',#14253,#14254,#7845,.T.);
#17848=EDGE_CURVE('',#14254,#14252,#7846,.T.);
#17849=EDGE_CURVE('',#14255,#14253,#7847,.T.);
#17850=EDGE_CURVE('',#14255,#14256,#7848,.T.);
#17851=EDGE_CURVE('',#14256,#14254,#7849,.T.);
#17852=EDGE_CURVE('',#14240,#14255,#7850,.T.);
#17853=EDGE_CURVE('',#14242,#14256,#7851,.T.);
#17854=EDGE_CURVE('',#14257,#14258,#1166,.T.);
#17855=EDGE_CURVE('',#14257,#14259,#7852,.T.);
#17856=EDGE_CURVE('',#14259,#14260,#1167,.T.);
#17857=EDGE_CURVE('',#14258,#14260,#7853,.T.);
#17858=EDGE_CURVE('',#14261,#14257,#1168,.T.);
#17859=EDGE_CURVE('',#14261,#14262,#7854,.T.);
#17860=EDGE_CURVE('',#14262,#14259,#1169,.T.);
#17861=EDGE_CURVE('',#14263,#14261,#1170,.T.);
#17862=EDGE_CURVE('',#14263,#14264,#7855,.T.);
#17863=EDGE_CURVE('',#14264,#14262,#1171,.T.);
#17864=EDGE_CURVE('',#14265,#14263,#1172,.T.);
#17865=EDGE_CURVE('',#14265,#14266,#7856,.T.);
#17866=EDGE_CURVE('',#14266,#14264,#1173,.T.);
#17867=EDGE_CURVE('',#14267,#14265,#1174,.T.);
#17868=EDGE_CURVE('',#14267,#14268,#7857,.T.);
#17869=EDGE_CURVE('',#14268,#14266,#1175,.T.);
#17870=EDGE_CURVE('',#14269,#14267,#1176,.T.);
#17871=EDGE_CURVE('',#14269,#14270,#7858,.T.);
#17872=EDGE_CURVE('',#14270,#14268,#1177,.T.);
#17873=EDGE_CURVE('',#14271,#14269,#1178,.T.);
#17874=EDGE_CURVE('',#14271,#14272,#7859,.T.);
#17875=EDGE_CURVE('',#14272,#14270,#1179,.T.);
#17876=EDGE_CURVE('',#14258,#14271,#1180,.T.);
#17877=EDGE_CURVE('',#14260,#14272,#1181,.T.);
#17878=EDGE_CURVE('',#14273,#14274,#1182,.T.);
#17879=EDGE_CURVE('',#14273,#14275,#7860,.T.);
#17880=EDGE_CURVE('',#14275,#14276,#1183,.T.);
#17881=EDGE_CURVE('',#14274,#14276,#7861,.T.);
#17882=EDGE_CURVE('',#14277,#14273,#1184,.T.);
#17883=EDGE_CURVE('',#14277,#14278,#7862,.T.);
#17884=EDGE_CURVE('',#14278,#14275,#1185,.T.);
#17885=EDGE_CURVE('',#14279,#14277,#1186,.T.);
#17886=EDGE_CURVE('',#14279,#14280,#7863,.T.);
#17887=EDGE_CURVE('',#14280,#14278,#1187,.T.);
#17888=EDGE_CURVE('',#14281,#14279,#1188,.T.);
#17889=EDGE_CURVE('',#14281,#14282,#7864,.T.);
#17890=EDGE_CURVE('',#14282,#14280,#1189,.T.);
#17891=EDGE_CURVE('',#14283,#14281,#1190,.T.);
#17892=EDGE_CURVE('',#14283,#14284,#7865,.T.);
#17893=EDGE_CURVE('',#14284,#14282,#1191,.T.);
#17894=EDGE_CURVE('',#14285,#14283,#1192,.T.);
#17895=EDGE_CURVE('',#14285,#14286,#7866,.T.);
#17896=EDGE_CURVE('',#14286,#14284,#1193,.T.);
#17897=EDGE_CURVE('',#14287,#14285,#1194,.T.);
#17898=EDGE_CURVE('',#14287,#14288,#7867,.T.);
#17899=EDGE_CURVE('',#14288,#14286,#1195,.T.);
#17900=EDGE_CURVE('',#14289,#14287,#1196,.T.);
#17901=EDGE_CURVE('',#14289,#14290,#7868,.T.);
#17902=EDGE_CURVE('',#14290,#14288,#1197,.T.);
#17903=EDGE_CURVE('',#14291,#14289,#1198,.T.);
#17904=EDGE_CURVE('',#14291,#14292,#7869,.T.);
#17905=EDGE_CURVE('',#14292,#14290,#1199,.T.);
#17906=EDGE_CURVE('',#14293,#14291,#1200,.T.);
#17907=EDGE_CURVE('',#14293,#14294,#7870,.T.);
#17908=EDGE_CURVE('',#14294,#14292,#1201,.T.);
#17909=EDGE_CURVE('',#14295,#14293,#1202,.T.);
#17910=EDGE_CURVE('',#14295,#14296,#7871,.T.);
#17911=EDGE_CURVE('',#14296,#14294,#1203,.T.);
#17912=EDGE_CURVE('',#14274,#14295,#1204,.T.);
#17913=EDGE_CURVE('',#14276,#14296,#1205,.T.);
#17914=EDGE_CURVE('',#14297,#14298,#1206,.T.);
#17915=EDGE_CURVE('',#14297,#14299,#7872,.T.);
#17916=EDGE_CURVE('',#14299,#14300,#1207,.T.);
#17917=EDGE_CURVE('',#14298,#14300,#7873,.T.);
#17918=EDGE_CURVE('',#14301,#14297,#1208,.T.);
#17919=EDGE_CURVE('',#14301,#14302,#7874,.T.);
#17920=EDGE_CURVE('',#14302,#14299,#1209,.T.);
#17921=EDGE_CURVE('',#14303,#14301,#1210,.T.);
#17922=EDGE_CURVE('',#14303,#14304,#7875,.T.);
#17923=EDGE_CURVE('',#14304,#14302,#1211,.T.);
#17924=EDGE_CURVE('',#14305,#14303,#1212,.T.);
#17925=EDGE_CURVE('',#14305,#14306,#7876,.T.);
#17926=EDGE_CURVE('',#14306,#14304,#1213,.T.);
#17927=EDGE_CURVE('',#14307,#14305,#1214,.T.);
#17928=EDGE_CURVE('',#14307,#14308,#7877,.T.);
#17929=EDGE_CURVE('',#14308,#14306,#1215,.T.);
#17930=EDGE_CURVE('',#14309,#14307,#1216,.T.);
#17931=EDGE_CURVE('',#14309,#14310,#7878,.T.);
#17932=EDGE_CURVE('',#14310,#14308,#1217,.T.);
#17933=EDGE_CURVE('',#14311,#14309,#1218,.T.);
#17934=EDGE_CURVE('',#14311,#14312,#7879,.T.);
#17935=EDGE_CURVE('',#14312,#14310,#1219,.T.);
#17936=EDGE_CURVE('',#14313,#14311,#1220,.T.);
#17937=EDGE_CURVE('',#14313,#14314,#7880,.T.);
#17938=EDGE_CURVE('',#14314,#14312,#1221,.T.);
#17939=EDGE_CURVE('',#14315,#14313,#1222,.T.);
#17940=EDGE_CURVE('',#14315,#14316,#7881,.T.);
#17941=EDGE_CURVE('',#14316,#14314,#1223,.T.);
#17942=EDGE_CURVE('',#14317,#14315,#7882,.T.);
#17943=EDGE_CURVE('',#14317,#14318,#7883,.T.);
#17944=EDGE_CURVE('',#14318,#14316,#7884,.T.);
#17945=EDGE_CURVE('',#14319,#14317,#1224,.T.);
#17946=EDGE_CURVE('',#14319,#14320,#7885,.T.);
#17947=EDGE_CURVE('',#14320,#14318,#1225,.T.);
#17948=EDGE_CURVE('',#14321,#14319,#1226,.T.);
#17949=EDGE_CURVE('',#14321,#14322,#7886,.T.);
#17950=EDGE_CURVE('',#14322,#14320,#1227,.T.);
#17951=EDGE_CURVE('',#14323,#14321,#1228,.T.);
#17952=EDGE_CURVE('',#14323,#14324,#7887,.T.);
#17953=EDGE_CURVE('',#14324,#14322,#1229,.T.);
#17954=EDGE_CURVE('',#14325,#14323,#1230,.T.);
#17955=EDGE_CURVE('',#14325,#14326,#7888,.T.);
#17956=EDGE_CURVE('',#14326,#14324,#1231,.T.);
#17957=EDGE_CURVE('',#14327,#14325,#1232,.T.);
#17958=EDGE_CURVE('',#14327,#14328,#7889,.T.);
#17959=EDGE_CURVE('',#14328,#14326,#1233,.T.);
#17960=EDGE_CURVE('',#14329,#14327,#1234,.T.);
#17961=EDGE_CURVE('',#14329,#14330,#7890,.T.);
#17962=EDGE_CURVE('',#14330,#14328,#1235,.T.);
#17963=EDGE_CURVE('',#14331,#14329,#1236,.T.);
#17964=EDGE_CURVE('',#14331,#14332,#7891,.T.);
#17965=EDGE_CURVE('',#14332,#14330,#1237,.T.);
#17966=EDGE_CURVE('',#14333,#14331,#1238,.T.);
#17967=EDGE_CURVE('',#14333,#14334,#7892,.T.);
#17968=EDGE_CURVE('',#14334,#14332,#1239,.T.);
#17969=EDGE_CURVE('',#14335,#14333,#1240,.T.);
#17970=EDGE_CURVE('',#14335,#14336,#7893,.T.);
#17971=EDGE_CURVE('',#14336,#14334,#1241,.T.);
#17972=EDGE_CURVE('',#14337,#14335,#7894,.T.);
#17973=EDGE_CURVE('',#14337,#14338,#7895,.T.);
#17974=EDGE_CURVE('',#14338,#14336,#7896,.T.);
#17975=EDGE_CURVE('',#14339,#14337,#7897,.T.);
#17976=EDGE_CURVE('',#14339,#14340,#7898,.T.);
#17977=EDGE_CURVE('',#14340,#14338,#7899,.T.);
#17978=EDGE_CURVE('',#14298,#14339,#7900,.T.);
#17979=EDGE_CURVE('',#14300,#14340,#7901,.T.);
#17980=EDGE_CURVE('',#14341,#14342,#1242,.T.);
#17981=EDGE_CURVE('',#14341,#14343,#7902,.T.);
#17982=EDGE_CURVE('',#14343,#14344,#1243,.T.);
#17983=EDGE_CURVE('',#14342,#14344,#7903,.T.);
#17984=EDGE_CURVE('',#14345,#14341,#1244,.T.);
#17985=EDGE_CURVE('',#14345,#14346,#7904,.T.);
#17986=EDGE_CURVE('',#14346,#14343,#1245,.T.);
#17987=EDGE_CURVE('',#14347,#14345,#1246,.T.);
#17988=EDGE_CURVE('',#14347,#14348,#7905,.T.);
#17989=EDGE_CURVE('',#14348,#14346,#1247,.T.);
#17990=EDGE_CURVE('',#14349,#14347,#1248,.T.);
#17991=EDGE_CURVE('',#14349,#14350,#7906,.T.);
#17992=EDGE_CURVE('',#14350,#14348,#1249,.T.);
#17993=EDGE_CURVE('',#14351,#14349,#1250,.T.);
#17994=EDGE_CURVE('',#14351,#14352,#7907,.T.);
#17995=EDGE_CURVE('',#14352,#14350,#1251,.T.);
#17996=EDGE_CURVE('',#14353,#14351,#1252,.T.);
#17997=EDGE_CURVE('',#14353,#14354,#7908,.T.);
#17998=EDGE_CURVE('',#14354,#14352,#1253,.T.);
#17999=EDGE_CURVE('',#14355,#14353,#1254,.T.);
#18000=EDGE_CURVE('',#14355,#14356,#7909,.T.);
#18001=EDGE_CURVE('',#14356,#14354,#1255,.T.);
#18002=EDGE_CURVE('',#14342,#14355,#1256,.T.);
#18003=EDGE_CURVE('',#14344,#14356,#1257,.T.);
#18004=EDGE_CURVE('',#14357,#14358,#1258,.T.);
#18005=EDGE_CURVE('',#14357,#14359,#7910,.T.);
#18006=EDGE_CURVE('',#14359,#14360,#1259,.T.);
#18007=EDGE_CURVE('',#14358,#14360,#7911,.T.);
#18008=EDGE_CURVE('',#14361,#14357,#1260,.T.);
#18009=EDGE_CURVE('',#14361,#14362,#7912,.T.);
#18010=EDGE_CURVE('',#14362,#14359,#1261,.T.);
#18011=EDGE_CURVE('',#14363,#14361,#1262,.T.);
#18012=EDGE_CURVE('',#14363,#14364,#7913,.T.);
#18013=EDGE_CURVE('',#14364,#14362,#1263,.T.);
#18014=EDGE_CURVE('',#14365,#14363,#1264,.T.);
#18015=EDGE_CURVE('',#14365,#14366,#7914,.T.);
#18016=EDGE_CURVE('',#14366,#14364,#1265,.T.);
#18017=EDGE_CURVE('',#14367,#14365,#1266,.T.);
#18018=EDGE_CURVE('',#14367,#14368,#7915,.T.);
#18019=EDGE_CURVE('',#14368,#14366,#1267,.T.);
#18020=EDGE_CURVE('',#14369,#14367,#1268,.T.);
#18021=EDGE_CURVE('',#14369,#14370,#7916,.T.);
#18022=EDGE_CURVE('',#14370,#14368,#1269,.T.);
#18023=EDGE_CURVE('',#14371,#14369,#1270,.T.);
#18024=EDGE_CURVE('',#14371,#14372,#7917,.T.);
#18025=EDGE_CURVE('',#14372,#14370,#1271,.T.);
#18026=EDGE_CURVE('',#14373,#14371,#1272,.T.);
#18027=EDGE_CURVE('',#14373,#14374,#7918,.T.);
#18028=EDGE_CURVE('',#14374,#14372,#1273,.T.);
#18029=EDGE_CURVE('',#14375,#14373,#1274,.T.);
#18030=EDGE_CURVE('',#14375,#14376,#7919,.T.);
#18031=EDGE_CURVE('',#14376,#14374,#1275,.T.);
#18032=EDGE_CURVE('',#14377,#14375,#1276,.T.);
#18033=EDGE_CURVE('',#14377,#14378,#7920,.T.);
#18034=EDGE_CURVE('',#14378,#14376,#1277,.T.);
#18035=EDGE_CURVE('',#14379,#14377,#1278,.T.);
#18036=EDGE_CURVE('',#14379,#14380,#7921,.T.);
#18037=EDGE_CURVE('',#14380,#14378,#1279,.T.);
#18038=EDGE_CURVE('',#14358,#14379,#1280,.T.);
#18039=EDGE_CURVE('',#14360,#14380,#1281,.T.);
#18040=EDGE_CURVE('',#14381,#14382,#1282,.T.);
#18041=EDGE_CURVE('',#14381,#14383,#7922,.T.);
#18042=EDGE_CURVE('',#14383,#14384,#1283,.T.);
#18043=EDGE_CURVE('',#14382,#14384,#7923,.T.);
#18044=EDGE_CURVE('',#14385,#14381,#1284,.T.);
#18045=EDGE_CURVE('',#14385,#14386,#7924,.T.);
#18046=EDGE_CURVE('',#14386,#14383,#1285,.T.);
#18047=EDGE_CURVE('',#14387,#14385,#1286,.T.);
#18048=EDGE_CURVE('',#14387,#14388,#7925,.T.);
#18049=EDGE_CURVE('',#14388,#14386,#1287,.T.);
#18050=EDGE_CURVE('',#14389,#14387,#1288,.T.);
#18051=EDGE_CURVE('',#14389,#14390,#7926,.T.);
#18052=EDGE_CURVE('',#14390,#14388,#1289,.T.);
#18053=EDGE_CURVE('',#14391,#14389,#1290,.T.);
#18054=EDGE_CURVE('',#14391,#14392,#7927,.T.);
#18055=EDGE_CURVE('',#14392,#14390,#1291,.T.);
#18056=EDGE_CURVE('',#14393,#14391,#1292,.T.);
#18057=EDGE_CURVE('',#14393,#14394,#7928,.T.);
#18058=EDGE_CURVE('',#14394,#14392,#1293,.T.);
#18059=EDGE_CURVE('',#14395,#14393,#1294,.T.);
#18060=EDGE_CURVE('',#14395,#14396,#7929,.T.);
#18061=EDGE_CURVE('',#14396,#14394,#1295,.T.);
#18062=EDGE_CURVE('',#14397,#14395,#1296,.T.);
#18063=EDGE_CURVE('',#14397,#14398,#7930,.T.);
#18064=EDGE_CURVE('',#14398,#14396,#1297,.T.);
#18065=EDGE_CURVE('',#14399,#14397,#1298,.T.);
#18066=EDGE_CURVE('',#14399,#14400,#7931,.T.);
#18067=EDGE_CURVE('',#14400,#14398,#1299,.T.);
#18068=EDGE_CURVE('',#14401,#14399,#1300,.T.);
#18069=EDGE_CURVE('',#14401,#14402,#7932,.T.);
#18070=EDGE_CURVE('',#14402,#14400,#1301,.T.);
#18071=EDGE_CURVE('',#14403,#14401,#1302,.T.);
#18072=EDGE_CURVE('',#14403,#14404,#7933,.T.);
#18073=EDGE_CURVE('',#14404,#14402,#1303,.T.);
#18074=EDGE_CURVE('',#14405,#14403,#1304,.T.);
#18075=EDGE_CURVE('',#14405,#14406,#7934,.T.);
#18076=EDGE_CURVE('',#14406,#14404,#1305,.T.);
#18077=EDGE_CURVE('',#14407,#14405,#7935,.T.);
#18078=EDGE_CURVE('',#14407,#14408,#7936,.T.);
#18079=EDGE_CURVE('',#14408,#14406,#7937,.T.);
#18080=EDGE_CURVE('',#14409,#14407,#1306,.T.);
#18081=EDGE_CURVE('',#14409,#14410,#7938,.T.);
#18082=EDGE_CURVE('',#14410,#14408,#1307,.T.);
#18083=EDGE_CURVE('',#14411,#14409,#1308,.T.);
#18084=EDGE_CURVE('',#14411,#14412,#7939,.T.);
#18085=EDGE_CURVE('',#14412,#14410,#1309,.T.);
#18086=EDGE_CURVE('',#14413,#14411,#1310,.T.);
#18087=EDGE_CURVE('',#14413,#14414,#7940,.T.);
#18088=EDGE_CURVE('',#14414,#14412,#1311,.T.);
#18089=EDGE_CURVE('',#14415,#14413,#1312,.T.);
#18090=EDGE_CURVE('',#14415,#14416,#7941,.T.);
#18091=EDGE_CURVE('',#14416,#14414,#1313,.T.);
#18092=EDGE_CURVE('',#14417,#14415,#1314,.T.);
#18093=EDGE_CURVE('',#14417,#14418,#7942,.T.);
#18094=EDGE_CURVE('',#14418,#14416,#1315,.T.);
#18095=EDGE_CURVE('',#14419,#14417,#1316,.T.);
#18096=EDGE_CURVE('',#14419,#14420,#7943,.T.);
#18097=EDGE_CURVE('',#14420,#14418,#1317,.T.);
#18098=EDGE_CURVE('',#14421,#14419,#1318,.T.);
#18099=EDGE_CURVE('',#14421,#14422,#7944,.T.);
#18100=EDGE_CURVE('',#14422,#14420,#1319,.T.);
#18101=EDGE_CURVE('',#14423,#14421,#7945,.T.);
#18102=EDGE_CURVE('',#14423,#14424,#7946,.T.);
#18103=EDGE_CURVE('',#14424,#14422,#7947,.T.);
#18104=EDGE_CURVE('',#14425,#14423,#1320,.T.);
#18105=EDGE_CURVE('',#14425,#14426,#7948,.T.);
#18106=EDGE_CURVE('',#14426,#14424,#1321,.T.);
#18107=EDGE_CURVE('',#14427,#14425,#1322,.T.);
#18108=EDGE_CURVE('',#14427,#14428,#7949,.T.);
#18109=EDGE_CURVE('',#14428,#14426,#1323,.T.);
#18110=EDGE_CURVE('',#14429,#14427,#1324,.T.);
#18111=EDGE_CURVE('',#14429,#14430,#7950,.T.);
#18112=EDGE_CURVE('',#14430,#14428,#1325,.T.);
#18113=EDGE_CURVE('',#14431,#14429,#1326,.T.);
#18114=EDGE_CURVE('',#14431,#14432,#7951,.T.);
#18115=EDGE_CURVE('',#14432,#14430,#1327,.T.);
#18116=EDGE_CURVE('',#14433,#14431,#1328,.T.);
#18117=EDGE_CURVE('',#14433,#14434,#7952,.T.);
#18118=EDGE_CURVE('',#14434,#14432,#1329,.T.);
#18119=EDGE_CURVE('',#14435,#14433,#1330,.T.);
#18120=EDGE_CURVE('',#14435,#14436,#7953,.T.);
#18121=EDGE_CURVE('',#14436,#14434,#1331,.T.);
#18122=EDGE_CURVE('',#14437,#14435,#1332,.T.);
#18123=EDGE_CURVE('',#14437,#14438,#7954,.T.);
#18124=EDGE_CURVE('',#14438,#14436,#1333,.T.);
#18125=EDGE_CURVE('',#14439,#14437,#7955,.T.);
#18126=EDGE_CURVE('',#14439,#14440,#7956,.T.);
#18127=EDGE_CURVE('',#14440,#14438,#7957,.T.);
#18128=EDGE_CURVE('',#14382,#14439,#1334,.T.);
#18129=EDGE_CURVE('',#14384,#14440,#1335,.T.);
#18130=EDGE_CURVE('',#14441,#14442,#1336,.T.);
#18131=EDGE_CURVE('',#14441,#14443,#7958,.T.);
#18132=EDGE_CURVE('',#14443,#14444,#1337,.T.);
#18133=EDGE_CURVE('',#14442,#14444,#7959,.T.);
#18134=EDGE_CURVE('',#14445,#14441,#1338,.T.);
#18135=EDGE_CURVE('',#14445,#14446,#7960,.T.);
#18136=EDGE_CURVE('',#14446,#14443,#1339,.T.);
#18137=EDGE_CURVE('',#14447,#14445,#1340,.T.);
#18138=EDGE_CURVE('',#14447,#14448,#7961,.T.);
#18139=EDGE_CURVE('',#14448,#14446,#1341,.T.);
#18140=EDGE_CURVE('',#14449,#14447,#1342,.T.);
#18141=EDGE_CURVE('',#14449,#14450,#7962,.T.);
#18142=EDGE_CURVE('',#14450,#14448,#1343,.T.);
#18143=EDGE_CURVE('',#14451,#14449,#1344,.T.);
#18144=EDGE_CURVE('',#14451,#14452,#7963,.T.);
#18145=EDGE_CURVE('',#14452,#14450,#1345,.T.);
#18146=EDGE_CURVE('',#14453,#14451,#1346,.T.);
#18147=EDGE_CURVE('',#14453,#14454,#7964,.T.);
#18148=EDGE_CURVE('',#14454,#14452,#1347,.T.);
#18149=EDGE_CURVE('',#14455,#14453,#1348,.T.);
#18150=EDGE_CURVE('',#14455,#14456,#7965,.T.);
#18151=EDGE_CURVE('',#14456,#14454,#1349,.T.);
#18152=EDGE_CURVE('',#14442,#14455,#1350,.T.);
#18153=EDGE_CURVE('',#14444,#14456,#1351,.T.);
#18154=EDGE_CURVE('',#14457,#14458,#1352,.T.);
#18155=EDGE_CURVE('',#14457,#14459,#7966,.T.);
#18156=EDGE_CURVE('',#14459,#14460,#1353,.T.);
#18157=EDGE_CURVE('',#14458,#14460,#7967,.T.);
#18158=EDGE_CURVE('',#14461,#14457,#1354,.T.);
#18159=EDGE_CURVE('',#14461,#14462,#7968,.T.);
#18160=EDGE_CURVE('',#14462,#14459,#1355,.T.);
#18161=EDGE_CURVE('',#14463,#14461,#1356,.T.);
#18162=EDGE_CURVE('',#14463,#14464,#7969,.T.);
#18163=EDGE_CURVE('',#14464,#14462,#1357,.T.);
#18164=EDGE_CURVE('',#14465,#14463,#1358,.T.);
#18165=EDGE_CURVE('',#14465,#14466,#7970,.T.);
#18166=EDGE_CURVE('',#14466,#14464,#1359,.T.);
#18167=EDGE_CURVE('',#14467,#14465,#1360,.T.);
#18168=EDGE_CURVE('',#14467,#14468,#7971,.T.);
#18169=EDGE_CURVE('',#14468,#14466,#1361,.T.);
#18170=EDGE_CURVE('',#14469,#14467,#1362,.T.);
#18171=EDGE_CURVE('',#14469,#14470,#7972,.T.);
#18172=EDGE_CURVE('',#14470,#14468,#1363,.T.);
#18173=EDGE_CURVE('',#14471,#14469,#1364,.T.);
#18174=EDGE_CURVE('',#14471,#14472,#7973,.T.);
#18175=EDGE_CURVE('',#14472,#14470,#1365,.T.);
#18176=EDGE_CURVE('',#14473,#14471,#1366,.T.);
#18177=EDGE_CURVE('',#14473,#14474,#7974,.T.);
#18178=EDGE_CURVE('',#14474,#14472,#1367,.T.);
#18179=EDGE_CURVE('',#14475,#14473,#1368,.T.);
#18180=EDGE_CURVE('',#14475,#14476,#7975,.T.);
#18181=EDGE_CURVE('',#14476,#14474,#1369,.T.);
#18182=EDGE_CURVE('',#14477,#14475,#1370,.T.);
#18183=EDGE_CURVE('',#14477,#14478,#7976,.T.);
#18184=EDGE_CURVE('',#14478,#14476,#1371,.T.);
#18185=EDGE_CURVE('',#14479,#14477,#1372,.T.);
#18186=EDGE_CURVE('',#14479,#14480,#7977,.T.);
#18187=EDGE_CURVE('',#14480,#14478,#1373,.T.);
#18188=EDGE_CURVE('',#14458,#14479,#1374,.T.);
#18189=EDGE_CURVE('',#14460,#14480,#1375,.T.);
#18190=EDGE_CURVE('',#14481,#14482,#7978,.T.);
#18191=EDGE_CURVE('',#14481,#14483,#7979,.T.);
#18192=EDGE_CURVE('',#14483,#14484,#7980,.T.);
#18193=EDGE_CURVE('',#14482,#14484,#7981,.T.);
#18194=EDGE_CURVE('',#14485,#14481,#7982,.T.);
#18195=EDGE_CURVE('',#14485,#14486,#7983,.T.);
#18196=EDGE_CURVE('',#14486,#14483,#7984,.T.);
#18197=EDGE_CURVE('',#14482,#14485,#7985,.T.);
#18198=EDGE_CURVE('',#14484,#14486,#7986,.T.);
#18199=EDGE_CURVE('',#14487,#14488,#7987,.T.);
#18200=EDGE_CURVE('',#14487,#14489,#7988,.T.);
#18201=EDGE_CURVE('',#14489,#14490,#7989,.T.);
#18202=EDGE_CURVE('',#14488,#14490,#7990,.T.);
#18203=EDGE_CURVE('',#14491,#14487,#7991,.T.);
#18204=EDGE_CURVE('',#14491,#14492,#7992,.T.);
#18205=EDGE_CURVE('',#14492,#14489,#7993,.T.);
#18206=EDGE_CURVE('',#14493,#14491,#7994,.T.);
#18207=EDGE_CURVE('',#14493,#14494,#7995,.T.);
#18208=EDGE_CURVE('',#14494,#14492,#7996,.T.);
#18209=EDGE_CURVE('',#14495,#14493,#7997,.T.);
#18210=EDGE_CURVE('',#14495,#14496,#7998,.T.);
#18211=EDGE_CURVE('',#14496,#14494,#7999,.T.);
#18212=EDGE_CURVE('',#14497,#14495,#8000,.T.);
#18213=EDGE_CURVE('',#14497,#14498,#8001,.T.);
#18214=EDGE_CURVE('',#14498,#14496,#8002,.T.);
#18215=EDGE_CURVE('',#14499,#14497,#8003,.T.);
#18216=EDGE_CURVE('',#14499,#14500,#8004,.T.);
#18217=EDGE_CURVE('',#14500,#14498,#8005,.T.);
#18218=EDGE_CURVE('',#14501,#14499,#8006,.T.);
#18219=EDGE_CURVE('',#14501,#14502,#8007,.T.);
#18220=EDGE_CURVE('',#14502,#14500,#8008,.T.);
#18221=EDGE_CURVE('',#14503,#14501,#8009,.T.);
#18222=EDGE_CURVE('',#14503,#14504,#8010,.T.);
#18223=EDGE_CURVE('',#14504,#14502,#8011,.T.);
#18224=EDGE_CURVE('',#14505,#14503,#8012,.T.);
#18225=EDGE_CURVE('',#14505,#14506,#8013,.T.);
#18226=EDGE_CURVE('',#14506,#14504,#8014,.T.);
#18227=EDGE_CURVE('',#14507,#14505,#8015,.T.);
#18228=EDGE_CURVE('',#14507,#14508,#8016,.T.);
#18229=EDGE_CURVE('',#14508,#14506,#8017,.T.);
#18230=EDGE_CURVE('',#14488,#14507,#8018,.T.);
#18231=EDGE_CURVE('',#14490,#14508,#8019,.T.);
#18232=EDGE_CURVE('',#14509,#14510,#8020,.T.);
#18233=EDGE_CURVE('',#14509,#14511,#8021,.T.);
#18234=EDGE_CURVE('',#14511,#14512,#8022,.T.);
#18235=EDGE_CURVE('',#14510,#14512,#8023,.T.);
#18236=EDGE_CURVE('',#14513,#14509,#8024,.T.);
#18237=EDGE_CURVE('',#14513,#14514,#8025,.T.);
#18238=EDGE_CURVE('',#14514,#14511,#8026,.T.);
#18239=EDGE_CURVE('',#14515,#14513,#8027,.T.);
#18240=EDGE_CURVE('',#14515,#14516,#8028,.T.);
#18241=EDGE_CURVE('',#14516,#14514,#8029,.T.);
#18242=EDGE_CURVE('',#14510,#14515,#8030,.T.);
#18243=EDGE_CURVE('',#14512,#14516,#8031,.T.);
#18244=EDGE_CURVE('',#14517,#14518,#8032,.T.);
#18245=EDGE_CURVE('',#14517,#14519,#8033,.T.);
#18246=EDGE_CURVE('',#14519,#14520,#8034,.T.);
#18247=EDGE_CURVE('',#14518,#14520,#8035,.T.);
#18248=EDGE_CURVE('',#14521,#14517,#8036,.T.);
#18249=EDGE_CURVE('',#14521,#14522,#8037,.T.);
#18250=EDGE_CURVE('',#14522,#14519,#8038,.T.);
#18251=EDGE_CURVE('',#14523,#14521,#8039,.T.);
#18252=EDGE_CURVE('',#14523,#14524,#8040,.T.);
#18253=EDGE_CURVE('',#14524,#14522,#8041,.T.);
#18254=EDGE_CURVE('',#14518,#14523,#8042,.T.);
#18255=EDGE_CURVE('',#14520,#14524,#8043,.T.);
#18256=EDGE_CURVE('',#14525,#14526,#8044,.T.);
#18257=EDGE_CURVE('',#14525,#14527,#8045,.T.);
#18258=EDGE_CURVE('',#14527,#14528,#8046,.T.);
#18259=EDGE_CURVE('',#14526,#14528,#8047,.T.);
#18260=EDGE_CURVE('',#14529,#14525,#8048,.T.);
#18261=EDGE_CURVE('',#14529,#14530,#8049,.T.);
#18262=EDGE_CURVE('',#14530,#14527,#8050,.T.);
#18263=EDGE_CURVE('',#14531,#14529,#8051,.T.);
#18264=EDGE_CURVE('',#14531,#14532,#8052,.T.);
#18265=EDGE_CURVE('',#14532,#14530,#8053,.T.);
#18266=EDGE_CURVE('',#14526,#14531,#8054,.T.);
#18267=EDGE_CURVE('',#14528,#14532,#8055,.T.);
#18268=EDGE_CURVE('',#14533,#14534,#8056,.T.);
#18269=EDGE_CURVE('',#14533,#14535,#8057,.T.);
#18270=EDGE_CURVE('',#14535,#14536,#8058,.T.);
#18271=EDGE_CURVE('',#14534,#14536,#8059,.T.);
#18272=EDGE_CURVE('',#14537,#14533,#8060,.T.);
#18273=EDGE_CURVE('',#14537,#14538,#8061,.T.);
#18274=EDGE_CURVE('',#14538,#14535,#8062,.T.);
#18275=EDGE_CURVE('',#14539,#14537,#8063,.T.);
#18276=EDGE_CURVE('',#14539,#14540,#8064,.T.);
#18277=EDGE_CURVE('',#14540,#14538,#8065,.T.);
#18278=EDGE_CURVE('',#14534,#14539,#8066,.T.);
#18279=EDGE_CURVE('',#14536,#14540,#8067,.T.);
#18280=EDGE_CURVE('',#14541,#14542,#8068,.T.);
#18281=EDGE_CURVE('',#14541,#14543,#8069,.T.);
#18282=EDGE_CURVE('',#14543,#14544,#8070,.T.);
#18283=EDGE_CURVE('',#14542,#14544,#8071,.T.);
#18284=EDGE_CURVE('',#14545,#14541,#8072,.T.);
#18285=EDGE_CURVE('',#14545,#14546,#8073,.T.);
#18286=EDGE_CURVE('',#14546,#14543,#8074,.T.);
#18287=EDGE_CURVE('',#14547,#14545,#8075,.T.);
#18288=EDGE_CURVE('',#14547,#14548,#8076,.T.);
#18289=EDGE_CURVE('',#14548,#14546,#8077,.T.);
#18290=EDGE_CURVE('',#14542,#14547,#8078,.T.);
#18291=EDGE_CURVE('',#14544,#14548,#8079,.T.);
#18292=EDGE_CURVE('',#14549,#14550,#8080,.T.);
#18293=EDGE_CURVE('',#14549,#14551,#8081,.T.);
#18294=EDGE_CURVE('',#14551,#14552,#8082,.T.);
#18295=EDGE_CURVE('',#14550,#14552,#8083,.T.);
#18296=EDGE_CURVE('',#14553,#14549,#8084,.T.);
#18297=EDGE_CURVE('',#14553,#14554,#8085,.T.);
#18298=EDGE_CURVE('',#14554,#14551,#8086,.T.);
#18299=EDGE_CURVE('',#14555,#14553,#8087,.T.);
#18300=EDGE_CURVE('',#14555,#14556,#8088,.T.);
#18301=EDGE_CURVE('',#14556,#14554,#8089,.T.);
#18302=EDGE_CURVE('',#14550,#14555,#8090,.T.);
#18303=EDGE_CURVE('',#14552,#14556,#8091,.T.);
#18304=EDGE_CURVE('',#14557,#14558,#8092,.T.);
#18305=EDGE_CURVE('',#14557,#14559,#8093,.T.);
#18306=EDGE_CURVE('',#14559,#14560,#8094,.T.);
#18307=EDGE_CURVE('',#14558,#14560,#8095,.T.);
#18308=EDGE_CURVE('',#14561,#14557,#8096,.T.);
#18309=EDGE_CURVE('',#14561,#14562,#8097,.T.);
#18310=EDGE_CURVE('',#14562,#14559,#8098,.T.);
#18311=EDGE_CURVE('',#14563,#14561,#8099,.T.);
#18312=EDGE_CURVE('',#14563,#14564,#8100,.T.);
#18313=EDGE_CURVE('',#14564,#14562,#8101,.T.);
#18314=EDGE_CURVE('',#14558,#14563,#8102,.T.);
#18315=EDGE_CURVE('',#14560,#14564,#8103,.T.);
#18316=EDGE_CURVE('',#14565,#14566,#8104,.T.);
#18317=EDGE_CURVE('',#14565,#14567,#8105,.T.);
#18318=EDGE_CURVE('',#14567,#14568,#8106,.T.);
#18319=EDGE_CURVE('',#14566,#14568,#8107,.T.);
#18320=EDGE_CURVE('',#14569,#14565,#8108,.T.);
#18321=EDGE_CURVE('',#14569,#14570,#8109,.T.);
#18322=EDGE_CURVE('',#14570,#14567,#8110,.T.);
#18323=EDGE_CURVE('',#14571,#14569,#8111,.T.);
#18324=EDGE_CURVE('',#14571,#14572,#8112,.T.);
#18325=EDGE_CURVE('',#14572,#14570,#8113,.T.);
#18326=EDGE_CURVE('',#14566,#14571,#8114,.T.);
#18327=EDGE_CURVE('',#14568,#14572,#8115,.T.);
#18328=EDGE_CURVE('',#14573,#14574,#8116,.T.);
#18329=EDGE_CURVE('',#14573,#14575,#8117,.T.);
#18330=EDGE_CURVE('',#14575,#14576,#8118,.T.);
#18331=EDGE_CURVE('',#14574,#14576,#8119,.T.);
#18332=EDGE_CURVE('',#14577,#14573,#8120,.T.);
#18333=EDGE_CURVE('',#14577,#14578,#8121,.T.);
#18334=EDGE_CURVE('',#14578,#14575,#8122,.T.);
#18335=EDGE_CURVE('',#14579,#14577,#8123,.T.);
#18336=EDGE_CURVE('',#14579,#14580,#8124,.T.);
#18337=EDGE_CURVE('',#14580,#14578,#8125,.T.);
#18338=EDGE_CURVE('',#14574,#14579,#8126,.T.);
#18339=EDGE_CURVE('',#14576,#14580,#8127,.T.);
#18340=EDGE_CURVE('',#14581,#14582,#8128,.T.);
#18341=EDGE_CURVE('',#14581,#14583,#8129,.T.);
#18342=EDGE_CURVE('',#14583,#14584,#8130,.T.);
#18343=EDGE_CURVE('',#14582,#14584,#8131,.T.);
#18344=EDGE_CURVE('',#14585,#14581,#8132,.T.);
#18345=EDGE_CURVE('',#14585,#14586,#8133,.T.);
#18346=EDGE_CURVE('',#14586,#14583,#8134,.T.);
#18347=EDGE_CURVE('',#14587,#14585,#8135,.T.);
#18348=EDGE_CURVE('',#14587,#14588,#8136,.T.);
#18349=EDGE_CURVE('',#14588,#14586,#8137,.T.);
#18350=EDGE_CURVE('',#14582,#14587,#8138,.T.);
#18351=EDGE_CURVE('',#14584,#14588,#8139,.T.);
#18352=EDGE_CURVE('',#14589,#14590,#8140,.T.);
#18353=EDGE_CURVE('',#14589,#14591,#8141,.T.);
#18354=EDGE_CURVE('',#14591,#14592,#8142,.T.);
#18355=EDGE_CURVE('',#14590,#14592,#8143,.T.);
#18356=EDGE_CURVE('',#14593,#14589,#8144,.T.);
#18357=EDGE_CURVE('',#14593,#14594,#8145,.T.);
#18358=EDGE_CURVE('',#14594,#14591,#8146,.T.);
#18359=EDGE_CURVE('',#14595,#14593,#8147,.T.);
#18360=EDGE_CURVE('',#14595,#14596,#8148,.T.);
#18361=EDGE_CURVE('',#14596,#14594,#8149,.T.);
#18362=EDGE_CURVE('',#14590,#14595,#8150,.T.);
#18363=EDGE_CURVE('',#14592,#14596,#8151,.T.);
#18364=EDGE_CURVE('',#14597,#14598,#8152,.T.);
#18365=EDGE_CURVE('',#14597,#14599,#8153,.T.);
#18366=EDGE_CURVE('',#14599,#14600,#8154,.T.);
#18367=EDGE_CURVE('',#14598,#14600,#8155,.T.);
#18368=EDGE_CURVE('',#14601,#14597,#8156,.T.);
#18369=EDGE_CURVE('',#14601,#14602,#8157,.T.);
#18370=EDGE_CURVE('',#14602,#14599,#8158,.T.);
#18371=EDGE_CURVE('',#14603,#14601,#8159,.T.);
#18372=EDGE_CURVE('',#14603,#14604,#8160,.T.);
#18373=EDGE_CURVE('',#14604,#14602,#8161,.T.);
#18374=EDGE_CURVE('',#14598,#14603,#8162,.T.);
#18375=EDGE_CURVE('',#14600,#14604,#8163,.T.);
#18376=EDGE_CURVE('',#14605,#14606,#8164,.T.);
#18377=EDGE_CURVE('',#14605,#14607,#8165,.T.);
#18378=EDGE_CURVE('',#14607,#14608,#8166,.T.);
#18379=EDGE_CURVE('',#14606,#14608,#8167,.T.);
#18380=EDGE_CURVE('',#14609,#14605,#8168,.T.);
#18381=EDGE_CURVE('',#14609,#14610,#8169,.T.);
#18382=EDGE_CURVE('',#14610,#14607,#8170,.T.);
#18383=EDGE_CURVE('',#14611,#14609,#8171,.T.);
#18384=EDGE_CURVE('',#14611,#14612,#8172,.T.);
#18385=EDGE_CURVE('',#14612,#14610,#8173,.T.);
#18386=EDGE_CURVE('',#14606,#14611,#8174,.T.);
#18387=EDGE_CURVE('',#14608,#14612,#8175,.T.);
#18388=EDGE_CURVE('',#14613,#14614,#8176,.T.);
#18389=EDGE_CURVE('',#14613,#14615,#8177,.T.);
#18390=EDGE_CURVE('',#14615,#14616,#8178,.T.);
#18391=EDGE_CURVE('',#14614,#14616,#8179,.T.);
#18392=EDGE_CURVE('',#14617,#14613,#8180,.T.);
#18393=EDGE_CURVE('',#14617,#14618,#8181,.T.);
#18394=EDGE_CURVE('',#14618,#14615,#8182,.T.);
#18395=EDGE_CURVE('',#14619,#14617,#8183,.T.);
#18396=EDGE_CURVE('',#14619,#14620,#8184,.T.);
#18397=EDGE_CURVE('',#14620,#14618,#8185,.T.);
#18398=EDGE_CURVE('',#14614,#14619,#8186,.T.);
#18399=EDGE_CURVE('',#14616,#14620,#8187,.T.);
#18400=EDGE_CURVE('',#14621,#14622,#8188,.T.);
#18401=EDGE_CURVE('',#14621,#14623,#8189,.T.);
#18402=EDGE_CURVE('',#14623,#14624,#8190,.T.);
#18403=EDGE_CURVE('',#14622,#14624,#8191,.T.);
#18404=EDGE_CURVE('',#14625,#14621,#8192,.T.);
#18405=EDGE_CURVE('',#14625,#14626,#8193,.T.);
#18406=EDGE_CURVE('',#14626,#14623,#8194,.T.);
#18407=EDGE_CURVE('',#14627,#14625,#8195,.T.);
#18408=EDGE_CURVE('',#14627,#14628,#8196,.T.);
#18409=EDGE_CURVE('',#14628,#14626,#8197,.T.);
#18410=EDGE_CURVE('',#14622,#14627,#8198,.T.);
#18411=EDGE_CURVE('',#14624,#14628,#8199,.T.);
#18412=EDGE_CURVE('',#14629,#14630,#8200,.T.);
#18413=EDGE_CURVE('',#14629,#14631,#8201,.T.);
#18414=EDGE_CURVE('',#14631,#14632,#8202,.T.);
#18415=EDGE_CURVE('',#14630,#14632,#8203,.T.);
#18416=EDGE_CURVE('',#14633,#14629,#8204,.T.);
#18417=EDGE_CURVE('',#14633,#14634,#8205,.T.);
#18418=EDGE_CURVE('',#14634,#14631,#8206,.T.);
#18419=EDGE_CURVE('',#14635,#14633,#8207,.T.);
#18420=EDGE_CURVE('',#14635,#14636,#8208,.T.);
#18421=EDGE_CURVE('',#14636,#14634,#8209,.T.);
#18422=EDGE_CURVE('',#14630,#14635,#8210,.T.);
#18423=EDGE_CURVE('',#14632,#14636,#8211,.T.);
#18424=EDGE_CURVE('',#14637,#14638,#8212,.T.);
#18425=EDGE_CURVE('',#14637,#14639,#8213,.T.);
#18426=EDGE_CURVE('',#14639,#14640,#8214,.T.);
#18427=EDGE_CURVE('',#14638,#14640,#8215,.T.);
#18428=EDGE_CURVE('',#14641,#14637,#8216,.T.);
#18429=EDGE_CURVE('',#14641,#14642,#8217,.T.);
#18430=EDGE_CURVE('',#14642,#14639,#8218,.T.);
#18431=EDGE_CURVE('',#14643,#14641,#8219,.T.);
#18432=EDGE_CURVE('',#14643,#14644,#8220,.T.);
#18433=EDGE_CURVE('',#14644,#14642,#8221,.T.);
#18434=EDGE_CURVE('',#14638,#14643,#8222,.T.);
#18435=EDGE_CURVE('',#14640,#14644,#8223,.T.);
#18436=EDGE_CURVE('',#14645,#14646,#8224,.T.);
#18437=EDGE_CURVE('',#14645,#14647,#8225,.T.);
#18438=EDGE_CURVE('',#14647,#14648,#8226,.T.);
#18439=EDGE_CURVE('',#14646,#14648,#8227,.T.);
#18440=EDGE_CURVE('',#14649,#14645,#8228,.T.);
#18441=EDGE_CURVE('',#14649,#14650,#8229,.T.);
#18442=EDGE_CURVE('',#14650,#14647,#8230,.T.);
#18443=EDGE_CURVE('',#14651,#14649,#8231,.T.);
#18444=EDGE_CURVE('',#14651,#14652,#8232,.T.);
#18445=EDGE_CURVE('',#14652,#14650,#8233,.T.);
#18446=EDGE_CURVE('',#14646,#14651,#8234,.T.);
#18447=EDGE_CURVE('',#14648,#14652,#8235,.T.);
#18448=EDGE_CURVE('',#14653,#14654,#8236,.T.);
#18449=EDGE_CURVE('',#14653,#14655,#8237,.T.);
#18450=EDGE_CURVE('',#14655,#14656,#8238,.T.);
#18451=EDGE_CURVE('',#14654,#14656,#8239,.T.);
#18452=EDGE_CURVE('',#14657,#14653,#8240,.T.);
#18453=EDGE_CURVE('',#14657,#14658,#8241,.T.);
#18454=EDGE_CURVE('',#14658,#14655,#8242,.T.);
#18455=EDGE_CURVE('',#14659,#14657,#8243,.T.);
#18456=EDGE_CURVE('',#14659,#14660,#8244,.T.);
#18457=EDGE_CURVE('',#14660,#14658,#8245,.T.);
#18458=EDGE_CURVE('',#14654,#14659,#8246,.T.);
#18459=EDGE_CURVE('',#14656,#14660,#8247,.T.);
#18460=EDGE_CURVE('',#14661,#14662,#8248,.T.);
#18461=EDGE_CURVE('',#14661,#14663,#8249,.T.);
#18462=EDGE_CURVE('',#14663,#14664,#8250,.T.);
#18463=EDGE_CURVE('',#14662,#14664,#8251,.T.);
#18464=EDGE_CURVE('',#14665,#14661,#8252,.T.);
#18465=EDGE_CURVE('',#14665,#14666,#8253,.T.);
#18466=EDGE_CURVE('',#14666,#14663,#8254,.T.);
#18467=EDGE_CURVE('',#14667,#14665,#8255,.T.);
#18468=EDGE_CURVE('',#14667,#14668,#8256,.T.);
#18469=EDGE_CURVE('',#14668,#14666,#8257,.T.);
#18470=EDGE_CURVE('',#14662,#14667,#8258,.T.);
#18471=EDGE_CURVE('',#14664,#14668,#8259,.T.);
#18472=EDGE_CURVE('',#14669,#14670,#8260,.T.);
#18473=EDGE_CURVE('',#14669,#14671,#8261,.T.);
#18474=EDGE_CURVE('',#14671,#14672,#8262,.T.);
#18475=EDGE_CURVE('',#14670,#14672,#8263,.T.);
#18476=EDGE_CURVE('',#14673,#14669,#8264,.T.);
#18477=EDGE_CURVE('',#14673,#14674,#8265,.T.);
#18478=EDGE_CURVE('',#14674,#14671,#8266,.T.);
#18479=EDGE_CURVE('',#14675,#14673,#8267,.T.);
#18480=EDGE_CURVE('',#14675,#14676,#8268,.T.);
#18481=EDGE_CURVE('',#14676,#14674,#8269,.T.);
#18482=EDGE_CURVE('',#14670,#14675,#8270,.T.);
#18483=EDGE_CURVE('',#14672,#14676,#8271,.T.);
#18484=EDGE_CURVE('',#14677,#14678,#8272,.T.);
#18485=EDGE_CURVE('',#14677,#14679,#8273,.T.);
#18486=EDGE_CURVE('',#14679,#14680,#8274,.T.);
#18487=EDGE_CURVE('',#14678,#14680,#8275,.T.);
#18488=EDGE_CURVE('',#14681,#14677,#8276,.T.);
#18489=EDGE_CURVE('',#14681,#14682,#8277,.T.);
#18490=EDGE_CURVE('',#14682,#14679,#8278,.T.);
#18491=EDGE_CURVE('',#14683,#14681,#8279,.T.);
#18492=EDGE_CURVE('',#14683,#14684,#8280,.T.);
#18493=EDGE_CURVE('',#14684,#14682,#8281,.T.);
#18494=EDGE_CURVE('',#14678,#14683,#8282,.T.);
#18495=EDGE_CURVE('',#14680,#14684,#8283,.T.);
#18496=EDGE_CURVE('',#14685,#14686,#8284,.T.);
#18497=EDGE_CURVE('',#14685,#14687,#8285,.T.);
#18498=EDGE_CURVE('',#14687,#14688,#8286,.T.);
#18499=EDGE_CURVE('',#14686,#14688,#8287,.T.);
#18500=EDGE_CURVE('',#14689,#14685,#8288,.T.);
#18501=EDGE_CURVE('',#14689,#14690,#8289,.T.);
#18502=EDGE_CURVE('',#14690,#14687,#8290,.T.);
#18503=EDGE_CURVE('',#14691,#14689,#8291,.T.);
#18504=EDGE_CURVE('',#14691,#14692,#8292,.T.);
#18505=EDGE_CURVE('',#14692,#14690,#8293,.T.);
#18506=EDGE_CURVE('',#14686,#14691,#8294,.T.);
#18507=EDGE_CURVE('',#14688,#14692,#8295,.T.);
#18508=EDGE_CURVE('',#14693,#14694,#8296,.T.);
#18509=EDGE_CURVE('',#14693,#14695,#8297,.T.);
#18510=EDGE_CURVE('',#14695,#14696,#8298,.T.);
#18511=EDGE_CURVE('',#14694,#14696,#8299,.T.);
#18512=EDGE_CURVE('',#14697,#14693,#8300,.T.);
#18513=EDGE_CURVE('',#14697,#14698,#8301,.T.);
#18514=EDGE_CURVE('',#14698,#14695,#8302,.T.);
#18515=EDGE_CURVE('',#14699,#14697,#8303,.T.);
#18516=EDGE_CURVE('',#14699,#14700,#8304,.T.);
#18517=EDGE_CURVE('',#14700,#14698,#8305,.T.);
#18518=EDGE_CURVE('',#14694,#14699,#8306,.T.);
#18519=EDGE_CURVE('',#14696,#14700,#8307,.T.);
#18520=EDGE_CURVE('',#14701,#14702,#8308,.T.);
#18521=EDGE_CURVE('',#14701,#14703,#8309,.T.);
#18522=EDGE_CURVE('',#14703,#14704,#8310,.T.);
#18523=EDGE_CURVE('',#14702,#14704,#8311,.T.);
#18524=EDGE_CURVE('',#14705,#14701,#8312,.T.);
#18525=EDGE_CURVE('',#14705,#14706,#8313,.T.);
#18526=EDGE_CURVE('',#14706,#14703,#8314,.T.);
#18527=EDGE_CURVE('',#14707,#14705,#8315,.T.);
#18528=EDGE_CURVE('',#14707,#14708,#8316,.T.);
#18529=EDGE_CURVE('',#14708,#14706,#8317,.T.);
#18530=EDGE_CURVE('',#14702,#14707,#8318,.T.);
#18531=EDGE_CURVE('',#14704,#14708,#8319,.T.);
#18532=EDGE_CURVE('',#14709,#14710,#8320,.T.);
#18533=EDGE_CURVE('',#14709,#14711,#8321,.T.);
#18534=EDGE_CURVE('',#14711,#14712,#8322,.T.);
#18535=EDGE_CURVE('',#14710,#14712,#8323,.T.);
#18536=EDGE_CURVE('',#14713,#14709,#8324,.T.);
#18537=EDGE_CURVE('',#14713,#14714,#8325,.T.);
#18538=EDGE_CURVE('',#14714,#14711,#8326,.T.);
#18539=EDGE_CURVE('',#14715,#14713,#8327,.T.);
#18540=EDGE_CURVE('',#14715,#14716,#8328,.T.);
#18541=EDGE_CURVE('',#14716,#14714,#8329,.T.);
#18542=EDGE_CURVE('',#14710,#14715,#8330,.T.);
#18543=EDGE_CURVE('',#14712,#14716,#8331,.T.);
#18544=EDGE_CURVE('',#14717,#14718,#8332,.T.);
#18545=EDGE_CURVE('',#14717,#14719,#8333,.T.);
#18546=EDGE_CURVE('',#14719,#14720,#8334,.T.);
#18547=EDGE_CURVE('',#14718,#14720,#8335,.T.);
#18548=EDGE_CURVE('',#14721,#14717,#8336,.T.);
#18549=EDGE_CURVE('',#14721,#14722,#8337,.T.);
#18550=EDGE_CURVE('',#14722,#14719,#8338,.T.);
#18551=EDGE_CURVE('',#14723,#14721,#8339,.T.);
#18552=EDGE_CURVE('',#14723,#14724,#8340,.T.);
#18553=EDGE_CURVE('',#14724,#14722,#8341,.T.);
#18554=EDGE_CURVE('',#14718,#14723,#8342,.T.);
#18555=EDGE_CURVE('',#14720,#14724,#8343,.T.);
#18556=EDGE_CURVE('',#14725,#14726,#8344,.T.);
#18557=EDGE_CURVE('',#14725,#14727,#8345,.T.);
#18558=EDGE_CURVE('',#14727,#14728,#8346,.T.);
#18559=EDGE_CURVE('',#14726,#14728,#8347,.T.);
#18560=EDGE_CURVE('',#14729,#14725,#8348,.T.);
#18561=EDGE_CURVE('',#14729,#14730,#8349,.T.);
#18562=EDGE_CURVE('',#14730,#14727,#8350,.T.);
#18563=EDGE_CURVE('',#14731,#14729,#8351,.T.);
#18564=EDGE_CURVE('',#14731,#14732,#8352,.T.);
#18565=EDGE_CURVE('',#14732,#14730,#8353,.T.);
#18566=EDGE_CURVE('',#14726,#14731,#8354,.T.);
#18567=EDGE_CURVE('',#14728,#14732,#8355,.T.);
#18568=EDGE_CURVE('',#14733,#14734,#8356,.T.);
#18569=EDGE_CURVE('',#14733,#14735,#8357,.T.);
#18570=EDGE_CURVE('',#14735,#14736,#8358,.T.);
#18571=EDGE_CURVE('',#14734,#14736,#8359,.T.);
#18572=EDGE_CURVE('',#14737,#14733,#8360,.T.);
#18573=EDGE_CURVE('',#14737,#14738,#8361,.T.);
#18574=EDGE_CURVE('',#14738,#14735,#8362,.T.);
#18575=EDGE_CURVE('',#14739,#14737,#8363,.T.);
#18576=EDGE_CURVE('',#14739,#14740,#8364,.T.);
#18577=EDGE_CURVE('',#14740,#14738,#8365,.T.);
#18578=EDGE_CURVE('',#14734,#14739,#8366,.T.);
#18579=EDGE_CURVE('',#14736,#14740,#8367,.T.);
#18580=EDGE_CURVE('',#14741,#14742,#8368,.T.);
#18581=EDGE_CURVE('',#14741,#14743,#8369,.T.);
#18582=EDGE_CURVE('',#14743,#14744,#8370,.T.);
#18583=EDGE_CURVE('',#14742,#14744,#8371,.T.);
#18584=EDGE_CURVE('',#14745,#14741,#8372,.T.);
#18585=EDGE_CURVE('',#14745,#14746,#8373,.T.);
#18586=EDGE_CURVE('',#14746,#14743,#8374,.T.);
#18587=EDGE_CURVE('',#14747,#14745,#8375,.T.);
#18588=EDGE_CURVE('',#14747,#14748,#8376,.T.);
#18589=EDGE_CURVE('',#14748,#14746,#8377,.T.);
#18590=EDGE_CURVE('',#14742,#14747,#8378,.T.);
#18591=EDGE_CURVE('',#14744,#14748,#8379,.T.);
#18592=EDGE_CURVE('',#14749,#14750,#8380,.T.);
#18593=EDGE_CURVE('',#14749,#14751,#8381,.T.);
#18594=EDGE_CURVE('',#14751,#14752,#8382,.T.);
#18595=EDGE_CURVE('',#14750,#14752,#8383,.T.);
#18596=EDGE_CURVE('',#14753,#14749,#8384,.T.);
#18597=EDGE_CURVE('',#14753,#14754,#8385,.T.);
#18598=EDGE_CURVE('',#14754,#14751,#8386,.T.);
#18599=EDGE_CURVE('',#14755,#14753,#8387,.T.);
#18600=EDGE_CURVE('',#14755,#14756,#8388,.T.);
#18601=EDGE_CURVE('',#14756,#14754,#8389,.T.);
#18602=EDGE_CURVE('',#14750,#14755,#8390,.T.);
#18603=EDGE_CURVE('',#14752,#14756,#8391,.T.);
#18604=EDGE_CURVE('',#14757,#14758,#8392,.T.);
#18605=EDGE_CURVE('',#14757,#14759,#8393,.T.);
#18606=EDGE_CURVE('',#14759,#14760,#8394,.T.);
#18607=EDGE_CURVE('',#14758,#14760,#8395,.T.);
#18608=EDGE_CURVE('',#14761,#14757,#8396,.T.);
#18609=EDGE_CURVE('',#14761,#14762,#8397,.T.);
#18610=EDGE_CURVE('',#14762,#14759,#8398,.T.);
#18611=EDGE_CURVE('',#14763,#14761,#8399,.T.);
#18612=EDGE_CURVE('',#14763,#14764,#8400,.T.);
#18613=EDGE_CURVE('',#14764,#14762,#8401,.T.);
#18614=EDGE_CURVE('',#14758,#14763,#8402,.T.);
#18615=EDGE_CURVE('',#14760,#14764,#8403,.T.);
#18616=EDGE_CURVE('',#14765,#14766,#8404,.T.);
#18617=EDGE_CURVE('',#14765,#14767,#8405,.T.);
#18618=EDGE_CURVE('',#14767,#14768,#8406,.T.);
#18619=EDGE_CURVE('',#14766,#14768,#8407,.T.);
#18620=EDGE_CURVE('',#14769,#14765,#8408,.T.);
#18621=EDGE_CURVE('',#14769,#14770,#8409,.T.);
#18622=EDGE_CURVE('',#14770,#14767,#8410,.T.);
#18623=EDGE_CURVE('',#14771,#14769,#8411,.T.);
#18624=EDGE_CURVE('',#14771,#14772,#8412,.T.);
#18625=EDGE_CURVE('',#14772,#14770,#8413,.T.);
#18626=EDGE_CURVE('',#14766,#14771,#8414,.T.);
#18627=EDGE_CURVE('',#14768,#14772,#8415,.T.);
#18628=EDGE_CURVE('',#14773,#14774,#8416,.T.);
#18629=EDGE_CURVE('',#14773,#14775,#8417,.T.);
#18630=EDGE_CURVE('',#14775,#14776,#8418,.T.);
#18631=EDGE_CURVE('',#14774,#14776,#8419,.T.);
#18632=EDGE_CURVE('',#14777,#14773,#8420,.T.);
#18633=EDGE_CURVE('',#14777,#14778,#8421,.T.);
#18634=EDGE_CURVE('',#14778,#14775,#8422,.T.);
#18635=EDGE_CURVE('',#14779,#14777,#8423,.T.);
#18636=EDGE_CURVE('',#14779,#14780,#8424,.T.);
#18637=EDGE_CURVE('',#14780,#14778,#8425,.T.);
#18638=EDGE_CURVE('',#14774,#14779,#8426,.T.);
#18639=EDGE_CURVE('',#14776,#14780,#8427,.T.);
#18640=EDGE_CURVE('',#14781,#14782,#8428,.T.);
#18641=EDGE_CURVE('',#14781,#14783,#8429,.T.);
#18642=EDGE_CURVE('',#14783,#14784,#8430,.T.);
#18643=EDGE_CURVE('',#14782,#14784,#8431,.T.);
#18644=EDGE_CURVE('',#14785,#14781,#8432,.T.);
#18645=EDGE_CURVE('',#14785,#14786,#8433,.T.);
#18646=EDGE_CURVE('',#14786,#14783,#8434,.T.);
#18647=EDGE_CURVE('',#14787,#14785,#8435,.T.);
#18648=EDGE_CURVE('',#14787,#14788,#8436,.T.);
#18649=EDGE_CURVE('',#14788,#14786,#8437,.T.);
#18650=EDGE_CURVE('',#14782,#14787,#8438,.T.);
#18651=EDGE_CURVE('',#14784,#14788,#8439,.T.);
#18652=EDGE_CURVE('',#14789,#14790,#8440,.T.);
#18653=EDGE_CURVE('',#14789,#14791,#8441,.T.);
#18654=EDGE_CURVE('',#14791,#14792,#8442,.T.);
#18655=EDGE_CURVE('',#14790,#14792,#8443,.T.);
#18656=EDGE_CURVE('',#14793,#14789,#8444,.T.);
#18657=EDGE_CURVE('',#14793,#14794,#8445,.T.);
#18658=EDGE_CURVE('',#14794,#14791,#8446,.T.);
#18659=EDGE_CURVE('',#14795,#14793,#8447,.T.);
#18660=EDGE_CURVE('',#14795,#14796,#8448,.T.);
#18661=EDGE_CURVE('',#14796,#14794,#8449,.T.);
#18662=EDGE_CURVE('',#14790,#14795,#8450,.T.);
#18663=EDGE_CURVE('',#14792,#14796,#8451,.T.);
#18664=EDGE_CURVE('',#14797,#14798,#8452,.T.);
#18665=EDGE_CURVE('',#14797,#14799,#8453,.T.);
#18666=EDGE_CURVE('',#14799,#14800,#8454,.T.);
#18667=EDGE_CURVE('',#14798,#14800,#8455,.T.);
#18668=EDGE_CURVE('',#14801,#14797,#8456,.T.);
#18669=EDGE_CURVE('',#14801,#14802,#8457,.T.);
#18670=EDGE_CURVE('',#14802,#14799,#8458,.T.);
#18671=EDGE_CURVE('',#14803,#14801,#8459,.T.);
#18672=EDGE_CURVE('',#14803,#14804,#8460,.T.);
#18673=EDGE_CURVE('',#14804,#14802,#8461,.T.);
#18674=EDGE_CURVE('',#14798,#14803,#8462,.T.);
#18675=EDGE_CURVE('',#14800,#14804,#8463,.T.);
#18676=EDGE_CURVE('',#14805,#14806,#8464,.T.);
#18677=EDGE_CURVE('',#14805,#14807,#8465,.T.);
#18678=EDGE_CURVE('',#14807,#14808,#8466,.T.);
#18679=EDGE_CURVE('',#14806,#14808,#8467,.T.);
#18680=EDGE_CURVE('',#14809,#14805,#8468,.T.);
#18681=EDGE_CURVE('',#14809,#14810,#8469,.T.);
#18682=EDGE_CURVE('',#14810,#14807,#8470,.T.);
#18683=EDGE_CURVE('',#14811,#14809,#8471,.T.);
#18684=EDGE_CURVE('',#14811,#14812,#8472,.T.);
#18685=EDGE_CURVE('',#14812,#14810,#8473,.T.);
#18686=EDGE_CURVE('',#14806,#14811,#8474,.T.);
#18687=EDGE_CURVE('',#14808,#14812,#8475,.T.);
#18688=EDGE_CURVE('',#14813,#14814,#8476,.T.);
#18689=EDGE_CURVE('',#14813,#14815,#8477,.T.);
#18690=EDGE_CURVE('',#14815,#14816,#8478,.T.);
#18691=EDGE_CURVE('',#14814,#14816,#8479,.T.);
#18692=EDGE_CURVE('',#14817,#14813,#8480,.T.);
#18693=EDGE_CURVE('',#14817,#14818,#8481,.T.);
#18694=EDGE_CURVE('',#14818,#14815,#8482,.T.);
#18695=EDGE_CURVE('',#14819,#14817,#8483,.T.);
#18696=EDGE_CURVE('',#14819,#14820,#8484,.T.);
#18697=EDGE_CURVE('',#14820,#14818,#8485,.T.);
#18698=EDGE_CURVE('',#14814,#14819,#8486,.T.);
#18699=EDGE_CURVE('',#14816,#14820,#8487,.T.);
#18700=EDGE_CURVE('',#14821,#14822,#8488,.T.);
#18701=EDGE_CURVE('',#14821,#14823,#8489,.T.);
#18702=EDGE_CURVE('',#14823,#14824,#8490,.T.);
#18703=EDGE_CURVE('',#14822,#14824,#8491,.T.);
#18704=EDGE_CURVE('',#14825,#14821,#8492,.T.);
#18705=EDGE_CURVE('',#14825,#14826,#8493,.T.);
#18706=EDGE_CURVE('',#14826,#14823,#8494,.T.);
#18707=EDGE_CURVE('',#14827,#14825,#8495,.T.);
#18708=EDGE_CURVE('',#14827,#14828,#8496,.T.);
#18709=EDGE_CURVE('',#14828,#14826,#8497,.T.);
#18710=EDGE_CURVE('',#14822,#14827,#8498,.T.);
#18711=EDGE_CURVE('',#14824,#14828,#8499,.T.);
#18712=EDGE_CURVE('',#14829,#14830,#8500,.T.);
#18713=EDGE_CURVE('',#14829,#14831,#8501,.T.);
#18714=EDGE_CURVE('',#14831,#14832,#8502,.T.);
#18715=EDGE_CURVE('',#14830,#14832,#8503,.T.);
#18716=EDGE_CURVE('',#14833,#14829,#8504,.T.);
#18717=EDGE_CURVE('',#14833,#14834,#8505,.T.);
#18718=EDGE_CURVE('',#14834,#14831,#8506,.T.);
#18719=EDGE_CURVE('',#14835,#14833,#8507,.T.);
#18720=EDGE_CURVE('',#14835,#14836,#8508,.T.);
#18721=EDGE_CURVE('',#14836,#14834,#8509,.T.);
#18722=EDGE_CURVE('',#14830,#14835,#8510,.T.);
#18723=EDGE_CURVE('',#14832,#14836,#8511,.T.);
#18724=EDGE_CURVE('',#14837,#14838,#8512,.T.);
#18725=EDGE_CURVE('',#14837,#14839,#8513,.T.);
#18726=EDGE_CURVE('',#14839,#14840,#8514,.T.);
#18727=EDGE_CURVE('',#14838,#14840,#8515,.T.);
#18728=EDGE_CURVE('',#14841,#14837,#8516,.T.);
#18729=EDGE_CURVE('',#14841,#14842,#8517,.T.);
#18730=EDGE_CURVE('',#14842,#14839,#8518,.T.);
#18731=EDGE_CURVE('',#14843,#14841,#8519,.T.);
#18732=EDGE_CURVE('',#14843,#14844,#8520,.T.);
#18733=EDGE_CURVE('',#14844,#14842,#8521,.T.);
#18734=EDGE_CURVE('',#14838,#14843,#8522,.T.);
#18735=EDGE_CURVE('',#14840,#14844,#8523,.T.);
#18736=EDGE_CURVE('',#14845,#14846,#8524,.T.);
#18737=EDGE_CURVE('',#14845,#14847,#8525,.T.);
#18738=EDGE_CURVE('',#14847,#14848,#8526,.T.);
#18739=EDGE_CURVE('',#14846,#14848,#8527,.T.);
#18740=EDGE_CURVE('',#14849,#14845,#8528,.T.);
#18741=EDGE_CURVE('',#14849,#14850,#8529,.T.);
#18742=EDGE_CURVE('',#14850,#14847,#8530,.T.);
#18743=EDGE_CURVE('',#14851,#14849,#8531,.T.);
#18744=EDGE_CURVE('',#14851,#14852,#8532,.T.);
#18745=EDGE_CURVE('',#14852,#14850,#8533,.T.);
#18746=EDGE_CURVE('',#14846,#14851,#8534,.T.);
#18747=EDGE_CURVE('',#14848,#14852,#8535,.T.);
#18748=EDGE_CURVE('',#14853,#14854,#8536,.T.);
#18749=EDGE_CURVE('',#14853,#14855,#8537,.T.);
#18750=EDGE_CURVE('',#14855,#14856,#8538,.T.);
#18751=EDGE_CURVE('',#14854,#14856,#8539,.T.);
#18752=EDGE_CURVE('',#14857,#14853,#8540,.T.);
#18753=EDGE_CURVE('',#14857,#14858,#8541,.T.);
#18754=EDGE_CURVE('',#14858,#14855,#8542,.T.);
#18755=EDGE_CURVE('',#14859,#14857,#8543,.T.);
#18756=EDGE_CURVE('',#14859,#14860,#8544,.T.);
#18757=EDGE_CURVE('',#14860,#14858,#8545,.T.);
#18758=EDGE_CURVE('',#14854,#14859,#8546,.T.);
#18759=EDGE_CURVE('',#14856,#14860,#8547,.T.);
#18760=EDGE_CURVE('',#14861,#14862,#8548,.T.);
#18761=EDGE_CURVE('',#14861,#14863,#8549,.T.);
#18762=EDGE_CURVE('',#14863,#14864,#8550,.T.);
#18763=EDGE_CURVE('',#14862,#14864,#8551,.T.);
#18764=EDGE_CURVE('',#14865,#14861,#8552,.T.);
#18765=EDGE_CURVE('',#14865,#14866,#8553,.T.);
#18766=EDGE_CURVE('',#14866,#14863,#8554,.T.);
#18767=EDGE_CURVE('',#14867,#14865,#8555,.T.);
#18768=EDGE_CURVE('',#14867,#14868,#8556,.T.);
#18769=EDGE_CURVE('',#14868,#14866,#8557,.T.);
#18770=EDGE_CURVE('',#14862,#14867,#8558,.T.);
#18771=EDGE_CURVE('',#14864,#14868,#8559,.T.);
#18772=EDGE_CURVE('',#14869,#14870,#8560,.T.);
#18773=EDGE_CURVE('',#14869,#14871,#8561,.T.);
#18774=EDGE_CURVE('',#14871,#14872,#8562,.T.);
#18775=EDGE_CURVE('',#14870,#14872,#8563,.T.);
#18776=EDGE_CURVE('',#14873,#14869,#8564,.T.);
#18777=EDGE_CURVE('',#14873,#14874,#8565,.T.);
#18778=EDGE_CURVE('',#14874,#14871,#8566,.T.);
#18779=EDGE_CURVE('',#14875,#14873,#8567,.T.);
#18780=EDGE_CURVE('',#14875,#14876,#8568,.T.);
#18781=EDGE_CURVE('',#14876,#14874,#8569,.T.);
#18782=EDGE_CURVE('',#14870,#14875,#8570,.T.);
#18783=EDGE_CURVE('',#14872,#14876,#8571,.T.);
#18784=EDGE_CURVE('',#14877,#14878,#8572,.T.);
#18785=EDGE_CURVE('',#14877,#14879,#8573,.T.);
#18786=EDGE_CURVE('',#14879,#14880,#8574,.T.);
#18787=EDGE_CURVE('',#14878,#14880,#8575,.T.);
#18788=EDGE_CURVE('',#14881,#14877,#8576,.T.);
#18789=EDGE_CURVE('',#14881,#14882,#8577,.T.);
#18790=EDGE_CURVE('',#14882,#14879,#8578,.T.);
#18791=EDGE_CURVE('',#14883,#14881,#8579,.T.);
#18792=EDGE_CURVE('',#14883,#14884,#8580,.T.);
#18793=EDGE_CURVE('',#14884,#14882,#8581,.T.);
#18794=EDGE_CURVE('',#14878,#14883,#8582,.T.);
#18795=EDGE_CURVE('',#14880,#14884,#8583,.T.);
#18796=EDGE_CURVE('',#14885,#14886,#8584,.T.);
#18797=EDGE_CURVE('',#14885,#14887,#8585,.T.);
#18798=EDGE_CURVE('',#14887,#14888,#8586,.T.);
#18799=EDGE_CURVE('',#14886,#14888,#8587,.T.);
#18800=EDGE_CURVE('',#14889,#14885,#8588,.T.);
#18801=EDGE_CURVE('',#14889,#14890,#8589,.T.);
#18802=EDGE_CURVE('',#14890,#14887,#8590,.T.);
#18803=EDGE_CURVE('',#14891,#14889,#8591,.T.);
#18804=EDGE_CURVE('',#14891,#14892,#8592,.T.);
#18805=EDGE_CURVE('',#14892,#14890,#8593,.T.);
#18806=EDGE_CURVE('',#14886,#14891,#8594,.T.);
#18807=EDGE_CURVE('',#14888,#14892,#8595,.T.);
#18808=EDGE_CURVE('',#14893,#14894,#8596,.T.);
#18809=EDGE_CURVE('',#14893,#14895,#8597,.T.);
#18810=EDGE_CURVE('',#14895,#14896,#8598,.T.);
#18811=EDGE_CURVE('',#14894,#14896,#8599,.T.);
#18812=EDGE_CURVE('',#14897,#14893,#8600,.T.);
#18813=EDGE_CURVE('',#14897,#14898,#8601,.T.);
#18814=EDGE_CURVE('',#14898,#14895,#8602,.T.);
#18815=EDGE_CURVE('',#14899,#14897,#8603,.T.);
#18816=EDGE_CURVE('',#14899,#14900,#8604,.T.);
#18817=EDGE_CURVE('',#14900,#14898,#8605,.T.);
#18818=EDGE_CURVE('',#14894,#14899,#8606,.T.);
#18819=EDGE_CURVE('',#14896,#14900,#8607,.T.);
#18820=EDGE_CURVE('',#14901,#14902,#8608,.T.);
#18821=EDGE_CURVE('',#14901,#14903,#8609,.T.);
#18822=EDGE_CURVE('',#14903,#14904,#8610,.T.);
#18823=EDGE_CURVE('',#14902,#14904,#8611,.T.);
#18824=EDGE_CURVE('',#14905,#14901,#8612,.T.);
#18825=EDGE_CURVE('',#14905,#14906,#8613,.T.);
#18826=EDGE_CURVE('',#14906,#14903,#8614,.T.);
#18827=EDGE_CURVE('',#14907,#14905,#8615,.T.);
#18828=EDGE_CURVE('',#14907,#14908,#8616,.T.);
#18829=EDGE_CURVE('',#14908,#14906,#8617,.T.);
#18830=EDGE_CURVE('',#14902,#14907,#8618,.T.);
#18831=EDGE_CURVE('',#14904,#14908,#8619,.T.);
#18832=EDGE_CURVE('',#14909,#14910,#8620,.T.);
#18833=EDGE_CURVE('',#14909,#14911,#8621,.T.);
#18834=EDGE_CURVE('',#14911,#14912,#8622,.T.);
#18835=EDGE_CURVE('',#14910,#14912,#8623,.T.);
#18836=EDGE_CURVE('',#14913,#14909,#8624,.T.);
#18837=EDGE_CURVE('',#14913,#14914,#8625,.T.);
#18838=EDGE_CURVE('',#14914,#14911,#8626,.T.);
#18839=EDGE_CURVE('',#14915,#14913,#8627,.T.);
#18840=EDGE_CURVE('',#14915,#14916,#8628,.T.);
#18841=EDGE_CURVE('',#14916,#14914,#8629,.T.);
#18842=EDGE_CURVE('',#14910,#14915,#8630,.T.);
#18843=EDGE_CURVE('',#14912,#14916,#8631,.T.);
#18844=EDGE_CURVE('',#14917,#14918,#8632,.T.);
#18845=EDGE_CURVE('',#14917,#14919,#8633,.T.);
#18846=EDGE_CURVE('',#14919,#14920,#8634,.T.);
#18847=EDGE_CURVE('',#14918,#14920,#8635,.T.);
#18848=EDGE_CURVE('',#14921,#14917,#8636,.T.);
#18849=EDGE_CURVE('',#14921,#14922,#8637,.T.);
#18850=EDGE_CURVE('',#14922,#14919,#8638,.T.);
#18851=EDGE_CURVE('',#14923,#14921,#8639,.T.);
#18852=EDGE_CURVE('',#14923,#14924,#8640,.T.);
#18853=EDGE_CURVE('',#14924,#14922,#8641,.T.);
#18854=EDGE_CURVE('',#14918,#14923,#8642,.T.);
#18855=EDGE_CURVE('',#14920,#14924,#8643,.T.);
#18856=EDGE_CURVE('',#14925,#14926,#8644,.T.);
#18857=EDGE_CURVE('',#14925,#14927,#8645,.T.);
#18858=EDGE_CURVE('',#14927,#14928,#8646,.T.);
#18859=EDGE_CURVE('',#14926,#14928,#8647,.T.);
#18860=EDGE_CURVE('',#14929,#14925,#8648,.T.);
#18861=EDGE_CURVE('',#14929,#14930,#8649,.T.);
#18862=EDGE_CURVE('',#14930,#14927,#8650,.T.);
#18863=EDGE_CURVE('',#14931,#14929,#8651,.T.);
#18864=EDGE_CURVE('',#14931,#14932,#8652,.T.);
#18865=EDGE_CURVE('',#14932,#14930,#8653,.T.);
#18866=EDGE_CURVE('',#14926,#14931,#8654,.T.);
#18867=EDGE_CURVE('',#14928,#14932,#8655,.T.);
#18868=EDGE_CURVE('',#14933,#14934,#8656,.T.);
#18869=EDGE_CURVE('',#14933,#14935,#8657,.T.);
#18870=EDGE_CURVE('',#14935,#14936,#8658,.T.);
#18871=EDGE_CURVE('',#14934,#14936,#8659,.T.);
#18872=EDGE_CURVE('',#14937,#14933,#8660,.T.);
#18873=EDGE_CURVE('',#14937,#14938,#8661,.T.);
#18874=EDGE_CURVE('',#14938,#14935,#8662,.T.);
#18875=EDGE_CURVE('',#14939,#14937,#8663,.T.);
#18876=EDGE_CURVE('',#14939,#14940,#8664,.T.);
#18877=EDGE_CURVE('',#14940,#14938,#8665,.T.);
#18878=EDGE_CURVE('',#14934,#14939,#8666,.T.);
#18879=EDGE_CURVE('',#14936,#14940,#8667,.T.);
#18880=EDGE_CURVE('',#14941,#14942,#8668,.T.);
#18881=EDGE_CURVE('',#14941,#14943,#8669,.T.);
#18882=EDGE_CURVE('',#14943,#14944,#8670,.T.);
#18883=EDGE_CURVE('',#14942,#14944,#8671,.T.);
#18884=EDGE_CURVE('',#14945,#14941,#8672,.T.);
#18885=EDGE_CURVE('',#14945,#14946,#8673,.T.);
#18886=EDGE_CURVE('',#14946,#14943,#8674,.T.);
#18887=EDGE_CURVE('',#14947,#14945,#8675,.T.);
#18888=EDGE_CURVE('',#14947,#14948,#8676,.T.);
#18889=EDGE_CURVE('',#14948,#14946,#8677,.T.);
#18890=EDGE_CURVE('',#14942,#14947,#8678,.T.);
#18891=EDGE_CURVE('',#14944,#14948,#8679,.T.);
#18892=EDGE_CURVE('',#14949,#14950,#8680,.T.);
#18893=EDGE_CURVE('',#14949,#14951,#8681,.T.);
#18894=EDGE_CURVE('',#14951,#14952,#8682,.T.);
#18895=EDGE_CURVE('',#14950,#14952,#8683,.T.);
#18896=EDGE_CURVE('',#14953,#14949,#8684,.T.);
#18897=EDGE_CURVE('',#14953,#14954,#8685,.T.);
#18898=EDGE_CURVE('',#14954,#14951,#8686,.T.);
#18899=EDGE_CURVE('',#14955,#14953,#8687,.T.);
#18900=EDGE_CURVE('',#14955,#14956,#8688,.T.);
#18901=EDGE_CURVE('',#14956,#14954,#8689,.T.);
#18902=EDGE_CURVE('',#14950,#14955,#8690,.T.);
#18903=EDGE_CURVE('',#14952,#14956,#8691,.T.);
#18904=EDGE_CURVE('',#14957,#14958,#8692,.T.);
#18905=EDGE_CURVE('',#14957,#14959,#8693,.T.);
#18906=EDGE_CURVE('',#14959,#14960,#8694,.T.);
#18907=EDGE_CURVE('',#14958,#14960,#8695,.T.);
#18908=EDGE_CURVE('',#14961,#14957,#8696,.T.);
#18909=EDGE_CURVE('',#14961,#14962,#8697,.T.);
#18910=EDGE_CURVE('',#14962,#14959,#8698,.T.);
#18911=EDGE_CURVE('',#14963,#14961,#8699,.T.);
#18912=EDGE_CURVE('',#14963,#14964,#8700,.T.);
#18913=EDGE_CURVE('',#14964,#14962,#8701,.T.);
#18914=EDGE_CURVE('',#14958,#14963,#8702,.T.);
#18915=EDGE_CURVE('',#14960,#14964,#8703,.T.);
#18916=EDGE_CURVE('',#14965,#14966,#8704,.T.);
#18917=EDGE_CURVE('',#14965,#14967,#8705,.T.);
#18918=EDGE_CURVE('',#14967,#14968,#8706,.T.);
#18919=EDGE_CURVE('',#14966,#14968,#8707,.T.);
#18920=EDGE_CURVE('',#14969,#14965,#8708,.T.);
#18921=EDGE_CURVE('',#14969,#14970,#8709,.T.);
#18922=EDGE_CURVE('',#14970,#14967,#8710,.T.);
#18923=EDGE_CURVE('',#14971,#14969,#8711,.T.);
#18924=EDGE_CURVE('',#14971,#14972,#8712,.T.);
#18925=EDGE_CURVE('',#14972,#14970,#8713,.T.);
#18926=EDGE_CURVE('',#14966,#14971,#8714,.T.);
#18927=EDGE_CURVE('',#14968,#14972,#8715,.T.);
#18928=EDGE_CURVE('',#14973,#14974,#8716,.T.);
#18929=EDGE_CURVE('',#14973,#14975,#8717,.T.);
#18930=EDGE_CURVE('',#14975,#14976,#8718,.T.);
#18931=EDGE_CURVE('',#14974,#14976,#8719,.T.);
#18932=EDGE_CURVE('',#14977,#14973,#8720,.T.);
#18933=EDGE_CURVE('',#14977,#14978,#8721,.T.);
#18934=EDGE_CURVE('',#14978,#14975,#8722,.T.);
#18935=EDGE_CURVE('',#14979,#14977,#8723,.T.);
#18936=EDGE_CURVE('',#14979,#14980,#8724,.T.);
#18937=EDGE_CURVE('',#14980,#14978,#8725,.T.);
#18938=EDGE_CURVE('',#14974,#14979,#8726,.T.);
#18939=EDGE_CURVE('',#14976,#14980,#8727,.T.);
#18940=EDGE_CURVE('',#14981,#14982,#8728,.T.);
#18941=EDGE_CURVE('',#14981,#14983,#8729,.T.);
#18942=EDGE_CURVE('',#14983,#14984,#8730,.T.);
#18943=EDGE_CURVE('',#14982,#14984,#8731,.T.);
#18944=EDGE_CURVE('',#14985,#14981,#8732,.T.);
#18945=EDGE_CURVE('',#14985,#14986,#8733,.T.);
#18946=EDGE_CURVE('',#14986,#14983,#8734,.T.);
#18947=EDGE_CURVE('',#14987,#14985,#8735,.T.);
#18948=EDGE_CURVE('',#14987,#14988,#8736,.T.);
#18949=EDGE_CURVE('',#14988,#14986,#8737,.T.);
#18950=EDGE_CURVE('',#14982,#14987,#8738,.T.);
#18951=EDGE_CURVE('',#14984,#14988,#8739,.T.);
#18952=EDGE_CURVE('',#14989,#14990,#8740,.T.);
#18953=EDGE_CURVE('',#14989,#14991,#8741,.T.);
#18954=EDGE_CURVE('',#14991,#14992,#8742,.T.);
#18955=EDGE_CURVE('',#14990,#14992,#8743,.T.);
#18956=EDGE_CURVE('',#14993,#14989,#8744,.T.);
#18957=EDGE_CURVE('',#14993,#14994,#8745,.T.);
#18958=EDGE_CURVE('',#14994,#14991,#8746,.T.);
#18959=EDGE_CURVE('',#14995,#14993,#8747,.T.);
#18960=EDGE_CURVE('',#14995,#14996,#8748,.T.);
#18961=EDGE_CURVE('',#14996,#14994,#8749,.T.);
#18962=EDGE_CURVE('',#14990,#14995,#8750,.T.);
#18963=EDGE_CURVE('',#14992,#14996,#8751,.T.);
#18964=EDGE_CURVE('',#14997,#14998,#8752,.T.);
#18965=EDGE_CURVE('',#14997,#14999,#8753,.T.);
#18966=EDGE_CURVE('',#14999,#15000,#8754,.T.);
#18967=EDGE_CURVE('',#14998,#15000,#8755,.T.);
#18968=EDGE_CURVE('',#15001,#14997,#8756,.T.);
#18969=EDGE_CURVE('',#15001,#15002,#8757,.T.);
#18970=EDGE_CURVE('',#15002,#14999,#8758,.T.);
#18971=EDGE_CURVE('',#15003,#15001,#8759,.T.);
#18972=EDGE_CURVE('',#15003,#15004,#8760,.T.);
#18973=EDGE_CURVE('',#15004,#15002,#8761,.T.);
#18974=EDGE_CURVE('',#14998,#15003,#8762,.T.);
#18975=EDGE_CURVE('',#15000,#15004,#8763,.T.);
#18976=EDGE_CURVE('',#15005,#15006,#8764,.T.);
#18977=EDGE_CURVE('',#15005,#15007,#8765,.T.);
#18978=EDGE_CURVE('',#15007,#15008,#8766,.T.);
#18979=EDGE_CURVE('',#15006,#15008,#8767,.T.);
#18980=EDGE_CURVE('',#15009,#15005,#8768,.T.);
#18981=EDGE_CURVE('',#15009,#15010,#8769,.T.);
#18982=EDGE_CURVE('',#15010,#15007,#8770,.T.);
#18983=EDGE_CURVE('',#15011,#15009,#8771,.T.);
#18984=EDGE_CURVE('',#15011,#15012,#8772,.T.);
#18985=EDGE_CURVE('',#15012,#15010,#8773,.T.);
#18986=EDGE_CURVE('',#15006,#15011,#8774,.T.);
#18987=EDGE_CURVE('',#15008,#15012,#8775,.T.);
#18988=EDGE_CURVE('',#15013,#15014,#8776,.T.);
#18989=EDGE_CURVE('',#15013,#15015,#8777,.T.);
#18990=EDGE_CURVE('',#15015,#15016,#8778,.T.);
#18991=EDGE_CURVE('',#15014,#15016,#8779,.T.);
#18992=EDGE_CURVE('',#15017,#15013,#8780,.T.);
#18993=EDGE_CURVE('',#15017,#15018,#8781,.T.);
#18994=EDGE_CURVE('',#15018,#15015,#8782,.T.);
#18995=EDGE_CURVE('',#15019,#15017,#8783,.T.);
#18996=EDGE_CURVE('',#15019,#15020,#8784,.T.);
#18997=EDGE_CURVE('',#15020,#15018,#8785,.T.);
#18998=EDGE_CURVE('',#15014,#15019,#8786,.T.);
#18999=EDGE_CURVE('',#15016,#15020,#8787,.T.);
#19000=EDGE_CURVE('',#15021,#15022,#8788,.T.);
#19001=EDGE_CURVE('',#15021,#15023,#8789,.T.);
#19002=EDGE_CURVE('',#15023,#15024,#8790,.T.);
#19003=EDGE_CURVE('',#15022,#15024,#8791,.T.);
#19004=EDGE_CURVE('',#15025,#15021,#8792,.T.);
#19005=EDGE_CURVE('',#15025,#15026,#8793,.T.);
#19006=EDGE_CURVE('',#15026,#15023,#8794,.T.);
#19007=EDGE_CURVE('',#15027,#15025,#8795,.T.);
#19008=EDGE_CURVE('',#15027,#15028,#8796,.T.);
#19009=EDGE_CURVE('',#15028,#15026,#8797,.T.);
#19010=EDGE_CURVE('',#15022,#15027,#8798,.T.);
#19011=EDGE_CURVE('',#15024,#15028,#8799,.T.);
#19012=EDGE_CURVE('',#15029,#15030,#8800,.T.);
#19013=EDGE_CURVE('',#15029,#15031,#8801,.T.);
#19014=EDGE_CURVE('',#15031,#15032,#8802,.T.);
#19015=EDGE_CURVE('',#15030,#15032,#8803,.T.);
#19016=EDGE_CURVE('',#15033,#15029,#8804,.T.);
#19017=EDGE_CURVE('',#15033,#15034,#8805,.T.);
#19018=EDGE_CURVE('',#15034,#15031,#8806,.T.);
#19019=EDGE_CURVE('',#15035,#15033,#8807,.T.);
#19020=EDGE_CURVE('',#15035,#15036,#8808,.T.);
#19021=EDGE_CURVE('',#15036,#15034,#8809,.T.);
#19022=EDGE_CURVE('',#15030,#15035,#8810,.T.);
#19023=EDGE_CURVE('',#15032,#15036,#8811,.T.);
#19024=EDGE_CURVE('',#15037,#15038,#8812,.T.);
#19025=EDGE_CURVE('',#15037,#15039,#8813,.T.);
#19026=EDGE_CURVE('',#15039,#15040,#8814,.T.);
#19027=EDGE_CURVE('',#15038,#15040,#8815,.T.);
#19028=EDGE_CURVE('',#15041,#15037,#8816,.T.);
#19029=EDGE_CURVE('',#15041,#15042,#8817,.T.);
#19030=EDGE_CURVE('',#15042,#15039,#8818,.T.);
#19031=EDGE_CURVE('',#15043,#15041,#8819,.T.);
#19032=EDGE_CURVE('',#15043,#15044,#8820,.T.);
#19033=EDGE_CURVE('',#15044,#15042,#8821,.T.);
#19034=EDGE_CURVE('',#15038,#15043,#8822,.T.);
#19035=EDGE_CURVE('',#15040,#15044,#8823,.T.);
#19036=EDGE_CURVE('',#15045,#15046,#8824,.T.);
#19037=EDGE_CURVE('',#15045,#15047,#8825,.T.);
#19038=EDGE_CURVE('',#15047,#15048,#8826,.T.);
#19039=EDGE_CURVE('',#15046,#15048,#8827,.T.);
#19040=EDGE_CURVE('',#15049,#15045,#8828,.T.);
#19041=EDGE_CURVE('',#15049,#15050,#8829,.T.);
#19042=EDGE_CURVE('',#15050,#15047,#8830,.T.);
#19043=EDGE_CURVE('',#15051,#15049,#8831,.T.);
#19044=EDGE_CURVE('',#15051,#15052,#8832,.T.);
#19045=EDGE_CURVE('',#15052,#15050,#8833,.T.);
#19046=EDGE_CURVE('',#15046,#15051,#8834,.T.);
#19047=EDGE_CURVE('',#15048,#15052,#8835,.T.);
#19048=EDGE_CURVE('',#15053,#15054,#8836,.T.);
#19049=EDGE_CURVE('',#15053,#15055,#8837,.T.);
#19050=EDGE_CURVE('',#15055,#15056,#8838,.T.);
#19051=EDGE_CURVE('',#15054,#15056,#8839,.T.);
#19052=EDGE_CURVE('',#15057,#15053,#8840,.T.);
#19053=EDGE_CURVE('',#15057,#15058,#8841,.T.);
#19054=EDGE_CURVE('',#15058,#15055,#8842,.T.);
#19055=EDGE_CURVE('',#15059,#15057,#8843,.T.);
#19056=EDGE_CURVE('',#15059,#15060,#8844,.T.);
#19057=EDGE_CURVE('',#15060,#15058,#8845,.T.);
#19058=EDGE_CURVE('',#15054,#15059,#8846,.T.);
#19059=EDGE_CURVE('',#15056,#15060,#8847,.T.);
#19060=EDGE_CURVE('',#15061,#15062,#8848,.T.);
#19061=EDGE_CURVE('',#15061,#15063,#8849,.T.);
#19062=EDGE_CURVE('',#15063,#15064,#8850,.T.);
#19063=EDGE_CURVE('',#15062,#15064,#8851,.T.);
#19064=EDGE_CURVE('',#15065,#15061,#8852,.T.);
#19065=EDGE_CURVE('',#15065,#15066,#8853,.T.);
#19066=EDGE_CURVE('',#15066,#15063,#8854,.T.);
#19067=EDGE_CURVE('',#15067,#15065,#8855,.T.);
#19068=EDGE_CURVE('',#15067,#15068,#8856,.T.);
#19069=EDGE_CURVE('',#15068,#15066,#8857,.T.);
#19070=EDGE_CURVE('',#15062,#15067,#8858,.T.);
#19071=EDGE_CURVE('',#15064,#15068,#8859,.T.);
#19072=EDGE_CURVE('',#15069,#15070,#8860,.T.);
#19073=EDGE_CURVE('',#15069,#15071,#8861,.T.);
#19074=EDGE_CURVE('',#15071,#15072,#8862,.T.);
#19075=EDGE_CURVE('',#15070,#15072,#8863,.T.);
#19076=EDGE_CURVE('',#15073,#15069,#8864,.T.);
#19077=EDGE_CURVE('',#15073,#15074,#8865,.T.);
#19078=EDGE_CURVE('',#15074,#15071,#8866,.T.);
#19079=EDGE_CURVE('',#15075,#15073,#8867,.T.);
#19080=EDGE_CURVE('',#15075,#15076,#8868,.T.);
#19081=EDGE_CURVE('',#15076,#15074,#8869,.T.);
#19082=EDGE_CURVE('',#15070,#15075,#8870,.T.);
#19083=EDGE_CURVE('',#15072,#15076,#8871,.T.);
#19084=EDGE_CURVE('',#15077,#15078,#8872,.T.);
#19085=EDGE_CURVE('',#15077,#15079,#8873,.T.);
#19086=EDGE_CURVE('',#15079,#15080,#8874,.T.);
#19087=EDGE_CURVE('',#15078,#15080,#8875,.T.);
#19088=EDGE_CURVE('',#15081,#15077,#8876,.T.);
#19089=EDGE_CURVE('',#15081,#15082,#8877,.T.);
#19090=EDGE_CURVE('',#15082,#15079,#8878,.T.);
#19091=EDGE_CURVE('',#15083,#15081,#8879,.T.);
#19092=EDGE_CURVE('',#15083,#15084,#8880,.T.);
#19093=EDGE_CURVE('',#15084,#15082,#8881,.T.);
#19094=EDGE_CURVE('',#15078,#15083,#8882,.T.);
#19095=EDGE_CURVE('',#15080,#15084,#8883,.T.);
#19096=EDGE_CURVE('',#15085,#15086,#8884,.T.);
#19097=EDGE_CURVE('',#15085,#15087,#8885,.T.);
#19098=EDGE_CURVE('',#15087,#15088,#8886,.T.);
#19099=EDGE_CURVE('',#15086,#15088,#8887,.T.);
#19100=EDGE_CURVE('',#15089,#15085,#8888,.T.);
#19101=EDGE_CURVE('',#15089,#15090,#8889,.T.);
#19102=EDGE_CURVE('',#15090,#15087,#8890,.T.);
#19103=EDGE_CURVE('',#15091,#15089,#8891,.T.);
#19104=EDGE_CURVE('',#15091,#15092,#8892,.T.);
#19105=EDGE_CURVE('',#15092,#15090,#8893,.T.);
#19106=EDGE_CURVE('',#15086,#15091,#8894,.T.);
#19107=EDGE_CURVE('',#15088,#15092,#8895,.T.);
#19108=EDGE_CURVE('',#15093,#15094,#8896,.T.);
#19109=EDGE_CURVE('',#15093,#15095,#8897,.T.);
#19110=EDGE_CURVE('',#15095,#15096,#8898,.T.);
#19111=EDGE_CURVE('',#15094,#15096,#8899,.T.);
#19112=EDGE_CURVE('',#15097,#15093,#8900,.T.);
#19113=EDGE_CURVE('',#15097,#15098,#8901,.T.);
#19114=EDGE_CURVE('',#15098,#15095,#8902,.T.);
#19115=EDGE_CURVE('',#15099,#15097,#8903,.T.);
#19116=EDGE_CURVE('',#15099,#15100,#8904,.T.);
#19117=EDGE_CURVE('',#15100,#15098,#8905,.T.);
#19118=EDGE_CURVE('',#15094,#15099,#8906,.T.);
#19119=EDGE_CURVE('',#15096,#15100,#8907,.T.);
#19120=EDGE_CURVE('',#15101,#15102,#8908,.T.);
#19121=EDGE_CURVE('',#15101,#15103,#8909,.T.);
#19122=EDGE_CURVE('',#15103,#15104,#8910,.T.);
#19123=EDGE_CURVE('',#15102,#15104,#8911,.T.);
#19124=EDGE_CURVE('',#15105,#15101,#8912,.T.);
#19125=EDGE_CURVE('',#15105,#15106,#8913,.T.);
#19126=EDGE_CURVE('',#15106,#15103,#8914,.T.);
#19127=EDGE_CURVE('',#15107,#15105,#8915,.T.);
#19128=EDGE_CURVE('',#15107,#15108,#8916,.T.);
#19129=EDGE_CURVE('',#15108,#15106,#8917,.T.);
#19130=EDGE_CURVE('',#15102,#15107,#8918,.T.);
#19131=EDGE_CURVE('',#15104,#15108,#8919,.T.);
#19132=EDGE_CURVE('',#15109,#15110,#8920,.T.);
#19133=EDGE_CURVE('',#15109,#15111,#8921,.T.);
#19134=EDGE_CURVE('',#15111,#15112,#8922,.T.);
#19135=EDGE_CURVE('',#15110,#15112,#8923,.T.);
#19136=EDGE_CURVE('',#15113,#15109,#8924,.T.);
#19137=EDGE_CURVE('',#15113,#15114,#8925,.T.);
#19138=EDGE_CURVE('',#15114,#15111,#8926,.T.);
#19139=EDGE_CURVE('',#15115,#15113,#8927,.T.);
#19140=EDGE_CURVE('',#15115,#15116,#8928,.T.);
#19141=EDGE_CURVE('',#15116,#15114,#8929,.T.);
#19142=EDGE_CURVE('',#15110,#15115,#8930,.T.);
#19143=EDGE_CURVE('',#15112,#15116,#8931,.T.);
#19144=EDGE_CURVE('',#15117,#15118,#8932,.T.);
#19145=EDGE_CURVE('',#15117,#15119,#8933,.T.);
#19146=EDGE_CURVE('',#15119,#15120,#8934,.T.);
#19147=EDGE_CURVE('',#15118,#15120,#8935,.T.);
#19148=EDGE_CURVE('',#15121,#15117,#8936,.T.);
#19149=EDGE_CURVE('',#15121,#15122,#8937,.T.);
#19150=EDGE_CURVE('',#15122,#15119,#8938,.T.);
#19151=EDGE_CURVE('',#15123,#15121,#8939,.T.);
#19152=EDGE_CURVE('',#15123,#15124,#8940,.T.);
#19153=EDGE_CURVE('',#15124,#15122,#8941,.T.);
#19154=EDGE_CURVE('',#15118,#15123,#8942,.T.);
#19155=EDGE_CURVE('',#15120,#15124,#8943,.T.);
#19156=EDGE_CURVE('',#15125,#15126,#8944,.T.);
#19157=EDGE_CURVE('',#15125,#15127,#8945,.T.);
#19158=EDGE_CURVE('',#15127,#15128,#8946,.T.);
#19159=EDGE_CURVE('',#15126,#15128,#8947,.T.);
#19160=EDGE_CURVE('',#15129,#15125,#8948,.T.);
#19161=EDGE_CURVE('',#15129,#15130,#8949,.T.);
#19162=EDGE_CURVE('',#15130,#15127,#8950,.T.);
#19163=EDGE_CURVE('',#15131,#15129,#8951,.T.);
#19164=EDGE_CURVE('',#15131,#15132,#8952,.T.);
#19165=EDGE_CURVE('',#15132,#15130,#8953,.T.);
#19166=EDGE_CURVE('',#15126,#15131,#8954,.T.);
#19167=EDGE_CURVE('',#15128,#15132,#8955,.T.);
#19168=EDGE_CURVE('',#15133,#15134,#8956,.T.);
#19169=EDGE_CURVE('',#15133,#15135,#8957,.T.);
#19170=EDGE_CURVE('',#15135,#15136,#8958,.T.);
#19171=EDGE_CURVE('',#15134,#15136,#8959,.T.);
#19172=EDGE_CURVE('',#15137,#15133,#8960,.T.);
#19173=EDGE_CURVE('',#15137,#15138,#8961,.T.);
#19174=EDGE_CURVE('',#15138,#15135,#8962,.T.);
#19175=EDGE_CURVE('',#15139,#15137,#8963,.T.);
#19176=EDGE_CURVE('',#15139,#15140,#8964,.T.);
#19177=EDGE_CURVE('',#15140,#15138,#8965,.T.);
#19178=EDGE_CURVE('',#15134,#15139,#8966,.T.);
#19179=EDGE_CURVE('',#15136,#15140,#8967,.T.);
#19180=EDGE_CURVE('',#15141,#15142,#8968,.T.);
#19181=EDGE_CURVE('',#15141,#15143,#8969,.T.);
#19182=EDGE_CURVE('',#15143,#15144,#8970,.T.);
#19183=EDGE_CURVE('',#15142,#15144,#8971,.T.);
#19184=EDGE_CURVE('',#15145,#15141,#8972,.T.);
#19185=EDGE_CURVE('',#15145,#15146,#8973,.T.);
#19186=EDGE_CURVE('',#15146,#15143,#8974,.T.);
#19187=EDGE_CURVE('',#15147,#15145,#8975,.T.);
#19188=EDGE_CURVE('',#15147,#15148,#8976,.T.);
#19189=EDGE_CURVE('',#15148,#15146,#8977,.T.);
#19190=EDGE_CURVE('',#15142,#15147,#8978,.T.);
#19191=EDGE_CURVE('',#15144,#15148,#8979,.T.);
#19192=EDGE_CURVE('',#15149,#15150,#8980,.T.);
#19193=EDGE_CURVE('',#15149,#15151,#8981,.T.);
#19194=EDGE_CURVE('',#15151,#15152,#8982,.T.);
#19195=EDGE_CURVE('',#15150,#15152,#8983,.T.);
#19196=EDGE_CURVE('',#15153,#15149,#8984,.T.);
#19197=EDGE_CURVE('',#15153,#15154,#8985,.T.);
#19198=EDGE_CURVE('',#15154,#15151,#8986,.T.);
#19199=EDGE_CURVE('',#15155,#15153,#8987,.T.);
#19200=EDGE_CURVE('',#15155,#15156,#8988,.T.);
#19201=EDGE_CURVE('',#15156,#15154,#8989,.T.);
#19202=EDGE_CURVE('',#15150,#15155,#8990,.T.);
#19203=EDGE_CURVE('',#15152,#15156,#8991,.T.);
#19204=EDGE_CURVE('',#15157,#15158,#8992,.T.);
#19205=EDGE_CURVE('',#15157,#15159,#8993,.T.);
#19206=EDGE_CURVE('',#15159,#15160,#8994,.T.);
#19207=EDGE_CURVE('',#15158,#15160,#8995,.T.);
#19208=EDGE_CURVE('',#15161,#15157,#8996,.T.);
#19209=EDGE_CURVE('',#15161,#15162,#8997,.T.);
#19210=EDGE_CURVE('',#15162,#15159,#8998,.T.);
#19211=EDGE_CURVE('',#15163,#15161,#8999,.T.);
#19212=EDGE_CURVE('',#15163,#15164,#9000,.T.);
#19213=EDGE_CURVE('',#15164,#15162,#9001,.T.);
#19214=EDGE_CURVE('',#15158,#15163,#9002,.T.);
#19215=EDGE_CURVE('',#15160,#15164,#9003,.T.);
#19216=EDGE_CURVE('',#15165,#15166,#9004,.T.);
#19217=EDGE_CURVE('',#15165,#15167,#9005,.T.);
#19218=EDGE_CURVE('',#15167,#15168,#9006,.T.);
#19219=EDGE_CURVE('',#15166,#15168,#9007,.T.);
#19220=EDGE_CURVE('',#15169,#15165,#9008,.T.);
#19221=EDGE_CURVE('',#15169,#15170,#9009,.T.);
#19222=EDGE_CURVE('',#15170,#15167,#9010,.T.);
#19223=EDGE_CURVE('',#15171,#15169,#9011,.T.);
#19224=EDGE_CURVE('',#15171,#15172,#9012,.T.);
#19225=EDGE_CURVE('',#15172,#15170,#9013,.T.);
#19226=EDGE_CURVE('',#15166,#15171,#9014,.T.);
#19227=EDGE_CURVE('',#15168,#15172,#9015,.T.);
#19228=EDGE_CURVE('',#15173,#15174,#9016,.T.);
#19229=EDGE_CURVE('',#15173,#15175,#9017,.T.);
#19230=EDGE_CURVE('',#15175,#15176,#9018,.T.);
#19231=EDGE_CURVE('',#15174,#15176,#9019,.T.);
#19232=EDGE_CURVE('',#15177,#15173,#9020,.T.);
#19233=EDGE_CURVE('',#15177,#15178,#9021,.T.);
#19234=EDGE_CURVE('',#15178,#15175,#9022,.T.);
#19235=EDGE_CURVE('',#15179,#15177,#9023,.T.);
#19236=EDGE_CURVE('',#15179,#15180,#9024,.T.);
#19237=EDGE_CURVE('',#15180,#15178,#9025,.T.);
#19238=EDGE_CURVE('',#15174,#15179,#9026,.T.);
#19239=EDGE_CURVE('',#15176,#15180,#9027,.T.);
#19240=EDGE_CURVE('',#15181,#15182,#9028,.T.);
#19241=EDGE_CURVE('',#15181,#15183,#9029,.T.);
#19242=EDGE_CURVE('',#15183,#15184,#9030,.T.);
#19243=EDGE_CURVE('',#15182,#15184,#9031,.T.);
#19244=EDGE_CURVE('',#15185,#15181,#9032,.T.);
#19245=EDGE_CURVE('',#15185,#15186,#9033,.T.);
#19246=EDGE_CURVE('',#15186,#15183,#9034,.T.);
#19247=EDGE_CURVE('',#15187,#15185,#9035,.T.);
#19248=EDGE_CURVE('',#15187,#15188,#9036,.T.);
#19249=EDGE_CURVE('',#15188,#15186,#9037,.T.);
#19250=EDGE_CURVE('',#15182,#15187,#9038,.T.);
#19251=EDGE_CURVE('',#15184,#15188,#9039,.T.);
#19252=EDGE_CURVE('',#15189,#15189,#12916,.T.);
#19253=EDGE_CURVE('',#15189,#15190,#9040,.T.);
#19254=EDGE_CURVE('',#15190,#15190,#12917,.T.);
#19255=EDGE_CURVE('',#15191,#15191,#12918,.T.);
#19256=EDGE_CURVE('',#15191,#15192,#9041,.T.);
#19257=EDGE_CURVE('',#15192,#15192,#12919,.T.);
#19258=EDGE_CURVE('',#15193,#15194,#9042,.T.);
#19259=EDGE_CURVE('',#15194,#15195,#9043,.T.);
#19260=EDGE_CURVE('',#15196,#15195,#9044,.T.);
#19261=EDGE_CURVE('',#15193,#15196,#9045,.T.);
#19262=EDGE_CURVE('',#15197,#15193,#12920,.T.);
#19263=EDGE_CURVE('',#15198,#15196,#12921,.T.);
#19264=EDGE_CURVE('',#15197,#15198,#9046,.T.);
#19265=EDGE_CURVE('',#15199,#15197,#9047,.T.);
#19266=EDGE_CURVE('',#15200,#15198,#9048,.T.);
#19267=EDGE_CURVE('',#15199,#15200,#9049,.T.);
#19268=EDGE_CURVE('',#15201,#15199,#12922,.T.);
#19269=EDGE_CURVE('',#15202,#15200,#12923,.T.);
#19270=EDGE_CURVE('',#15201,#15202,#9050,.T.);
#19271=EDGE_CURVE('',#15203,#15201,#9051,.T.);
#19272=EDGE_CURVE('',#15204,#15202,#9052,.T.);
#19273=EDGE_CURVE('',#15203,#15204,#9053,.T.);
#19274=EDGE_CURVE('',#15205,#15203,#12924,.T.);
#19275=EDGE_CURVE('',#15206,#15204,#12925,.T.);
#19276=EDGE_CURVE('',#15205,#15206,#9054,.T.);
#19277=EDGE_CURVE('',#15207,#15205,#9055,.T.);
#19278=EDGE_CURVE('',#15208,#15206,#9056,.T.);
#19279=EDGE_CURVE('',#15207,#15208,#9057,.T.);
#19280=EDGE_CURVE('',#15194,#15207,#12926,.T.);
#19281=EDGE_CURVE('',#15195,#15208,#12927,.T.);
#22782=ORIENTED_EDGE('',*,*,#17242,.F.);
#22783=ORIENTED_EDGE('',*,*,#17243,.T.);
#22784=ORIENTED_EDGE('',*,*,#17244,.T.);
#22785=ORIENTED_EDGE('',*,*,#17245,.F.);
#22786=ORIENTED_EDGE('',*,*,#17246,.F.);
#22787=ORIENTED_EDGE('',*,*,#17247,.T.);
#22788=ORIENTED_EDGE('',*,*,#17248,.T.);
#22789=ORIENTED_EDGE('',*,*,#17243,.F.);
#22790=ORIENTED_EDGE('',*,*,#17249,.F.);
#22791=ORIENTED_EDGE('',*,*,#17250,.T.);
#22792=ORIENTED_EDGE('',*,*,#17251,.T.);
#22793=ORIENTED_EDGE('',*,*,#17247,.F.);
#22794=ORIENTED_EDGE('',*,*,#17252,.F.);
#22795=ORIENTED_EDGE('',*,*,#17253,.T.);
#22796=ORIENTED_EDGE('',*,*,#17254,.T.);
#22797=ORIENTED_EDGE('',*,*,#17250,.F.);
#22798=ORIENTED_EDGE('',*,*,#17255,.F.);
#22799=ORIENTED_EDGE('',*,*,#17256,.T.);
#22800=ORIENTED_EDGE('',*,*,#17257,.T.);
#22801=ORIENTED_EDGE('',*,*,#17253,.F.);
#22802=ORIENTED_EDGE('',*,*,#17258,.F.);
#22803=ORIENTED_EDGE('',*,*,#17259,.T.);
#22804=ORIENTED_EDGE('',*,*,#17260,.T.);
#22805=ORIENTED_EDGE('',*,*,#17256,.F.);
#22806=ORIENTED_EDGE('',*,*,#17261,.F.);
#22807=ORIENTED_EDGE('',*,*,#17262,.T.);
#22808=ORIENTED_EDGE('',*,*,#17263,.T.);
#22809=ORIENTED_EDGE('',*,*,#17259,.F.);
#22810=ORIENTED_EDGE('',*,*,#17264,.F.);
#22811=ORIENTED_EDGE('',*,*,#17245,.T.);
#22812=ORIENTED_EDGE('',*,*,#17265,.T.);
#22813=ORIENTED_EDGE('',*,*,#17262,.F.);
#22814=ORIENTED_EDGE('',*,*,#17266,.F.);
#22815=ORIENTED_EDGE('',*,*,#17267,.T.);
#22816=ORIENTED_EDGE('',*,*,#17268,.T.);
#22817=ORIENTED_EDGE('',*,*,#17269,.F.);
#22818=ORIENTED_EDGE('',*,*,#17270,.F.);
#22819=ORIENTED_EDGE('',*,*,#17271,.T.);
#22820=ORIENTED_EDGE('',*,*,#17272,.T.);
#22821=ORIENTED_EDGE('',*,*,#17267,.F.);
#22822=ORIENTED_EDGE('',*,*,#17273,.F.);
#22823=ORIENTED_EDGE('',*,*,#17274,.T.);
#22824=ORIENTED_EDGE('',*,*,#17275,.T.);
#22825=ORIENTED_EDGE('',*,*,#17271,.F.);
#22826=ORIENTED_EDGE('',*,*,#17276,.F.);
#22827=ORIENTED_EDGE('',*,*,#17277,.T.);
#22828=ORIENTED_EDGE('',*,*,#17278,.T.);
#22829=ORIENTED_EDGE('',*,*,#17274,.F.);
#22830=ORIENTED_EDGE('',*,*,#17279,.F.);
#22831=ORIENTED_EDGE('',*,*,#17280,.T.);
#22832=ORIENTED_EDGE('',*,*,#17281,.T.);
#22833=ORIENTED_EDGE('',*,*,#17277,.F.);
#22834=ORIENTED_EDGE('',*,*,#17282,.F.);
#22835=ORIENTED_EDGE('',*,*,#17283,.T.);
#22836=ORIENTED_EDGE('',*,*,#17284,.T.);
#22837=ORIENTED_EDGE('',*,*,#17280,.F.);
#22838=ORIENTED_EDGE('',*,*,#17285,.F.);
#22839=ORIENTED_EDGE('',*,*,#17286,.T.);
#22840=ORIENTED_EDGE('',*,*,#17287,.T.);
#22841=ORIENTED_EDGE('',*,*,#17283,.F.);
#22842=ORIENTED_EDGE('',*,*,#17288,.F.);
#22843=ORIENTED_EDGE('',*,*,#17289,.T.);
#22844=ORIENTED_EDGE('',*,*,#17290,.T.);
#22845=ORIENTED_EDGE('',*,*,#17286,.F.);
#22846=ORIENTED_EDGE('',*,*,#17291,.F.);
#22847=ORIENTED_EDGE('',*,*,#17292,.T.);
#22848=ORIENTED_EDGE('',*,*,#17293,.T.);
#22849=ORIENTED_EDGE('',*,*,#17289,.F.);
#22850=ORIENTED_EDGE('',*,*,#17294,.F.);
#22851=ORIENTED_EDGE('',*,*,#17295,.T.);
#22852=ORIENTED_EDGE('',*,*,#17296,.T.);
#22853=ORIENTED_EDGE('',*,*,#17292,.F.);
#22854=ORIENTED_EDGE('',*,*,#17297,.F.);
#22855=ORIENTED_EDGE('',*,*,#17298,.T.);
#22856=ORIENTED_EDGE('',*,*,#17299,.T.);
#22857=ORIENTED_EDGE('',*,*,#17295,.F.);
#22858=ORIENTED_EDGE('',*,*,#17300,.F.);
#22859=ORIENTED_EDGE('',*,*,#17269,.T.);
#22860=ORIENTED_EDGE('',*,*,#17301,.T.);
#22861=ORIENTED_EDGE('',*,*,#17298,.F.);
#22862=ORIENTED_EDGE('',*,*,#17301,.F.);
#22863=ORIENTED_EDGE('',*,*,#17268,.F.);
#22864=ORIENTED_EDGE('',*,*,#17272,.F.);
#22865=ORIENTED_EDGE('',*,*,#17275,.F.);
#22866=ORIENTED_EDGE('',*,*,#17278,.F.);
#22867=ORIENTED_EDGE('',*,*,#17281,.F.);
#22868=ORIENTED_EDGE('',*,*,#17284,.F.);
#22869=ORIENTED_EDGE('',*,*,#17287,.F.);
#22870=ORIENTED_EDGE('',*,*,#17290,.F.);
#22871=ORIENTED_EDGE('',*,*,#17293,.F.);
#22872=ORIENTED_EDGE('',*,*,#17296,.F.);
#22873=ORIENTED_EDGE('',*,*,#17299,.F.);
#22874=ORIENTED_EDGE('',*,*,#17265,.F.);
#22875=ORIENTED_EDGE('',*,*,#17244,.F.);
#22876=ORIENTED_EDGE('',*,*,#17248,.F.);
#22877=ORIENTED_EDGE('',*,*,#17251,.F.);
#22878=ORIENTED_EDGE('',*,*,#17254,.F.);
#22879=ORIENTED_EDGE('',*,*,#17257,.F.);
#22880=ORIENTED_EDGE('',*,*,#17260,.F.);
#22881=ORIENTED_EDGE('',*,*,#17263,.F.);
#22882=ORIENTED_EDGE('',*,*,#17302,.F.);
#22883=ORIENTED_EDGE('',*,*,#17303,.T.);
#22884=ORIENTED_EDGE('',*,*,#17304,.T.);
#22885=ORIENTED_EDGE('',*,*,#17305,.F.);
#22886=ORIENTED_EDGE('',*,*,#17306,.F.);
#22887=ORIENTED_EDGE('',*,*,#17307,.T.);
#22888=ORIENTED_EDGE('',*,*,#17308,.T.);
#22889=ORIENTED_EDGE('',*,*,#17303,.F.);
#22890=ORIENTED_EDGE('',*,*,#17309,.F.);
#22891=ORIENTED_EDGE('',*,*,#17305,.T.);
#22892=ORIENTED_EDGE('',*,*,#17310,.T.);
#22893=ORIENTED_EDGE('',*,*,#17307,.F.);
#22894=ORIENTED_EDGE('',*,*,#17311,.F.);
#22895=ORIENTED_EDGE('',*,*,#17312,.T.);
#22896=ORIENTED_EDGE('',*,*,#17313,.T.);
#22897=ORIENTED_EDGE('',*,*,#17314,.F.);
#22898=ORIENTED_EDGE('',*,*,#17315,.F.);
#22899=ORIENTED_EDGE('',*,*,#17316,.T.);
#22900=ORIENTED_EDGE('',*,*,#17317,.T.);
#22901=ORIENTED_EDGE('',*,*,#17312,.F.);
#22902=ORIENTED_EDGE('',*,*,#17318,.F.);
#22903=ORIENTED_EDGE('',*,*,#17319,.T.);
#22904=ORIENTED_EDGE('',*,*,#17320,.T.);
#22905=ORIENTED_EDGE('',*,*,#17316,.F.);
#22906=ORIENTED_EDGE('',*,*,#17321,.F.);
#22907=ORIENTED_EDGE('',*,*,#17322,.T.);
#22908=ORIENTED_EDGE('',*,*,#17323,.T.);
#22909=ORIENTED_EDGE('',*,*,#17319,.F.);
#22910=ORIENTED_EDGE('',*,*,#17324,.F.);
#22911=ORIENTED_EDGE('',*,*,#17325,.T.);
#22912=ORIENTED_EDGE('',*,*,#17326,.T.);
#22913=ORIENTED_EDGE('',*,*,#17322,.F.);
#22914=ORIENTED_EDGE('',*,*,#17327,.F.);
#22915=ORIENTED_EDGE('',*,*,#17328,.T.);
#22916=ORIENTED_EDGE('',*,*,#17329,.T.);
#22917=ORIENTED_EDGE('',*,*,#17325,.F.);
#22918=ORIENTED_EDGE('',*,*,#17330,.F.);
#22919=ORIENTED_EDGE('',*,*,#17331,.T.);
#22920=ORIENTED_EDGE('',*,*,#17332,.T.);
#22921=ORIENTED_EDGE('',*,*,#17328,.F.);
#22922=ORIENTED_EDGE('',*,*,#17333,.F.);
#22923=ORIENTED_EDGE('',*,*,#17334,.T.);
#22924=ORIENTED_EDGE('',*,*,#17335,.T.);
#22925=ORIENTED_EDGE('',*,*,#17331,.F.);
#22926=ORIENTED_EDGE('',*,*,#17336,.F.);
#22927=ORIENTED_EDGE('',*,*,#17337,.T.);
#22928=ORIENTED_EDGE('',*,*,#17338,.T.);
#22929=ORIENTED_EDGE('',*,*,#17334,.F.);
#22930=ORIENTED_EDGE('',*,*,#17339,.F.);
#22931=ORIENTED_EDGE('',*,*,#17340,.T.);
#22932=ORIENTED_EDGE('',*,*,#17341,.T.);
#22933=ORIENTED_EDGE('',*,*,#17337,.F.);
#22934=ORIENTED_EDGE('',*,*,#17342,.F.);
#22935=ORIENTED_EDGE('',*,*,#17314,.T.);
#22936=ORIENTED_EDGE('',*,*,#17343,.T.);
#22937=ORIENTED_EDGE('',*,*,#17340,.F.);
#22938=ORIENTED_EDGE('',*,*,#17343,.F.);
#22939=ORIENTED_EDGE('',*,*,#17313,.F.);
#22940=ORIENTED_EDGE('',*,*,#17317,.F.);
#22941=ORIENTED_EDGE('',*,*,#17320,.F.);
#22942=ORIENTED_EDGE('',*,*,#17323,.F.);
#22943=ORIENTED_EDGE('',*,*,#17326,.F.);
#22944=ORIENTED_EDGE('',*,*,#17329,.F.);
#22945=ORIENTED_EDGE('',*,*,#17332,.F.);
#22946=ORIENTED_EDGE('',*,*,#17335,.F.);
#22947=ORIENTED_EDGE('',*,*,#17338,.F.);
#22948=ORIENTED_EDGE('',*,*,#17341,.F.);
#22949=ORIENTED_EDGE('',*,*,#17310,.F.);
#22950=ORIENTED_EDGE('',*,*,#17304,.F.);
#22951=ORIENTED_EDGE('',*,*,#17308,.F.);
#22952=ORIENTED_EDGE('',*,*,#17302,.T.);
#22953=ORIENTED_EDGE('',*,*,#17309,.T.);
#22954=ORIENTED_EDGE('',*,*,#17306,.T.);
#22955=ORIENTED_EDGE('',*,*,#17242,.T.);
#22956=ORIENTED_EDGE('',*,*,#17264,.T.);
#22957=ORIENTED_EDGE('',*,*,#17261,.T.);
#22958=ORIENTED_EDGE('',*,*,#17258,.T.);
#22959=ORIENTED_EDGE('',*,*,#17255,.T.);
#22960=ORIENTED_EDGE('',*,*,#17252,.T.);
#22961=ORIENTED_EDGE('',*,*,#17249,.T.);
#22962=ORIENTED_EDGE('',*,*,#17246,.T.);
#22963=ORIENTED_EDGE('',*,*,#17344,.F.);
#22964=ORIENTED_EDGE('',*,*,#17345,.T.);
#22965=ORIENTED_EDGE('',*,*,#17346,.T.);
#22966=ORIENTED_EDGE('',*,*,#17347,.F.);
#22967=ORIENTED_EDGE('',*,*,#17348,.F.);
#22968=ORIENTED_EDGE('',*,*,#17349,.T.);
#22969=ORIENTED_EDGE('',*,*,#17350,.T.);
#22970=ORIENTED_EDGE('',*,*,#17345,.F.);
#22971=ORIENTED_EDGE('',*,*,#17351,.F.);
#22972=ORIENTED_EDGE('',*,*,#17352,.T.);
#22973=ORIENTED_EDGE('',*,*,#17353,.T.);
#22974=ORIENTED_EDGE('',*,*,#17349,.F.);
#22975=ORIENTED_EDGE('',*,*,#17354,.F.);
#22976=ORIENTED_EDGE('',*,*,#17355,.T.);
#22977=ORIENTED_EDGE('',*,*,#17356,.T.);
#22978=ORIENTED_EDGE('',*,*,#17352,.F.);
#22979=ORIENTED_EDGE('',*,*,#17357,.F.);
#22980=ORIENTED_EDGE('',*,*,#17358,.T.);
#22981=ORIENTED_EDGE('',*,*,#17359,.T.);
#22982=ORIENTED_EDGE('',*,*,#17355,.F.);
#22983=ORIENTED_EDGE('',*,*,#17360,.F.);
#22984=ORIENTED_EDGE('',*,*,#17361,.T.);
#22985=ORIENTED_EDGE('',*,*,#17362,.T.);
#22986=ORIENTED_EDGE('',*,*,#17358,.F.);
#22987=ORIENTED_EDGE('',*,*,#17363,.F.);
#22988=ORIENTED_EDGE('',*,*,#17364,.T.);
#22989=ORIENTED_EDGE('',*,*,#17365,.T.);
#22990=ORIENTED_EDGE('',*,*,#17361,.F.);
#22991=ORIENTED_EDGE('',*,*,#17366,.F.);
#22992=ORIENTED_EDGE('',*,*,#17347,.T.);
#22993=ORIENTED_EDGE('',*,*,#17367,.T.);
#22994=ORIENTED_EDGE('',*,*,#17364,.F.);
#22995=ORIENTED_EDGE('',*,*,#17368,.F.);
#22996=ORIENTED_EDGE('',*,*,#17369,.T.);
#22997=ORIENTED_EDGE('',*,*,#17370,.T.);
#22998=ORIENTED_EDGE('',*,*,#17371,.F.);
#22999=ORIENTED_EDGE('',*,*,#17372,.F.);
#23000=ORIENTED_EDGE('',*,*,#17373,.T.);
#23001=ORIENTED_EDGE('',*,*,#17374,.T.);
#23002=ORIENTED_EDGE('',*,*,#17369,.F.);
#23003=ORIENTED_EDGE('',*,*,#17375,.F.);
#23004=ORIENTED_EDGE('',*,*,#17376,.T.);
#23005=ORIENTED_EDGE('',*,*,#17377,.T.);
#23006=ORIENTED_EDGE('',*,*,#17373,.F.);
#23007=ORIENTED_EDGE('',*,*,#17378,.F.);
#23008=ORIENTED_EDGE('',*,*,#17379,.T.);
#23009=ORIENTED_EDGE('',*,*,#17380,.T.);
#23010=ORIENTED_EDGE('',*,*,#17376,.F.);
#23011=ORIENTED_EDGE('',*,*,#17381,.F.);
#23012=ORIENTED_EDGE('',*,*,#17382,.T.);
#23013=ORIENTED_EDGE('',*,*,#17383,.T.);
#23014=ORIENTED_EDGE('',*,*,#17379,.F.);
#23015=ORIENTED_EDGE('',*,*,#17384,.F.);
#23016=ORIENTED_EDGE('',*,*,#17385,.T.);
#23017=ORIENTED_EDGE('',*,*,#17386,.T.);
#23018=ORIENTED_EDGE('',*,*,#17382,.F.);
#23019=ORIENTED_EDGE('',*,*,#17387,.F.);
#23020=ORIENTED_EDGE('',*,*,#17388,.T.);
#23021=ORIENTED_EDGE('',*,*,#17389,.T.);
#23022=ORIENTED_EDGE('',*,*,#17385,.F.);
#23023=ORIENTED_EDGE('',*,*,#17390,.F.);
#23024=ORIENTED_EDGE('',*,*,#17391,.T.);
#23025=ORIENTED_EDGE('',*,*,#17392,.T.);
#23026=ORIENTED_EDGE('',*,*,#17388,.F.);
#23027=ORIENTED_EDGE('',*,*,#17393,.F.);
#23028=ORIENTED_EDGE('',*,*,#17394,.T.);
#23029=ORIENTED_EDGE('',*,*,#17395,.T.);
#23030=ORIENTED_EDGE('',*,*,#17391,.F.);
#23031=ORIENTED_EDGE('',*,*,#17396,.F.);
#23032=ORIENTED_EDGE('',*,*,#17397,.T.);
#23033=ORIENTED_EDGE('',*,*,#17398,.T.);
#23034=ORIENTED_EDGE('',*,*,#17394,.F.);
#23035=ORIENTED_EDGE('',*,*,#17399,.F.);
#23036=ORIENTED_EDGE('',*,*,#17400,.T.);
#23037=ORIENTED_EDGE('',*,*,#17401,.T.);
#23038=ORIENTED_EDGE('',*,*,#17397,.F.);
#23039=ORIENTED_EDGE('',*,*,#17402,.F.);
#23040=ORIENTED_EDGE('',*,*,#17371,.T.);
#23041=ORIENTED_EDGE('',*,*,#17403,.T.);
#23042=ORIENTED_EDGE('',*,*,#17400,.F.);
#23043=ORIENTED_EDGE('',*,*,#17403,.F.);
#23044=ORIENTED_EDGE('',*,*,#17370,.F.);
#23045=ORIENTED_EDGE('',*,*,#17374,.F.);
#23046=ORIENTED_EDGE('',*,*,#17377,.F.);
#23047=ORIENTED_EDGE('',*,*,#17380,.F.);
#23048=ORIENTED_EDGE('',*,*,#17383,.F.);
#23049=ORIENTED_EDGE('',*,*,#17386,.F.);
#23050=ORIENTED_EDGE('',*,*,#17389,.F.);
#23051=ORIENTED_EDGE('',*,*,#17392,.F.);
#23052=ORIENTED_EDGE('',*,*,#17395,.F.);
#23053=ORIENTED_EDGE('',*,*,#17398,.F.);
#23054=ORIENTED_EDGE('',*,*,#17401,.F.);
#23055=ORIENTED_EDGE('',*,*,#17367,.F.);
#23056=ORIENTED_EDGE('',*,*,#17346,.F.);
#23057=ORIENTED_EDGE('',*,*,#17350,.F.);
#23058=ORIENTED_EDGE('',*,*,#17353,.F.);
#23059=ORIENTED_EDGE('',*,*,#17356,.F.);
#23060=ORIENTED_EDGE('',*,*,#17359,.F.);
#23061=ORIENTED_EDGE('',*,*,#17362,.F.);
#23062=ORIENTED_EDGE('',*,*,#17365,.F.);
#23063=ORIENTED_EDGE('',*,*,#17404,.F.);
#23064=ORIENTED_EDGE('',*,*,#17405,.T.);
#23065=ORIENTED_EDGE('',*,*,#17406,.T.);
#23066=ORIENTED_EDGE('',*,*,#17407,.F.);
#23067=ORIENTED_EDGE('',*,*,#17408,.F.);
#23068=ORIENTED_EDGE('',*,*,#17409,.T.);
#23069=ORIENTED_EDGE('',*,*,#17410,.T.);
#23070=ORIENTED_EDGE('',*,*,#17405,.F.);
#23071=ORIENTED_EDGE('',*,*,#17411,.F.);
#23072=ORIENTED_EDGE('',*,*,#17412,.T.);
#23073=ORIENTED_EDGE('',*,*,#17413,.T.);
#23074=ORIENTED_EDGE('',*,*,#17409,.F.);
#23075=ORIENTED_EDGE('',*,*,#17414,.F.);
#23076=ORIENTED_EDGE('',*,*,#17415,.T.);
#23077=ORIENTED_EDGE('',*,*,#17416,.T.);
#23078=ORIENTED_EDGE('',*,*,#17412,.F.);
#23079=ORIENTED_EDGE('',*,*,#17417,.F.);
#23080=ORIENTED_EDGE('',*,*,#17418,.T.);
#23081=ORIENTED_EDGE('',*,*,#17419,.T.);
#23082=ORIENTED_EDGE('',*,*,#17415,.F.);
#23083=ORIENTED_EDGE('',*,*,#17420,.F.);
#23084=ORIENTED_EDGE('',*,*,#17421,.T.);
#23085=ORIENTED_EDGE('',*,*,#17422,.T.);
#23086=ORIENTED_EDGE('',*,*,#17418,.F.);
#23087=ORIENTED_EDGE('',*,*,#17423,.F.);
#23088=ORIENTED_EDGE('',*,*,#17424,.T.);
#23089=ORIENTED_EDGE('',*,*,#17425,.T.);
#23090=ORIENTED_EDGE('',*,*,#17421,.F.);
#23091=ORIENTED_EDGE('',*,*,#17426,.F.);
#23092=ORIENTED_EDGE('',*,*,#17427,.T.);
#23093=ORIENTED_EDGE('',*,*,#17428,.T.);
#23094=ORIENTED_EDGE('',*,*,#17424,.F.);
#23095=ORIENTED_EDGE('',*,*,#17429,.F.);
#23096=ORIENTED_EDGE('',*,*,#17430,.T.);
#23097=ORIENTED_EDGE('',*,*,#17431,.T.);
#23098=ORIENTED_EDGE('',*,*,#17427,.F.);
#23099=ORIENTED_EDGE('',*,*,#17432,.F.);
#23100=ORIENTED_EDGE('',*,*,#17433,.T.);
#23101=ORIENTED_EDGE('',*,*,#17434,.T.);
#23102=ORIENTED_EDGE('',*,*,#17430,.F.);
#23103=ORIENTED_EDGE('',*,*,#17435,.F.);
#23104=ORIENTED_EDGE('',*,*,#17436,.T.);
#23105=ORIENTED_EDGE('',*,*,#17437,.T.);
#23106=ORIENTED_EDGE('',*,*,#17433,.F.);
#23107=ORIENTED_EDGE('',*,*,#17438,.F.);
#23108=ORIENTED_EDGE('',*,*,#17439,.T.);
#23109=ORIENTED_EDGE('',*,*,#17440,.T.);
#23110=ORIENTED_EDGE('',*,*,#17436,.F.);
#23111=ORIENTED_EDGE('',*,*,#17441,.F.);
#23112=ORIENTED_EDGE('',*,*,#17442,.T.);
#23113=ORIENTED_EDGE('',*,*,#17443,.T.);
#23114=ORIENTED_EDGE('',*,*,#17439,.F.);
#23115=ORIENTED_EDGE('',*,*,#17444,.F.);
#23116=ORIENTED_EDGE('',*,*,#17445,.T.);
#23117=ORIENTED_EDGE('',*,*,#17446,.T.);
#23118=ORIENTED_EDGE('',*,*,#17442,.F.);
#23119=ORIENTED_EDGE('',*,*,#17447,.F.);
#23120=ORIENTED_EDGE('',*,*,#17448,.T.);
#23121=ORIENTED_EDGE('',*,*,#17449,.T.);
#23122=ORIENTED_EDGE('',*,*,#17445,.F.);
#23123=ORIENTED_EDGE('',*,*,#17450,.F.);
#23124=ORIENTED_EDGE('',*,*,#17451,.T.);
#23125=ORIENTED_EDGE('',*,*,#17452,.T.);
#23126=ORIENTED_EDGE('',*,*,#17448,.F.);
#23127=ORIENTED_EDGE('',*,*,#17453,.F.);
#23128=ORIENTED_EDGE('',*,*,#17454,.T.);
#23129=ORIENTED_EDGE('',*,*,#17455,.T.);
#23130=ORIENTED_EDGE('',*,*,#17451,.F.);
#23131=ORIENTED_EDGE('',*,*,#17456,.F.);
#23132=ORIENTED_EDGE('',*,*,#17457,.T.);
#23133=ORIENTED_EDGE('',*,*,#17458,.T.);
#23134=ORIENTED_EDGE('',*,*,#17454,.F.);
#23135=ORIENTED_EDGE('',*,*,#17459,.F.);
#23136=ORIENTED_EDGE('',*,*,#17460,.T.);
#23137=ORIENTED_EDGE('',*,*,#17461,.T.);
#23138=ORIENTED_EDGE('',*,*,#17457,.F.);
#23139=ORIENTED_EDGE('',*,*,#17462,.F.);
#23140=ORIENTED_EDGE('',*,*,#17463,.T.);
#23141=ORIENTED_EDGE('',*,*,#17464,.T.);
#23142=ORIENTED_EDGE('',*,*,#17460,.F.);
#23143=ORIENTED_EDGE('',*,*,#17465,.F.);
#23144=ORIENTED_EDGE('',*,*,#17466,.T.);
#23145=ORIENTED_EDGE('',*,*,#17467,.T.);
#23146=ORIENTED_EDGE('',*,*,#17463,.F.);
#23147=ORIENTED_EDGE('',*,*,#17468,.F.);
#23148=ORIENTED_EDGE('',*,*,#17469,.T.);
#23149=ORIENTED_EDGE('',*,*,#17470,.T.);
#23150=ORIENTED_EDGE('',*,*,#17466,.F.);
#23151=ORIENTED_EDGE('',*,*,#17471,.F.);
#23152=ORIENTED_EDGE('',*,*,#17472,.T.);
#23153=ORIENTED_EDGE('',*,*,#17473,.T.);
#23154=ORIENTED_EDGE('',*,*,#17469,.F.);
#23155=ORIENTED_EDGE('',*,*,#17474,.F.);
#23156=ORIENTED_EDGE('',*,*,#17475,.T.);
#23157=ORIENTED_EDGE('',*,*,#17476,.T.);
#23158=ORIENTED_EDGE('',*,*,#17472,.F.);
#23159=ORIENTED_EDGE('',*,*,#17477,.F.);
#23160=ORIENTED_EDGE('',*,*,#17478,.T.);
#23161=ORIENTED_EDGE('',*,*,#17479,.T.);
#23162=ORIENTED_EDGE('',*,*,#17475,.F.);
#23163=ORIENTED_EDGE('',*,*,#17480,.F.);
#23164=ORIENTED_EDGE('',*,*,#17481,.T.);
#23165=ORIENTED_EDGE('',*,*,#17482,.T.);
#23166=ORIENTED_EDGE('',*,*,#17478,.F.);
#23167=ORIENTED_EDGE('',*,*,#17483,.F.);
#23168=ORIENTED_EDGE('',*,*,#17484,.T.);
#23169=ORIENTED_EDGE('',*,*,#17485,.T.);
#23170=ORIENTED_EDGE('',*,*,#17481,.F.);
#23171=ORIENTED_EDGE('',*,*,#17486,.F.);
#23172=ORIENTED_EDGE('',*,*,#17487,.T.);
#23173=ORIENTED_EDGE('',*,*,#17488,.T.);
#23174=ORIENTED_EDGE('',*,*,#17484,.F.);
#23175=ORIENTED_EDGE('',*,*,#17489,.F.);
#23176=ORIENTED_EDGE('',*,*,#17490,.T.);
#23177=ORIENTED_EDGE('',*,*,#17491,.T.);
#23178=ORIENTED_EDGE('',*,*,#17487,.F.);
#23179=ORIENTED_EDGE('',*,*,#17492,.F.);
#23180=ORIENTED_EDGE('',*,*,#17407,.T.);
#23181=ORIENTED_EDGE('',*,*,#17493,.T.);
#23182=ORIENTED_EDGE('',*,*,#17490,.F.);
#23183=ORIENTED_EDGE('',*,*,#17493,.F.);
#23184=ORIENTED_EDGE('',*,*,#17406,.F.);
#23185=ORIENTED_EDGE('',*,*,#17410,.F.);
#23186=ORIENTED_EDGE('',*,*,#17413,.F.);
#23187=ORIENTED_EDGE('',*,*,#17416,.F.);
#23188=ORIENTED_EDGE('',*,*,#17419,.F.);
#23189=ORIENTED_EDGE('',*,*,#17422,.F.);
#23190=ORIENTED_EDGE('',*,*,#17425,.F.);
#23191=ORIENTED_EDGE('',*,*,#17428,.F.);
#23192=ORIENTED_EDGE('',*,*,#17431,.F.);
#23193=ORIENTED_EDGE('',*,*,#17434,.F.);
#23194=ORIENTED_EDGE('',*,*,#17437,.F.);
#23195=ORIENTED_EDGE('',*,*,#17440,.F.);
#23196=ORIENTED_EDGE('',*,*,#17443,.F.);
#23197=ORIENTED_EDGE('',*,*,#17446,.F.);
#23198=ORIENTED_EDGE('',*,*,#17449,.F.);
#23199=ORIENTED_EDGE('',*,*,#17452,.F.);
#23200=ORIENTED_EDGE('',*,*,#17455,.F.);
#23201=ORIENTED_EDGE('',*,*,#17458,.F.);
#23202=ORIENTED_EDGE('',*,*,#17461,.F.);
#23203=ORIENTED_EDGE('',*,*,#17464,.F.);
#23204=ORIENTED_EDGE('',*,*,#17467,.F.);
#23205=ORIENTED_EDGE('',*,*,#17470,.F.);
#23206=ORIENTED_EDGE('',*,*,#17473,.F.);
#23207=ORIENTED_EDGE('',*,*,#17476,.F.);
#23208=ORIENTED_EDGE('',*,*,#17479,.F.);
#23209=ORIENTED_EDGE('',*,*,#17482,.F.);
#23210=ORIENTED_EDGE('',*,*,#17485,.F.);
#23211=ORIENTED_EDGE('',*,*,#17488,.F.);
#23212=ORIENTED_EDGE('',*,*,#17491,.F.);
#23213=ORIENTED_EDGE('',*,*,#17344,.T.);
#23214=ORIENTED_EDGE('',*,*,#17366,.T.);
#23215=ORIENTED_EDGE('',*,*,#17363,.T.);
#23216=ORIENTED_EDGE('',*,*,#17360,.T.);
#23217=ORIENTED_EDGE('',*,*,#17357,.T.);
#23218=ORIENTED_EDGE('',*,*,#17354,.T.);
#23219=ORIENTED_EDGE('',*,*,#17351,.T.);
#23220=ORIENTED_EDGE('',*,*,#17348,.T.);
#23221=ORIENTED_EDGE('',*,*,#17494,.F.);
#23222=ORIENTED_EDGE('',*,*,#17495,.T.);
#23223=ORIENTED_EDGE('',*,*,#17496,.T.);
#23224=ORIENTED_EDGE('',*,*,#17497,.F.);
#23225=ORIENTED_EDGE('',*,*,#17498,.F.);
#23226=ORIENTED_EDGE('',*,*,#17499,.T.);
#23227=ORIENTED_EDGE('',*,*,#17500,.T.);
#23228=ORIENTED_EDGE('',*,*,#17495,.F.);
#23229=ORIENTED_EDGE('',*,*,#17501,.F.);
#23230=ORIENTED_EDGE('',*,*,#17502,.T.);
#23231=ORIENTED_EDGE('',*,*,#17503,.T.);
#23232=ORIENTED_EDGE('',*,*,#17499,.F.);
#23233=ORIENTED_EDGE('',*,*,#17504,.F.);
#23234=ORIENTED_EDGE('',*,*,#17505,.T.);
#23235=ORIENTED_EDGE('',*,*,#17506,.T.);
#23236=ORIENTED_EDGE('',*,*,#17502,.F.);
#23237=ORIENTED_EDGE('',*,*,#17507,.F.);
#23238=ORIENTED_EDGE('',*,*,#17508,.T.);
#23239=ORIENTED_EDGE('',*,*,#17509,.T.);
#23240=ORIENTED_EDGE('',*,*,#17505,.F.);
#23241=ORIENTED_EDGE('',*,*,#17510,.F.);
#23242=ORIENTED_EDGE('',*,*,#17511,.T.);
#23243=ORIENTED_EDGE('',*,*,#17512,.T.);
#23244=ORIENTED_EDGE('',*,*,#17508,.F.);
#23245=ORIENTED_EDGE('',*,*,#17513,.F.);
#23246=ORIENTED_EDGE('',*,*,#17514,.T.);
#23247=ORIENTED_EDGE('',*,*,#17515,.T.);
#23248=ORIENTED_EDGE('',*,*,#17511,.F.);
#23249=ORIENTED_EDGE('',*,*,#17516,.F.);
#23250=ORIENTED_EDGE('',*,*,#17497,.T.);
#23251=ORIENTED_EDGE('',*,*,#17517,.T.);
#23252=ORIENTED_EDGE('',*,*,#17514,.F.);
#23253=ORIENTED_EDGE('',*,*,#17518,.F.);
#23254=ORIENTED_EDGE('',*,*,#17519,.T.);
#23255=ORIENTED_EDGE('',*,*,#17520,.T.);
#23256=ORIENTED_EDGE('',*,*,#17521,.F.);
#23257=ORIENTED_EDGE('',*,*,#17522,.F.);
#23258=ORIENTED_EDGE('',*,*,#17523,.T.);
#23259=ORIENTED_EDGE('',*,*,#17524,.T.);
#23260=ORIENTED_EDGE('',*,*,#17519,.F.);
#23261=ORIENTED_EDGE('',*,*,#17525,.F.);
#23262=ORIENTED_EDGE('',*,*,#17526,.T.);
#23263=ORIENTED_EDGE('',*,*,#17527,.T.);
#23264=ORIENTED_EDGE('',*,*,#17523,.F.);
#23265=ORIENTED_EDGE('',*,*,#17528,.F.);
#23266=ORIENTED_EDGE('',*,*,#17529,.T.);
#23267=ORIENTED_EDGE('',*,*,#17530,.T.);
#23268=ORIENTED_EDGE('',*,*,#17526,.F.);
#23269=ORIENTED_EDGE('',*,*,#17531,.F.);
#23270=ORIENTED_EDGE('',*,*,#17532,.T.);
#23271=ORIENTED_EDGE('',*,*,#17533,.T.);
#23272=ORIENTED_EDGE('',*,*,#17529,.F.);
#23273=ORIENTED_EDGE('',*,*,#17534,.F.);
#23274=ORIENTED_EDGE('',*,*,#17535,.T.);
#23275=ORIENTED_EDGE('',*,*,#17536,.T.);
#23276=ORIENTED_EDGE('',*,*,#17532,.F.);
#23277=ORIENTED_EDGE('',*,*,#17537,.F.);
#23278=ORIENTED_EDGE('',*,*,#17538,.T.);
#23279=ORIENTED_EDGE('',*,*,#17539,.T.);
#23280=ORIENTED_EDGE('',*,*,#17535,.F.);
#23281=ORIENTED_EDGE('',*,*,#17540,.F.);
#23282=ORIENTED_EDGE('',*,*,#17541,.T.);
#23283=ORIENTED_EDGE('',*,*,#17542,.T.);
#23284=ORIENTED_EDGE('',*,*,#17538,.F.);
#23285=ORIENTED_EDGE('',*,*,#17543,.F.);
#23286=ORIENTED_EDGE('',*,*,#17544,.T.);
#23287=ORIENTED_EDGE('',*,*,#17545,.T.);
#23288=ORIENTED_EDGE('',*,*,#17541,.F.);
#23289=ORIENTED_EDGE('',*,*,#17546,.F.);
#23290=ORIENTED_EDGE('',*,*,#17547,.T.);
#23291=ORIENTED_EDGE('',*,*,#17548,.T.);
#23292=ORIENTED_EDGE('',*,*,#17544,.F.);
#23293=ORIENTED_EDGE('',*,*,#17549,.F.);
#23294=ORIENTED_EDGE('',*,*,#17550,.T.);
#23295=ORIENTED_EDGE('',*,*,#17551,.T.);
#23296=ORIENTED_EDGE('',*,*,#17547,.F.);
#23297=ORIENTED_EDGE('',*,*,#17552,.F.);
#23298=ORIENTED_EDGE('',*,*,#17521,.T.);
#23299=ORIENTED_EDGE('',*,*,#17553,.T.);
#23300=ORIENTED_EDGE('',*,*,#17550,.F.);
#23301=ORIENTED_EDGE('',*,*,#17553,.F.);
#23302=ORIENTED_EDGE('',*,*,#17520,.F.);
#23303=ORIENTED_EDGE('',*,*,#17524,.F.);
#23304=ORIENTED_EDGE('',*,*,#17527,.F.);
#23305=ORIENTED_EDGE('',*,*,#17530,.F.);
#23306=ORIENTED_EDGE('',*,*,#17533,.F.);
#23307=ORIENTED_EDGE('',*,*,#17536,.F.);
#23308=ORIENTED_EDGE('',*,*,#17539,.F.);
#23309=ORIENTED_EDGE('',*,*,#17542,.F.);
#23310=ORIENTED_EDGE('',*,*,#17545,.F.);
#23311=ORIENTED_EDGE('',*,*,#17548,.F.);
#23312=ORIENTED_EDGE('',*,*,#17551,.F.);
#23313=ORIENTED_EDGE('',*,*,#17517,.F.);
#23314=ORIENTED_EDGE('',*,*,#17496,.F.);
#23315=ORIENTED_EDGE('',*,*,#17500,.F.);
#23316=ORIENTED_EDGE('',*,*,#17503,.F.);
#23317=ORIENTED_EDGE('',*,*,#17506,.F.);
#23318=ORIENTED_EDGE('',*,*,#17509,.F.);
#23319=ORIENTED_EDGE('',*,*,#17512,.F.);
#23320=ORIENTED_EDGE('',*,*,#17515,.F.);
#23321=ORIENTED_EDGE('',*,*,#17554,.F.);
#23322=ORIENTED_EDGE('',*,*,#17555,.T.);
#23323=ORIENTED_EDGE('',*,*,#17556,.T.);
#23324=ORIENTED_EDGE('',*,*,#17557,.F.);
#23325=ORIENTED_EDGE('',*,*,#17558,.F.);
#23326=ORIENTED_EDGE('',*,*,#17559,.T.);
#23327=ORIENTED_EDGE('',*,*,#17560,.T.);
#23328=ORIENTED_EDGE('',*,*,#17555,.F.);
#23329=ORIENTED_EDGE('',*,*,#17561,.F.);
#23330=ORIENTED_EDGE('',*,*,#17562,.T.);
#23331=ORIENTED_EDGE('',*,*,#17563,.T.);
#23332=ORIENTED_EDGE('',*,*,#17559,.F.);
#23333=ORIENTED_EDGE('',*,*,#17564,.F.);
#23334=ORIENTED_EDGE('',*,*,#17565,.T.);
#23335=ORIENTED_EDGE('',*,*,#17566,.T.);
#23336=ORIENTED_EDGE('',*,*,#17562,.F.);
#23337=ORIENTED_EDGE('',*,*,#17567,.F.);
#23338=ORIENTED_EDGE('',*,*,#17568,.T.);
#23339=ORIENTED_EDGE('',*,*,#17569,.T.);
#23340=ORIENTED_EDGE('',*,*,#17565,.F.);
#23341=ORIENTED_EDGE('',*,*,#17570,.F.);
#23342=ORIENTED_EDGE('',*,*,#17571,.T.);
#23343=ORIENTED_EDGE('',*,*,#17572,.T.);
#23344=ORIENTED_EDGE('',*,*,#17568,.F.);
#23345=ORIENTED_EDGE('',*,*,#17573,.F.);
#23346=ORIENTED_EDGE('',*,*,#17574,.T.);
#23347=ORIENTED_EDGE('',*,*,#17575,.T.);
#23348=ORIENTED_EDGE('',*,*,#17571,.F.);
#23349=ORIENTED_EDGE('',*,*,#17576,.F.);
#23350=ORIENTED_EDGE('',*,*,#17577,.T.);
#23351=ORIENTED_EDGE('',*,*,#17578,.T.);
#23352=ORIENTED_EDGE('',*,*,#17574,.F.);
#23353=ORIENTED_EDGE('',*,*,#17579,.F.);
#23354=ORIENTED_EDGE('',*,*,#17580,.T.);
#23355=ORIENTED_EDGE('',*,*,#17581,.T.);
#23356=ORIENTED_EDGE('',*,*,#17577,.F.);
#23357=ORIENTED_EDGE('',*,*,#17582,.F.);
#23358=ORIENTED_EDGE('',*,*,#17583,.T.);
#23359=ORIENTED_EDGE('',*,*,#17584,.T.);
#23360=ORIENTED_EDGE('',*,*,#17580,.F.);
#23361=ORIENTED_EDGE('',*,*,#17585,.F.);
#23362=ORIENTED_EDGE('',*,*,#17586,.T.);
#23363=ORIENTED_EDGE('',*,*,#17587,.T.);
#23364=ORIENTED_EDGE('',*,*,#17583,.F.);
#23365=ORIENTED_EDGE('',*,*,#17588,.F.);
#23366=ORIENTED_EDGE('',*,*,#17589,.T.);
#23367=ORIENTED_EDGE('',*,*,#17590,.T.);
#23368=ORIENTED_EDGE('',*,*,#17586,.F.);
#23369=ORIENTED_EDGE('',*,*,#17591,.F.);
#23370=ORIENTED_EDGE('',*,*,#17592,.T.);
#23371=ORIENTED_EDGE('',*,*,#17593,.T.);
#23372=ORIENTED_EDGE('',*,*,#17589,.F.);
#23373=ORIENTED_EDGE('',*,*,#17594,.F.);
#23374=ORIENTED_EDGE('',*,*,#17595,.T.);
#23375=ORIENTED_EDGE('',*,*,#17596,.T.);
#23376=ORIENTED_EDGE('',*,*,#17592,.F.);
#23377=ORIENTED_EDGE('',*,*,#17597,.F.);
#23378=ORIENTED_EDGE('',*,*,#17598,.T.);
#23379=ORIENTED_EDGE('',*,*,#17599,.T.);
#23380=ORIENTED_EDGE('',*,*,#17595,.F.);
#23381=ORIENTED_EDGE('',*,*,#17600,.F.);
#23382=ORIENTED_EDGE('',*,*,#17601,.T.);
#23383=ORIENTED_EDGE('',*,*,#17602,.T.);
#23384=ORIENTED_EDGE('',*,*,#17598,.F.);
#23385=ORIENTED_EDGE('',*,*,#17603,.F.);
#23386=ORIENTED_EDGE('',*,*,#17604,.T.);
#23387=ORIENTED_EDGE('',*,*,#17605,.T.);
#23388=ORIENTED_EDGE('',*,*,#17601,.F.);
#23389=ORIENTED_EDGE('',*,*,#17606,.F.);
#23390=ORIENTED_EDGE('',*,*,#17607,.T.);
#23391=ORIENTED_EDGE('',*,*,#17608,.T.);
#23392=ORIENTED_EDGE('',*,*,#17604,.F.);
#23393=ORIENTED_EDGE('',*,*,#17609,.F.);
#23394=ORIENTED_EDGE('',*,*,#17610,.T.);
#23395=ORIENTED_EDGE('',*,*,#17611,.T.);
#23396=ORIENTED_EDGE('',*,*,#17607,.F.);
#23397=ORIENTED_EDGE('',*,*,#17612,.F.);
#23398=ORIENTED_EDGE('',*,*,#17613,.T.);
#23399=ORIENTED_EDGE('',*,*,#17614,.T.);
#23400=ORIENTED_EDGE('',*,*,#17610,.F.);
#23401=ORIENTED_EDGE('',*,*,#17615,.F.);
#23402=ORIENTED_EDGE('',*,*,#17616,.T.);
#23403=ORIENTED_EDGE('',*,*,#17617,.T.);
#23404=ORIENTED_EDGE('',*,*,#17613,.F.);
#23405=ORIENTED_EDGE('',*,*,#17618,.F.);
#23406=ORIENTED_EDGE('',*,*,#17557,.T.);
#23407=ORIENTED_EDGE('',*,*,#17619,.T.);
#23408=ORIENTED_EDGE('',*,*,#17616,.F.);
#23409=ORIENTED_EDGE('',*,*,#17619,.F.);
#23410=ORIENTED_EDGE('',*,*,#17556,.F.);
#23411=ORIENTED_EDGE('',*,*,#17560,.F.);
#23412=ORIENTED_EDGE('',*,*,#17563,.F.);
#23413=ORIENTED_EDGE('',*,*,#17566,.F.);
#23414=ORIENTED_EDGE('',*,*,#17569,.F.);
#23415=ORIENTED_EDGE('',*,*,#17572,.F.);
#23416=ORIENTED_EDGE('',*,*,#17575,.F.);
#23417=ORIENTED_EDGE('',*,*,#17578,.F.);
#23418=ORIENTED_EDGE('',*,*,#17581,.F.);
#23419=ORIENTED_EDGE('',*,*,#17584,.F.);
#23420=ORIENTED_EDGE('',*,*,#17587,.F.);
#23421=ORIENTED_EDGE('',*,*,#17590,.F.);
#23422=ORIENTED_EDGE('',*,*,#17593,.F.);
#23423=ORIENTED_EDGE('',*,*,#17596,.F.);
#23424=ORIENTED_EDGE('',*,*,#17599,.F.);
#23425=ORIENTED_EDGE('',*,*,#17602,.F.);
#23426=ORIENTED_EDGE('',*,*,#17605,.F.);
#23427=ORIENTED_EDGE('',*,*,#17608,.F.);
#23428=ORIENTED_EDGE('',*,*,#17611,.F.);
#23429=ORIENTED_EDGE('',*,*,#17614,.F.);
#23430=ORIENTED_EDGE('',*,*,#17617,.F.);
#23431=ORIENTED_EDGE('',*,*,#17494,.T.);
#23432=ORIENTED_EDGE('',*,*,#17516,.T.);
#23433=ORIENTED_EDGE('',*,*,#17513,.T.);
#23434=ORIENTED_EDGE('',*,*,#17510,.T.);
#23435=ORIENTED_EDGE('',*,*,#17507,.T.);
#23436=ORIENTED_EDGE('',*,*,#17504,.T.);
#23437=ORIENTED_EDGE('',*,*,#17501,.T.);
#23438=ORIENTED_EDGE('',*,*,#17498,.T.);
#23439=ORIENTED_EDGE('',*,*,#17620,.F.);
#23440=ORIENTED_EDGE('',*,*,#17621,.T.);
#23441=ORIENTED_EDGE('',*,*,#17622,.T.);
#23442=ORIENTED_EDGE('',*,*,#17623,.F.);
#23443=ORIENTED_EDGE('',*,*,#17624,.F.);
#23444=ORIENTED_EDGE('',*,*,#17625,.T.);
#23445=ORIENTED_EDGE('',*,*,#17626,.T.);
#23446=ORIENTED_EDGE('',*,*,#17621,.F.);
#23447=ORIENTED_EDGE('',*,*,#17627,.F.);
#23448=ORIENTED_EDGE('',*,*,#17628,.T.);
#23449=ORIENTED_EDGE('',*,*,#17629,.T.);
#23450=ORIENTED_EDGE('',*,*,#17625,.F.);
#23451=ORIENTED_EDGE('',*,*,#17630,.F.);
#23452=ORIENTED_EDGE('',*,*,#17631,.T.);
#23453=ORIENTED_EDGE('',*,*,#17632,.T.);
#23454=ORIENTED_EDGE('',*,*,#17628,.F.);
#23455=ORIENTED_EDGE('',*,*,#17633,.F.);
#23456=ORIENTED_EDGE('',*,*,#17634,.T.);
#23457=ORIENTED_EDGE('',*,*,#17635,.T.);
#23458=ORIENTED_EDGE('',*,*,#17631,.F.);
#23459=ORIENTED_EDGE('',*,*,#17636,.F.);
#23460=ORIENTED_EDGE('',*,*,#17637,.T.);
#23461=ORIENTED_EDGE('',*,*,#17638,.T.);
#23462=ORIENTED_EDGE('',*,*,#17634,.F.);
#23463=ORIENTED_EDGE('',*,*,#17639,.F.);
#23464=ORIENTED_EDGE('',*,*,#17640,.T.);
#23465=ORIENTED_EDGE('',*,*,#17641,.T.);
#23466=ORIENTED_EDGE('',*,*,#17637,.F.);
#23467=ORIENTED_EDGE('',*,*,#17642,.F.);
#23468=ORIENTED_EDGE('',*,*,#17623,.T.);
#23469=ORIENTED_EDGE('',*,*,#17643,.T.);
#23470=ORIENTED_EDGE('',*,*,#17640,.F.);
#23471=ORIENTED_EDGE('',*,*,#17644,.F.);
#23472=ORIENTED_EDGE('',*,*,#17645,.T.);
#23473=ORIENTED_EDGE('',*,*,#17646,.T.);
#23474=ORIENTED_EDGE('',*,*,#17647,.F.);
#23475=ORIENTED_EDGE('',*,*,#17648,.F.);
#23476=ORIENTED_EDGE('',*,*,#17649,.T.);
#23477=ORIENTED_EDGE('',*,*,#17650,.T.);
#23478=ORIENTED_EDGE('',*,*,#17645,.F.);
#23479=ORIENTED_EDGE('',*,*,#17651,.F.);
#23480=ORIENTED_EDGE('',*,*,#17652,.T.);
#23481=ORIENTED_EDGE('',*,*,#17653,.T.);
#23482=ORIENTED_EDGE('',*,*,#17649,.F.);
#23483=ORIENTED_EDGE('',*,*,#17654,.F.);
#23484=ORIENTED_EDGE('',*,*,#17655,.T.);
#23485=ORIENTED_EDGE('',*,*,#17656,.T.);
#23486=ORIENTED_EDGE('',*,*,#17652,.F.);
#23487=ORIENTED_EDGE('',*,*,#17657,.F.);
#23488=ORIENTED_EDGE('',*,*,#17658,.T.);
#23489=ORIENTED_EDGE('',*,*,#17659,.T.);
#23490=ORIENTED_EDGE('',*,*,#17655,.F.);
#23491=ORIENTED_EDGE('',*,*,#17660,.F.);
#23492=ORIENTED_EDGE('',*,*,#17661,.T.);
#23493=ORIENTED_EDGE('',*,*,#17662,.T.);
#23494=ORIENTED_EDGE('',*,*,#17658,.F.);
#23495=ORIENTED_EDGE('',*,*,#17663,.F.);
#23496=ORIENTED_EDGE('',*,*,#17664,.T.);
#23497=ORIENTED_EDGE('',*,*,#17665,.T.);
#23498=ORIENTED_EDGE('',*,*,#17661,.F.);
#23499=ORIENTED_EDGE('',*,*,#17666,.F.);
#23500=ORIENTED_EDGE('',*,*,#17667,.T.);
#23501=ORIENTED_EDGE('',*,*,#17668,.T.);
#23502=ORIENTED_EDGE('',*,*,#17664,.F.);
#23503=ORIENTED_EDGE('',*,*,#17669,.F.);
#23504=ORIENTED_EDGE('',*,*,#17670,.T.);
#23505=ORIENTED_EDGE('',*,*,#17671,.T.);
#23506=ORIENTED_EDGE('',*,*,#17667,.F.);
#23507=ORIENTED_EDGE('',*,*,#17672,.F.);
#23508=ORIENTED_EDGE('',*,*,#17673,.T.);
#23509=ORIENTED_EDGE('',*,*,#17674,.T.);
#23510=ORIENTED_EDGE('',*,*,#17670,.F.);
#23511=ORIENTED_EDGE('',*,*,#17675,.F.);
#23512=ORIENTED_EDGE('',*,*,#17676,.T.);
#23513=ORIENTED_EDGE('',*,*,#17677,.T.);
#23514=ORIENTED_EDGE('',*,*,#17673,.F.);
#23515=ORIENTED_EDGE('',*,*,#17678,.F.);
#23516=ORIENTED_EDGE('',*,*,#17647,.T.);
#23517=ORIENTED_EDGE('',*,*,#17679,.T.);
#23518=ORIENTED_EDGE('',*,*,#17676,.F.);
#23519=ORIENTED_EDGE('',*,*,#17679,.F.);
#23520=ORIENTED_EDGE('',*,*,#17646,.F.);
#23521=ORIENTED_EDGE('',*,*,#17650,.F.);
#23522=ORIENTED_EDGE('',*,*,#17653,.F.);
#23523=ORIENTED_EDGE('',*,*,#17656,.F.);
#23524=ORIENTED_EDGE('',*,*,#17659,.F.);
#23525=ORIENTED_EDGE('',*,*,#17662,.F.);
#23526=ORIENTED_EDGE('',*,*,#17665,.F.);
#23527=ORIENTED_EDGE('',*,*,#17668,.F.);
#23528=ORIENTED_EDGE('',*,*,#17671,.F.);
#23529=ORIENTED_EDGE('',*,*,#17674,.F.);
#23530=ORIENTED_EDGE('',*,*,#17677,.F.);
#23531=ORIENTED_EDGE('',*,*,#17643,.F.);
#23532=ORIENTED_EDGE('',*,*,#17622,.F.);
#23533=ORIENTED_EDGE('',*,*,#17626,.F.);
#23534=ORIENTED_EDGE('',*,*,#17629,.F.);
#23535=ORIENTED_EDGE('',*,*,#17632,.F.);
#23536=ORIENTED_EDGE('',*,*,#17635,.F.);
#23537=ORIENTED_EDGE('',*,*,#17638,.F.);
#23538=ORIENTED_EDGE('',*,*,#17641,.F.);
#23539=ORIENTED_EDGE('',*,*,#17680,.F.);
#23540=ORIENTED_EDGE('',*,*,#17681,.T.);
#23541=ORIENTED_EDGE('',*,*,#17682,.T.);
#23542=ORIENTED_EDGE('',*,*,#17683,.F.);
#23543=ORIENTED_EDGE('',*,*,#17684,.F.);
#23544=ORIENTED_EDGE('',*,*,#17685,.T.);
#23545=ORIENTED_EDGE('',*,*,#17686,.T.);
#23546=ORIENTED_EDGE('',*,*,#17681,.F.);
#23547=ORIENTED_EDGE('',*,*,#17687,.F.);
#23548=ORIENTED_EDGE('',*,*,#17688,.T.);
#23549=ORIENTED_EDGE('',*,*,#17689,.T.);
#23550=ORIENTED_EDGE('',*,*,#17685,.F.);
#23551=ORIENTED_EDGE('',*,*,#17690,.F.);
#23552=ORIENTED_EDGE('',*,*,#17691,.T.);
#23553=ORIENTED_EDGE('',*,*,#17692,.T.);
#23554=ORIENTED_EDGE('',*,*,#17688,.F.);
#23555=ORIENTED_EDGE('',*,*,#17693,.F.);
#23556=ORIENTED_EDGE('',*,*,#17694,.T.);
#23557=ORIENTED_EDGE('',*,*,#17695,.T.);
#23558=ORIENTED_EDGE('',*,*,#17691,.F.);
#23559=ORIENTED_EDGE('',*,*,#17696,.F.);
#23560=ORIENTED_EDGE('',*,*,#17697,.T.);
#23561=ORIENTED_EDGE('',*,*,#17698,.T.);
#23562=ORIENTED_EDGE('',*,*,#17694,.F.);
#23563=ORIENTED_EDGE('',*,*,#17699,.F.);
#23564=ORIENTED_EDGE('',*,*,#17700,.T.);
#23565=ORIENTED_EDGE('',*,*,#17701,.T.);
#23566=ORIENTED_EDGE('',*,*,#17697,.F.);
#23567=ORIENTED_EDGE('',*,*,#17702,.F.);
#23568=ORIENTED_EDGE('',*,*,#17703,.T.);
#23569=ORIENTED_EDGE('',*,*,#17704,.T.);
#23570=ORIENTED_EDGE('',*,*,#17700,.F.);
#23571=ORIENTED_EDGE('',*,*,#17705,.F.);
#23572=ORIENTED_EDGE('',*,*,#17683,.T.);
#23573=ORIENTED_EDGE('',*,*,#17706,.T.);
#23574=ORIENTED_EDGE('',*,*,#17703,.F.);
#23575=ORIENTED_EDGE('',*,*,#17706,.F.);
#23576=ORIENTED_EDGE('',*,*,#17682,.F.);
#23577=ORIENTED_EDGE('',*,*,#17686,.F.);
#23578=ORIENTED_EDGE('',*,*,#17689,.F.);
#23579=ORIENTED_EDGE('',*,*,#17692,.F.);
#23580=ORIENTED_EDGE('',*,*,#17695,.F.);
#23581=ORIENTED_EDGE('',*,*,#17698,.F.);
#23582=ORIENTED_EDGE('',*,*,#17701,.F.);
#23583=ORIENTED_EDGE('',*,*,#17704,.F.);
#23584=ORIENTED_EDGE('',*,*,#17620,.T.);
#23585=ORIENTED_EDGE('',*,*,#17642,.T.);
#23586=ORIENTED_EDGE('',*,*,#17639,.T.);
#23587=ORIENTED_EDGE('',*,*,#17636,.T.);
#23588=ORIENTED_EDGE('',*,*,#17633,.T.);
#23589=ORIENTED_EDGE('',*,*,#17630,.T.);
#23590=ORIENTED_EDGE('',*,*,#17627,.T.);
#23591=ORIENTED_EDGE('',*,*,#17624,.T.);
#23592=ORIENTED_EDGE('',*,*,#17707,.F.);
#23593=ORIENTED_EDGE('',*,*,#17708,.T.);
#23594=ORIENTED_EDGE('',*,*,#17709,.T.);
#23595=ORIENTED_EDGE('',*,*,#17710,.F.);
#23596=ORIENTED_EDGE('',*,*,#17711,.F.);
#23597=ORIENTED_EDGE('',*,*,#17712,.T.);
#23598=ORIENTED_EDGE('',*,*,#17713,.T.);
#23599=ORIENTED_EDGE('',*,*,#17708,.F.);
#23600=ORIENTED_EDGE('',*,*,#17714,.F.);
#23601=ORIENTED_EDGE('',*,*,#17715,.T.);
#23602=ORIENTED_EDGE('',*,*,#17716,.T.);
#23603=ORIENTED_EDGE('',*,*,#17712,.F.);
#23604=ORIENTED_EDGE('',*,*,#17717,.F.);
#23605=ORIENTED_EDGE('',*,*,#17718,.T.);
#23606=ORIENTED_EDGE('',*,*,#17719,.T.);
#23607=ORIENTED_EDGE('',*,*,#17715,.F.);
#23608=ORIENTED_EDGE('',*,*,#17720,.F.);
#23609=ORIENTED_EDGE('',*,*,#17721,.T.);
#23610=ORIENTED_EDGE('',*,*,#17722,.T.);
#23611=ORIENTED_EDGE('',*,*,#17718,.F.);
#23612=ORIENTED_EDGE('',*,*,#17723,.F.);
#23613=ORIENTED_EDGE('',*,*,#17724,.T.);
#23614=ORIENTED_EDGE('',*,*,#17725,.T.);
#23615=ORIENTED_EDGE('',*,*,#17721,.F.);
#23616=ORIENTED_EDGE('',*,*,#17726,.F.);
#23617=ORIENTED_EDGE('',*,*,#17727,.T.);
#23618=ORIENTED_EDGE('',*,*,#17728,.T.);
#23619=ORIENTED_EDGE('',*,*,#17724,.F.);
#23620=ORIENTED_EDGE('',*,*,#17729,.F.);
#23621=ORIENTED_EDGE('',*,*,#17710,.T.);
#23622=ORIENTED_EDGE('',*,*,#17730,.T.);
#23623=ORIENTED_EDGE('',*,*,#17727,.F.);
#23624=ORIENTED_EDGE('',*,*,#17731,.F.);
#23625=ORIENTED_EDGE('',*,*,#17732,.T.);
#23626=ORIENTED_EDGE('',*,*,#17733,.T.);
#23627=ORIENTED_EDGE('',*,*,#17734,.F.);
#23628=ORIENTED_EDGE('',*,*,#17735,.F.);
#23629=ORIENTED_EDGE('',*,*,#17736,.T.);
#23630=ORIENTED_EDGE('',*,*,#17737,.T.);
#23631=ORIENTED_EDGE('',*,*,#17732,.F.);
#23632=ORIENTED_EDGE('',*,*,#17738,.F.);
#23633=ORIENTED_EDGE('',*,*,#17739,.T.);
#23634=ORIENTED_EDGE('',*,*,#17740,.T.);
#23635=ORIENTED_EDGE('',*,*,#17736,.F.);
#23636=ORIENTED_EDGE('',*,*,#17741,.F.);
#23637=ORIENTED_EDGE('',*,*,#17742,.T.);
#23638=ORIENTED_EDGE('',*,*,#17743,.T.);
#23639=ORIENTED_EDGE('',*,*,#17739,.F.);
#23640=ORIENTED_EDGE('',*,*,#17744,.F.);
#23641=ORIENTED_EDGE('',*,*,#17745,.T.);
#23642=ORIENTED_EDGE('',*,*,#17746,.T.);
#23643=ORIENTED_EDGE('',*,*,#17742,.F.);
#23644=ORIENTED_EDGE('',*,*,#17747,.F.);
#23645=ORIENTED_EDGE('',*,*,#17748,.T.);
#23646=ORIENTED_EDGE('',*,*,#17749,.T.);
#23647=ORIENTED_EDGE('',*,*,#17745,.F.);
#23648=ORIENTED_EDGE('',*,*,#17750,.F.);
#23649=ORIENTED_EDGE('',*,*,#17751,.T.);
#23650=ORIENTED_EDGE('',*,*,#17752,.T.);
#23651=ORIENTED_EDGE('',*,*,#17748,.F.);
#23652=ORIENTED_EDGE('',*,*,#17753,.F.);
#23653=ORIENTED_EDGE('',*,*,#17754,.T.);
#23654=ORIENTED_EDGE('',*,*,#17755,.T.);
#23655=ORIENTED_EDGE('',*,*,#17751,.F.);
#23656=ORIENTED_EDGE('',*,*,#17756,.F.);
#23657=ORIENTED_EDGE('',*,*,#17757,.T.);
#23658=ORIENTED_EDGE('',*,*,#17758,.T.);
#23659=ORIENTED_EDGE('',*,*,#17754,.F.);
#23660=ORIENTED_EDGE('',*,*,#17759,.F.);
#23661=ORIENTED_EDGE('',*,*,#17760,.T.);
#23662=ORIENTED_EDGE('',*,*,#17761,.T.);
#23663=ORIENTED_EDGE('',*,*,#17757,.F.);
#23664=ORIENTED_EDGE('',*,*,#17762,.F.);
#23665=ORIENTED_EDGE('',*,*,#17763,.T.);
#23666=ORIENTED_EDGE('',*,*,#17764,.T.);
#23667=ORIENTED_EDGE('',*,*,#17760,.F.);
#23668=ORIENTED_EDGE('',*,*,#17765,.F.);
#23669=ORIENTED_EDGE('',*,*,#17734,.T.);
#23670=ORIENTED_EDGE('',*,*,#17766,.T.);
#23671=ORIENTED_EDGE('',*,*,#17763,.F.);
#23672=ORIENTED_EDGE('',*,*,#17766,.F.);
#23673=ORIENTED_EDGE('',*,*,#17733,.F.);
#23674=ORIENTED_EDGE('',*,*,#17737,.F.);
#23675=ORIENTED_EDGE('',*,*,#17740,.F.);
#23676=ORIENTED_EDGE('',*,*,#17743,.F.);
#23677=ORIENTED_EDGE('',*,*,#17746,.F.);
#23678=ORIENTED_EDGE('',*,*,#17749,.F.);
#23679=ORIENTED_EDGE('',*,*,#17752,.F.);
#23680=ORIENTED_EDGE('',*,*,#17755,.F.);
#23681=ORIENTED_EDGE('',*,*,#17758,.F.);
#23682=ORIENTED_EDGE('',*,*,#17761,.F.);
#23683=ORIENTED_EDGE('',*,*,#17764,.F.);
#23684=ORIENTED_EDGE('',*,*,#17730,.F.);
#23685=ORIENTED_EDGE('',*,*,#17709,.F.);
#23686=ORIENTED_EDGE('',*,*,#17713,.F.);
#23687=ORIENTED_EDGE('',*,*,#17716,.F.);
#23688=ORIENTED_EDGE('',*,*,#17719,.F.);
#23689=ORIENTED_EDGE('',*,*,#17722,.F.);
#23690=ORIENTED_EDGE('',*,*,#17725,.F.);
#23691=ORIENTED_EDGE('',*,*,#17728,.F.);
#23692=ORIENTED_EDGE('',*,*,#17707,.T.);
#23693=ORIENTED_EDGE('',*,*,#17729,.T.);
#23694=ORIENTED_EDGE('',*,*,#17726,.T.);
#23695=ORIENTED_EDGE('',*,*,#17723,.T.);
#23696=ORIENTED_EDGE('',*,*,#17720,.T.);
#23697=ORIENTED_EDGE('',*,*,#17717,.T.);
#23698=ORIENTED_EDGE('',*,*,#17714,.T.);
#23699=ORIENTED_EDGE('',*,*,#17711,.T.);
#23700=ORIENTED_EDGE('',*,*,#17767,.F.);
#23701=ORIENTED_EDGE('',*,*,#17768,.T.);
#23702=ORIENTED_EDGE('',*,*,#17769,.T.);
#23703=ORIENTED_EDGE('',*,*,#17770,.F.);
#23704=ORIENTED_EDGE('',*,*,#17771,.F.);
#23705=ORIENTED_EDGE('',*,*,#17772,.T.);
#23706=ORIENTED_EDGE('',*,*,#17773,.T.);
#23707=ORIENTED_EDGE('',*,*,#17768,.F.);
#23708=ORIENTED_EDGE('',*,*,#17774,.F.);
#23709=ORIENTED_EDGE('',*,*,#17775,.T.);
#23710=ORIENTED_EDGE('',*,*,#17776,.T.);
#23711=ORIENTED_EDGE('',*,*,#17772,.F.);
#23712=ORIENTED_EDGE('',*,*,#17777,.F.);
#23713=ORIENTED_EDGE('',*,*,#17778,.T.);
#23714=ORIENTED_EDGE('',*,*,#17779,.T.);
#23715=ORIENTED_EDGE('',*,*,#17775,.F.);
#23716=ORIENTED_EDGE('',*,*,#17780,.F.);
#23717=ORIENTED_EDGE('',*,*,#17781,.T.);
#23718=ORIENTED_EDGE('',*,*,#17782,.T.);
#23719=ORIENTED_EDGE('',*,*,#17778,.F.);
#23720=ORIENTED_EDGE('',*,*,#17783,.F.);
#23721=ORIENTED_EDGE('',*,*,#17784,.T.);
#23722=ORIENTED_EDGE('',*,*,#17785,.T.);
#23723=ORIENTED_EDGE('',*,*,#17781,.F.);
#23724=ORIENTED_EDGE('',*,*,#17786,.F.);
#23725=ORIENTED_EDGE('',*,*,#17787,.T.);
#23726=ORIENTED_EDGE('',*,*,#17788,.T.);
#23727=ORIENTED_EDGE('',*,*,#17784,.F.);
#23728=ORIENTED_EDGE('',*,*,#17789,.F.);
#23729=ORIENTED_EDGE('',*,*,#17770,.T.);
#23730=ORIENTED_EDGE('',*,*,#17790,.T.);
#23731=ORIENTED_EDGE('',*,*,#17787,.F.);
#23732=ORIENTED_EDGE('',*,*,#17791,.F.);
#23733=ORIENTED_EDGE('',*,*,#17792,.T.);
#23734=ORIENTED_EDGE('',*,*,#17793,.T.);
#23735=ORIENTED_EDGE('',*,*,#17794,.F.);
#23736=ORIENTED_EDGE('',*,*,#17795,.F.);
#23737=ORIENTED_EDGE('',*,*,#17796,.T.);
#23738=ORIENTED_EDGE('',*,*,#17797,.T.);
#23739=ORIENTED_EDGE('',*,*,#17792,.F.);
#23740=ORIENTED_EDGE('',*,*,#17798,.F.);
#23741=ORIENTED_EDGE('',*,*,#17799,.T.);
#23742=ORIENTED_EDGE('',*,*,#17800,.T.);
#23743=ORIENTED_EDGE('',*,*,#17796,.F.);
#23744=ORIENTED_EDGE('',*,*,#17801,.F.);
#23745=ORIENTED_EDGE('',*,*,#17802,.T.);
#23746=ORIENTED_EDGE('',*,*,#17803,.T.);
#23747=ORIENTED_EDGE('',*,*,#17799,.F.);
#23748=ORIENTED_EDGE('',*,*,#17804,.F.);
#23749=ORIENTED_EDGE('',*,*,#17805,.T.);
#23750=ORIENTED_EDGE('',*,*,#17806,.T.);
#23751=ORIENTED_EDGE('',*,*,#17802,.F.);
#23752=ORIENTED_EDGE('',*,*,#17807,.F.);
#23753=ORIENTED_EDGE('',*,*,#17808,.T.);
#23754=ORIENTED_EDGE('',*,*,#17809,.T.);
#23755=ORIENTED_EDGE('',*,*,#17805,.F.);
#23756=ORIENTED_EDGE('',*,*,#17810,.F.);
#23757=ORIENTED_EDGE('',*,*,#17811,.T.);
#23758=ORIENTED_EDGE('',*,*,#17812,.T.);
#23759=ORIENTED_EDGE('',*,*,#17808,.F.);
#23760=ORIENTED_EDGE('',*,*,#17813,.F.);
#23761=ORIENTED_EDGE('',*,*,#17814,.T.);
#23762=ORIENTED_EDGE('',*,*,#17815,.T.);
#23763=ORIENTED_EDGE('',*,*,#17811,.F.);
#23764=ORIENTED_EDGE('',*,*,#17816,.F.);
#23765=ORIENTED_EDGE('',*,*,#17817,.T.);
#23766=ORIENTED_EDGE('',*,*,#17818,.T.);
#23767=ORIENTED_EDGE('',*,*,#17814,.F.);
#23768=ORIENTED_EDGE('',*,*,#17819,.F.);
#23769=ORIENTED_EDGE('',*,*,#17820,.T.);
#23770=ORIENTED_EDGE('',*,*,#17821,.T.);
#23771=ORIENTED_EDGE('',*,*,#17817,.F.);
#23772=ORIENTED_EDGE('',*,*,#17822,.F.);
#23773=ORIENTED_EDGE('',*,*,#17823,.T.);
#23774=ORIENTED_EDGE('',*,*,#17824,.T.);
#23775=ORIENTED_EDGE('',*,*,#17820,.F.);
#23776=ORIENTED_EDGE('',*,*,#17825,.F.);
#23777=ORIENTED_EDGE('',*,*,#17794,.T.);
#23778=ORIENTED_EDGE('',*,*,#17826,.T.);
#23779=ORIENTED_EDGE('',*,*,#17823,.F.);
#23780=ORIENTED_EDGE('',*,*,#17826,.F.);
#23781=ORIENTED_EDGE('',*,*,#17793,.F.);
#23782=ORIENTED_EDGE('',*,*,#17797,.F.);
#23783=ORIENTED_EDGE('',*,*,#17800,.F.);
#23784=ORIENTED_EDGE('',*,*,#17803,.F.);
#23785=ORIENTED_EDGE('',*,*,#17806,.F.);
#23786=ORIENTED_EDGE('',*,*,#17809,.F.);
#23787=ORIENTED_EDGE('',*,*,#17812,.F.);
#23788=ORIENTED_EDGE('',*,*,#17815,.F.);
#23789=ORIENTED_EDGE('',*,*,#17818,.F.);
#23790=ORIENTED_EDGE('',*,*,#17821,.F.);
#23791=ORIENTED_EDGE('',*,*,#17824,.F.);
#23792=ORIENTED_EDGE('',*,*,#17790,.F.);
#23793=ORIENTED_EDGE('',*,*,#17769,.F.);
#23794=ORIENTED_EDGE('',*,*,#17773,.F.);
#23795=ORIENTED_EDGE('',*,*,#17776,.F.);
#23796=ORIENTED_EDGE('',*,*,#17779,.F.);
#23797=ORIENTED_EDGE('',*,*,#17782,.F.);
#23798=ORIENTED_EDGE('',*,*,#17785,.F.);
#23799=ORIENTED_EDGE('',*,*,#17788,.F.);
#23800=ORIENTED_EDGE('',*,*,#17827,.F.);
#23801=ORIENTED_EDGE('',*,*,#17828,.T.);
#23802=ORIENTED_EDGE('',*,*,#17829,.T.);
#23803=ORIENTED_EDGE('',*,*,#17830,.F.);
#23804=ORIENTED_EDGE('',*,*,#17831,.F.);
#23805=ORIENTED_EDGE('',*,*,#17832,.T.);
#23806=ORIENTED_EDGE('',*,*,#17833,.T.);
#23807=ORIENTED_EDGE('',*,*,#17828,.F.);
#23808=ORIENTED_EDGE('',*,*,#17834,.F.);
#23809=ORIENTED_EDGE('',*,*,#17835,.T.);
#23810=ORIENTED_EDGE('',*,*,#17836,.T.);
#23811=ORIENTED_EDGE('',*,*,#17832,.F.);
#23812=ORIENTED_EDGE('',*,*,#17837,.F.);
#23813=ORIENTED_EDGE('',*,*,#17838,.T.);
#23814=ORIENTED_EDGE('',*,*,#17839,.T.);
#23815=ORIENTED_EDGE('',*,*,#17835,.F.);
#23816=ORIENTED_EDGE('',*,*,#17840,.F.);
#23817=ORIENTED_EDGE('',*,*,#17841,.T.);
#23818=ORIENTED_EDGE('',*,*,#17842,.T.);
#23819=ORIENTED_EDGE('',*,*,#17838,.F.);
#23820=ORIENTED_EDGE('',*,*,#17843,.F.);
#23821=ORIENTED_EDGE('',*,*,#17844,.T.);
#23822=ORIENTED_EDGE('',*,*,#17845,.T.);
#23823=ORIENTED_EDGE('',*,*,#17841,.F.);
#23824=ORIENTED_EDGE('',*,*,#17846,.F.);
#23825=ORIENTED_EDGE('',*,*,#17847,.T.);
#23826=ORIENTED_EDGE('',*,*,#17848,.T.);
#23827=ORIENTED_EDGE('',*,*,#17844,.F.);
#23828=ORIENTED_EDGE('',*,*,#17849,.F.);
#23829=ORIENTED_EDGE('',*,*,#17850,.T.);
#23830=ORIENTED_EDGE('',*,*,#17851,.T.);
#23831=ORIENTED_EDGE('',*,*,#17847,.F.);
#23832=ORIENTED_EDGE('',*,*,#17852,.F.);
#23833=ORIENTED_EDGE('',*,*,#17830,.T.);
#23834=ORIENTED_EDGE('',*,*,#17853,.T.);
#23835=ORIENTED_EDGE('',*,*,#17850,.F.);
#23836=ORIENTED_EDGE('',*,*,#17853,.F.);
#23837=ORIENTED_EDGE('',*,*,#17829,.F.);
#23838=ORIENTED_EDGE('',*,*,#17833,.F.);
#23839=ORIENTED_EDGE('',*,*,#17836,.F.);
#23840=ORIENTED_EDGE('',*,*,#17839,.F.);
#23841=ORIENTED_EDGE('',*,*,#17842,.F.);
#23842=ORIENTED_EDGE('',*,*,#17845,.F.);
#23843=ORIENTED_EDGE('',*,*,#17848,.F.);
#23844=ORIENTED_EDGE('',*,*,#17851,.F.);
#23845=ORIENTED_EDGE('',*,*,#17767,.T.);
#23846=ORIENTED_EDGE('',*,*,#17789,.T.);
#23847=ORIENTED_EDGE('',*,*,#17786,.T.);
#23848=ORIENTED_EDGE('',*,*,#17783,.T.);
#23849=ORIENTED_EDGE('',*,*,#17780,.T.);
#23850=ORIENTED_EDGE('',*,*,#17777,.T.);
#23851=ORIENTED_EDGE('',*,*,#17774,.T.);
#23852=ORIENTED_EDGE('',*,*,#17771,.T.);
#23853=ORIENTED_EDGE('',*,*,#17854,.F.);
#23854=ORIENTED_EDGE('',*,*,#17855,.T.);
#23855=ORIENTED_EDGE('',*,*,#17856,.T.);
#23856=ORIENTED_EDGE('',*,*,#17857,.F.);
#23857=ORIENTED_EDGE('',*,*,#17858,.F.);
#23858=ORIENTED_EDGE('',*,*,#17859,.T.);
#23859=ORIENTED_EDGE('',*,*,#17860,.T.);
#23860=ORIENTED_EDGE('',*,*,#17855,.F.);
#23861=ORIENTED_EDGE('',*,*,#17861,.F.);
#23862=ORIENTED_EDGE('',*,*,#17862,.T.);
#23863=ORIENTED_EDGE('',*,*,#17863,.T.);
#23864=ORIENTED_EDGE('',*,*,#17859,.F.);
#23865=ORIENTED_EDGE('',*,*,#17864,.F.);
#23866=ORIENTED_EDGE('',*,*,#17865,.T.);
#23867=ORIENTED_EDGE('',*,*,#17866,.T.);
#23868=ORIENTED_EDGE('',*,*,#17862,.F.);
#23869=ORIENTED_EDGE('',*,*,#17867,.F.);
#23870=ORIENTED_EDGE('',*,*,#17868,.T.);
#23871=ORIENTED_EDGE('',*,*,#17869,.T.);
#23872=ORIENTED_EDGE('',*,*,#17865,.F.);
#23873=ORIENTED_EDGE('',*,*,#17870,.F.);
#23874=ORIENTED_EDGE('',*,*,#17871,.T.);
#23875=ORIENTED_EDGE('',*,*,#17872,.T.);
#23876=ORIENTED_EDGE('',*,*,#17868,.F.);
#23877=ORIENTED_EDGE('',*,*,#17873,.F.);
#23878=ORIENTED_EDGE('',*,*,#17874,.T.);
#23879=ORIENTED_EDGE('',*,*,#17875,.T.);
#23880=ORIENTED_EDGE('',*,*,#17871,.F.);
#23881=ORIENTED_EDGE('',*,*,#17876,.F.);
#23882=ORIENTED_EDGE('',*,*,#17857,.T.);
#23883=ORIENTED_EDGE('',*,*,#17877,.T.);
#23884=ORIENTED_EDGE('',*,*,#17874,.F.);
#23885=ORIENTED_EDGE('',*,*,#17878,.F.);
#23886=ORIENTED_EDGE('',*,*,#17879,.T.);
#23887=ORIENTED_EDGE('',*,*,#17880,.T.);
#23888=ORIENTED_EDGE('',*,*,#17881,.F.);
#23889=ORIENTED_EDGE('',*,*,#17882,.F.);
#23890=ORIENTED_EDGE('',*,*,#17883,.T.);
#23891=ORIENTED_EDGE('',*,*,#17884,.T.);
#23892=ORIENTED_EDGE('',*,*,#17879,.F.);
#23893=ORIENTED_EDGE('',*,*,#17885,.F.);
#23894=ORIENTED_EDGE('',*,*,#17886,.T.);
#23895=ORIENTED_EDGE('',*,*,#17887,.T.);
#23896=ORIENTED_EDGE('',*,*,#17883,.F.);
#23897=ORIENTED_EDGE('',*,*,#17888,.F.);
#23898=ORIENTED_EDGE('',*,*,#17889,.T.);
#23899=ORIENTED_EDGE('',*,*,#17890,.T.);
#23900=ORIENTED_EDGE('',*,*,#17886,.F.);
#23901=ORIENTED_EDGE('',*,*,#17891,.F.);
#23902=ORIENTED_EDGE('',*,*,#17892,.T.);
#23903=ORIENTED_EDGE('',*,*,#17893,.T.);
#23904=ORIENTED_EDGE('',*,*,#17889,.F.);
#23905=ORIENTED_EDGE('',*,*,#17894,.F.);
#23906=ORIENTED_EDGE('',*,*,#17895,.T.);
#23907=ORIENTED_EDGE('',*,*,#17896,.T.);
#23908=ORIENTED_EDGE('',*,*,#17892,.F.);
#23909=ORIENTED_EDGE('',*,*,#17897,.F.);
#23910=ORIENTED_EDGE('',*,*,#17898,.T.);
#23911=ORIENTED_EDGE('',*,*,#17899,.T.);
#23912=ORIENTED_EDGE('',*,*,#17895,.F.);
#23913=ORIENTED_EDGE('',*,*,#17900,.F.);
#23914=ORIENTED_EDGE('',*,*,#17901,.T.);
#23915=ORIENTED_EDGE('',*,*,#17902,.T.);
#23916=ORIENTED_EDGE('',*,*,#17898,.F.);
#23917=ORIENTED_EDGE('',*,*,#17903,.F.);
#23918=ORIENTED_EDGE('',*,*,#17904,.T.);
#23919=ORIENTED_EDGE('',*,*,#17905,.T.);
#23920=ORIENTED_EDGE('',*,*,#17901,.F.);
#23921=ORIENTED_EDGE('',*,*,#17906,.F.);
#23922=ORIENTED_EDGE('',*,*,#17907,.T.);
#23923=ORIENTED_EDGE('',*,*,#17908,.T.);
#23924=ORIENTED_EDGE('',*,*,#17904,.F.);
#23925=ORIENTED_EDGE('',*,*,#17909,.F.);
#23926=ORIENTED_EDGE('',*,*,#17910,.T.);
#23927=ORIENTED_EDGE('',*,*,#17911,.T.);
#23928=ORIENTED_EDGE('',*,*,#17907,.F.);
#23929=ORIENTED_EDGE('',*,*,#17912,.F.);
#23930=ORIENTED_EDGE('',*,*,#17881,.T.);
#23931=ORIENTED_EDGE('',*,*,#17913,.T.);
#23932=ORIENTED_EDGE('',*,*,#17910,.F.);
#23933=ORIENTED_EDGE('',*,*,#17913,.F.);
#23934=ORIENTED_EDGE('',*,*,#17880,.F.);
#23935=ORIENTED_EDGE('',*,*,#17884,.F.);
#23936=ORIENTED_EDGE('',*,*,#17887,.F.);
#23937=ORIENTED_EDGE('',*,*,#17890,.F.);
#23938=ORIENTED_EDGE('',*,*,#17893,.F.);
#23939=ORIENTED_EDGE('',*,*,#17896,.F.);
#23940=ORIENTED_EDGE('',*,*,#17899,.F.);
#23941=ORIENTED_EDGE('',*,*,#17902,.F.);
#23942=ORIENTED_EDGE('',*,*,#17905,.F.);
#23943=ORIENTED_EDGE('',*,*,#17908,.F.);
#23944=ORIENTED_EDGE('',*,*,#17911,.F.);
#23945=ORIENTED_EDGE('',*,*,#17877,.F.);
#23946=ORIENTED_EDGE('',*,*,#17856,.F.);
#23947=ORIENTED_EDGE('',*,*,#17860,.F.);
#23948=ORIENTED_EDGE('',*,*,#17863,.F.);
#23949=ORIENTED_EDGE('',*,*,#17866,.F.);
#23950=ORIENTED_EDGE('',*,*,#17869,.F.);
#23951=ORIENTED_EDGE('',*,*,#17872,.F.);
#23952=ORIENTED_EDGE('',*,*,#17875,.F.);
#23953=ORIENTED_EDGE('',*,*,#17914,.F.);
#23954=ORIENTED_EDGE('',*,*,#17915,.T.);
#23955=ORIENTED_EDGE('',*,*,#17916,.T.);
#23956=ORIENTED_EDGE('',*,*,#17917,.F.);
#23957=ORIENTED_EDGE('',*,*,#17918,.F.);
#23958=ORIENTED_EDGE('',*,*,#17919,.T.);
#23959=ORIENTED_EDGE('',*,*,#17920,.T.);
#23960=ORIENTED_EDGE('',*,*,#17915,.F.);
#23961=ORIENTED_EDGE('',*,*,#17921,.F.);
#23962=ORIENTED_EDGE('',*,*,#17922,.T.);
#23963=ORIENTED_EDGE('',*,*,#17923,.T.);
#23964=ORIENTED_EDGE('',*,*,#17919,.F.);
#23965=ORIENTED_EDGE('',*,*,#17924,.F.);
#23966=ORIENTED_EDGE('',*,*,#17925,.T.);
#23967=ORIENTED_EDGE('',*,*,#17926,.T.);
#23968=ORIENTED_EDGE('',*,*,#17922,.F.);
#23969=ORIENTED_EDGE('',*,*,#17927,.F.);
#23970=ORIENTED_EDGE('',*,*,#17928,.T.);
#23971=ORIENTED_EDGE('',*,*,#17929,.T.);
#23972=ORIENTED_EDGE('',*,*,#17925,.F.);
#23973=ORIENTED_EDGE('',*,*,#17930,.F.);
#23974=ORIENTED_EDGE('',*,*,#17931,.T.);
#23975=ORIENTED_EDGE('',*,*,#17932,.T.);
#23976=ORIENTED_EDGE('',*,*,#17928,.F.);
#23977=ORIENTED_EDGE('',*,*,#17933,.F.);
#23978=ORIENTED_EDGE('',*,*,#17934,.T.);
#23979=ORIENTED_EDGE('',*,*,#17935,.T.);
#23980=ORIENTED_EDGE('',*,*,#17931,.F.);
#23981=ORIENTED_EDGE('',*,*,#17936,.F.);
#23982=ORIENTED_EDGE('',*,*,#17937,.T.);
#23983=ORIENTED_EDGE('',*,*,#17938,.T.);
#23984=ORIENTED_EDGE('',*,*,#17934,.F.);
#23985=ORIENTED_EDGE('',*,*,#17939,.F.);
#23986=ORIENTED_EDGE('',*,*,#17940,.T.);
#23987=ORIENTED_EDGE('',*,*,#17941,.T.);
#23988=ORIENTED_EDGE('',*,*,#17937,.F.);
#23989=ORIENTED_EDGE('',*,*,#17942,.F.);
#23990=ORIENTED_EDGE('',*,*,#17943,.T.);
#23991=ORIENTED_EDGE('',*,*,#17944,.T.);
#23992=ORIENTED_EDGE('',*,*,#17940,.F.);
#23993=ORIENTED_EDGE('',*,*,#17945,.F.);
#23994=ORIENTED_EDGE('',*,*,#17946,.T.);
#23995=ORIENTED_EDGE('',*,*,#17947,.T.);
#23996=ORIENTED_EDGE('',*,*,#17943,.F.);
#23997=ORIENTED_EDGE('',*,*,#17948,.F.);
#23998=ORIENTED_EDGE('',*,*,#17949,.T.);
#23999=ORIENTED_EDGE('',*,*,#17950,.T.);
#24000=ORIENTED_EDGE('',*,*,#17946,.F.);
#24001=ORIENTED_EDGE('',*,*,#17951,.F.);
#24002=ORIENTED_EDGE('',*,*,#17952,.T.);
#24003=ORIENTED_EDGE('',*,*,#17953,.T.);
#24004=ORIENTED_EDGE('',*,*,#17949,.F.);
#24005=ORIENTED_EDGE('',*,*,#17954,.F.);
#24006=ORIENTED_EDGE('',*,*,#17955,.T.);
#24007=ORIENTED_EDGE('',*,*,#17956,.T.);
#24008=ORIENTED_EDGE('',*,*,#17952,.F.);
#24009=ORIENTED_EDGE('',*,*,#17957,.F.);
#24010=ORIENTED_EDGE('',*,*,#17958,.T.);
#24011=ORIENTED_EDGE('',*,*,#17959,.T.);
#24012=ORIENTED_EDGE('',*,*,#17955,.F.);
#24013=ORIENTED_EDGE('',*,*,#17960,.F.);
#24014=ORIENTED_EDGE('',*,*,#17961,.T.);
#24015=ORIENTED_EDGE('',*,*,#17962,.T.);
#24016=ORIENTED_EDGE('',*,*,#17958,.F.);
#24017=ORIENTED_EDGE('',*,*,#17963,.F.);
#24018=ORIENTED_EDGE('',*,*,#17964,.T.);
#24019=ORIENTED_EDGE('',*,*,#17965,.T.);
#24020=ORIENTED_EDGE('',*,*,#17961,.F.);
#24021=ORIENTED_EDGE('',*,*,#17966,.F.);
#24022=ORIENTED_EDGE('',*,*,#17967,.T.);
#24023=ORIENTED_EDGE('',*,*,#17968,.T.);
#24024=ORIENTED_EDGE('',*,*,#17964,.F.);
#24025=ORIENTED_EDGE('',*,*,#17969,.F.);
#24026=ORIENTED_EDGE('',*,*,#17970,.T.);
#24027=ORIENTED_EDGE('',*,*,#17971,.T.);
#24028=ORIENTED_EDGE('',*,*,#17967,.F.);
#24029=ORIENTED_EDGE('',*,*,#17972,.F.);
#24030=ORIENTED_EDGE('',*,*,#17973,.T.);
#24031=ORIENTED_EDGE('',*,*,#17974,.T.);
#24032=ORIENTED_EDGE('',*,*,#17970,.F.);
#24033=ORIENTED_EDGE('',*,*,#17975,.F.);
#24034=ORIENTED_EDGE('',*,*,#17976,.T.);
#24035=ORIENTED_EDGE('',*,*,#17977,.T.);
#24036=ORIENTED_EDGE('',*,*,#17973,.F.);
#24037=ORIENTED_EDGE('',*,*,#17978,.F.);
#24038=ORIENTED_EDGE('',*,*,#17917,.T.);
#24039=ORIENTED_EDGE('',*,*,#17979,.T.);
#24040=ORIENTED_EDGE('',*,*,#17976,.F.);
#24041=ORIENTED_EDGE('',*,*,#17979,.F.);
#24042=ORIENTED_EDGE('',*,*,#17916,.F.);
#24043=ORIENTED_EDGE('',*,*,#17920,.F.);
#24044=ORIENTED_EDGE('',*,*,#17923,.F.);
#24045=ORIENTED_EDGE('',*,*,#17926,.F.);
#24046=ORIENTED_EDGE('',*,*,#17929,.F.);
#24047=ORIENTED_EDGE('',*,*,#17932,.F.);
#24048=ORIENTED_EDGE('',*,*,#17935,.F.);
#24049=ORIENTED_EDGE('',*,*,#17938,.F.);
#24050=ORIENTED_EDGE('',*,*,#17941,.F.);
#24051=ORIENTED_EDGE('',*,*,#17944,.F.);
#24052=ORIENTED_EDGE('',*,*,#17947,.F.);
#24053=ORIENTED_EDGE('',*,*,#17950,.F.);
#24054=ORIENTED_EDGE('',*,*,#17953,.F.);
#24055=ORIENTED_EDGE('',*,*,#17956,.F.);
#24056=ORIENTED_EDGE('',*,*,#17959,.F.);
#24057=ORIENTED_EDGE('',*,*,#17962,.F.);
#24058=ORIENTED_EDGE('',*,*,#17965,.F.);
#24059=ORIENTED_EDGE('',*,*,#17968,.F.);
#24060=ORIENTED_EDGE('',*,*,#17971,.F.);
#24061=ORIENTED_EDGE('',*,*,#17974,.F.);
#24062=ORIENTED_EDGE('',*,*,#17977,.F.);
#24063=ORIENTED_EDGE('',*,*,#17854,.T.);
#24064=ORIENTED_EDGE('',*,*,#17876,.T.);
#24065=ORIENTED_EDGE('',*,*,#17873,.T.);
#24066=ORIENTED_EDGE('',*,*,#17870,.T.);
#24067=ORIENTED_EDGE('',*,*,#17867,.T.);
#24068=ORIENTED_EDGE('',*,*,#17864,.T.);
#24069=ORIENTED_EDGE('',*,*,#17861,.T.);
#24070=ORIENTED_EDGE('',*,*,#17858,.T.);
#24071=ORIENTED_EDGE('',*,*,#17980,.F.);
#24072=ORIENTED_EDGE('',*,*,#17981,.T.);
#24073=ORIENTED_EDGE('',*,*,#17982,.T.);
#24074=ORIENTED_EDGE('',*,*,#17983,.F.);
#24075=ORIENTED_EDGE('',*,*,#17984,.F.);
#24076=ORIENTED_EDGE('',*,*,#17985,.T.);
#24077=ORIENTED_EDGE('',*,*,#17986,.T.);
#24078=ORIENTED_EDGE('',*,*,#17981,.F.);
#24079=ORIENTED_EDGE('',*,*,#17987,.F.);
#24080=ORIENTED_EDGE('',*,*,#17988,.T.);
#24081=ORIENTED_EDGE('',*,*,#17989,.T.);
#24082=ORIENTED_EDGE('',*,*,#17985,.F.);
#24083=ORIENTED_EDGE('',*,*,#17990,.F.);
#24084=ORIENTED_EDGE('',*,*,#17991,.T.);
#24085=ORIENTED_EDGE('',*,*,#17992,.T.);
#24086=ORIENTED_EDGE('',*,*,#17988,.F.);
#24087=ORIENTED_EDGE('',*,*,#17993,.F.);
#24088=ORIENTED_EDGE('',*,*,#17994,.T.);
#24089=ORIENTED_EDGE('',*,*,#17995,.T.);
#24090=ORIENTED_EDGE('',*,*,#17991,.F.);
#24091=ORIENTED_EDGE('',*,*,#17996,.F.);
#24092=ORIENTED_EDGE('',*,*,#17997,.T.);
#24093=ORIENTED_EDGE('',*,*,#17998,.T.);
#24094=ORIENTED_EDGE('',*,*,#17994,.F.);
#24095=ORIENTED_EDGE('',*,*,#17999,.F.);
#24096=ORIENTED_EDGE('',*,*,#18000,.T.);
#24097=ORIENTED_EDGE('',*,*,#18001,.T.);
#24098=ORIENTED_EDGE('',*,*,#17997,.F.);
#24099=ORIENTED_EDGE('',*,*,#18002,.F.);
#24100=ORIENTED_EDGE('',*,*,#17983,.T.);
#24101=ORIENTED_EDGE('',*,*,#18003,.T.);
#24102=ORIENTED_EDGE('',*,*,#18000,.F.);
#24103=ORIENTED_EDGE('',*,*,#18004,.F.);
#24104=ORIENTED_EDGE('',*,*,#18005,.T.);
#24105=ORIENTED_EDGE('',*,*,#18006,.T.);
#24106=ORIENTED_EDGE('',*,*,#18007,.F.);
#24107=ORIENTED_EDGE('',*,*,#18008,.F.);
#24108=ORIENTED_EDGE('',*,*,#18009,.T.);
#24109=ORIENTED_EDGE('',*,*,#18010,.T.);
#24110=ORIENTED_EDGE('',*,*,#18005,.F.);
#24111=ORIENTED_EDGE('',*,*,#18011,.F.);
#24112=ORIENTED_EDGE('',*,*,#18012,.T.);
#24113=ORIENTED_EDGE('',*,*,#18013,.T.);
#24114=ORIENTED_EDGE('',*,*,#18009,.F.);
#24115=ORIENTED_EDGE('',*,*,#18014,.F.);
#24116=ORIENTED_EDGE('',*,*,#18015,.T.);
#24117=ORIENTED_EDGE('',*,*,#18016,.T.);
#24118=ORIENTED_EDGE('',*,*,#18012,.F.);
#24119=ORIENTED_EDGE('',*,*,#18017,.F.);
#24120=ORIENTED_EDGE('',*,*,#18018,.T.);
#24121=ORIENTED_EDGE('',*,*,#18019,.T.);
#24122=ORIENTED_EDGE('',*,*,#18015,.F.);
#24123=ORIENTED_EDGE('',*,*,#18020,.F.);
#24124=ORIENTED_EDGE('',*,*,#18021,.T.);
#24125=ORIENTED_EDGE('',*,*,#18022,.T.);
#24126=ORIENTED_EDGE('',*,*,#18018,.F.);
#24127=ORIENTED_EDGE('',*,*,#18023,.F.);
#24128=ORIENTED_EDGE('',*,*,#18024,.T.);
#24129=ORIENTED_EDGE('',*,*,#18025,.T.);
#24130=ORIENTED_EDGE('',*,*,#18021,.F.);
#24131=ORIENTED_EDGE('',*,*,#18026,.F.);
#24132=ORIENTED_EDGE('',*,*,#18027,.T.);
#24133=ORIENTED_EDGE('',*,*,#18028,.T.);
#24134=ORIENTED_EDGE('',*,*,#18024,.F.);
#24135=ORIENTED_EDGE('',*,*,#18029,.F.);
#24136=ORIENTED_EDGE('',*,*,#18030,.T.);
#24137=ORIENTED_EDGE('',*,*,#18031,.T.);
#24138=ORIENTED_EDGE('',*,*,#18027,.F.);
#24139=ORIENTED_EDGE('',*,*,#18032,.F.);
#24140=ORIENTED_EDGE('',*,*,#18033,.T.);
#24141=ORIENTED_EDGE('',*,*,#18034,.T.);
#24142=ORIENTED_EDGE('',*,*,#18030,.F.);
#24143=ORIENTED_EDGE('',*,*,#18035,.F.);
#24144=ORIENTED_EDGE('',*,*,#18036,.T.);
#24145=ORIENTED_EDGE('',*,*,#18037,.T.);
#24146=ORIENTED_EDGE('',*,*,#18033,.F.);
#24147=ORIENTED_EDGE('',*,*,#18038,.F.);
#24148=ORIENTED_EDGE('',*,*,#18007,.T.);
#24149=ORIENTED_EDGE('',*,*,#18039,.T.);
#24150=ORIENTED_EDGE('',*,*,#18036,.F.);
#24151=ORIENTED_EDGE('',*,*,#18039,.F.);
#24152=ORIENTED_EDGE('',*,*,#18006,.F.);
#24153=ORIENTED_EDGE('',*,*,#18010,.F.);
#24154=ORIENTED_EDGE('',*,*,#18013,.F.);
#24155=ORIENTED_EDGE('',*,*,#18016,.F.);
#24156=ORIENTED_EDGE('',*,*,#18019,.F.);
#24157=ORIENTED_EDGE('',*,*,#18022,.F.);
#24158=ORIENTED_EDGE('',*,*,#18025,.F.);
#24159=ORIENTED_EDGE('',*,*,#18028,.F.);
#24160=ORIENTED_EDGE('',*,*,#18031,.F.);
#24161=ORIENTED_EDGE('',*,*,#18034,.F.);
#24162=ORIENTED_EDGE('',*,*,#18037,.F.);
#24163=ORIENTED_EDGE('',*,*,#18003,.F.);
#24164=ORIENTED_EDGE('',*,*,#17982,.F.);
#24165=ORIENTED_EDGE('',*,*,#17986,.F.);
#24166=ORIENTED_EDGE('',*,*,#17989,.F.);
#24167=ORIENTED_EDGE('',*,*,#17992,.F.);
#24168=ORIENTED_EDGE('',*,*,#17995,.F.);
#24169=ORIENTED_EDGE('',*,*,#17998,.F.);
#24170=ORIENTED_EDGE('',*,*,#18001,.F.);
#24171=ORIENTED_EDGE('',*,*,#18040,.F.);
#24172=ORIENTED_EDGE('',*,*,#18041,.T.);
#24173=ORIENTED_EDGE('',*,*,#18042,.T.);
#24174=ORIENTED_EDGE('',*,*,#18043,.F.);
#24175=ORIENTED_EDGE('',*,*,#18044,.F.);
#24176=ORIENTED_EDGE('',*,*,#18045,.T.);
#24177=ORIENTED_EDGE('',*,*,#18046,.T.);
#24178=ORIENTED_EDGE('',*,*,#18041,.F.);
#24179=ORIENTED_EDGE('',*,*,#18047,.F.);
#24180=ORIENTED_EDGE('',*,*,#18048,.T.);
#24181=ORIENTED_EDGE('',*,*,#18049,.T.);
#24182=ORIENTED_EDGE('',*,*,#18045,.F.);
#24183=ORIENTED_EDGE('',*,*,#18050,.F.);
#24184=ORIENTED_EDGE('',*,*,#18051,.T.);
#24185=ORIENTED_EDGE('',*,*,#18052,.T.);
#24186=ORIENTED_EDGE('',*,*,#18048,.F.);
#24187=ORIENTED_EDGE('',*,*,#18053,.F.);
#24188=ORIENTED_EDGE('',*,*,#18054,.T.);
#24189=ORIENTED_EDGE('',*,*,#18055,.T.);
#24190=ORIENTED_EDGE('',*,*,#18051,.F.);
#24191=ORIENTED_EDGE('',*,*,#18056,.F.);
#24192=ORIENTED_EDGE('',*,*,#18057,.T.);
#24193=ORIENTED_EDGE('',*,*,#18058,.T.);
#24194=ORIENTED_EDGE('',*,*,#18054,.F.);
#24195=ORIENTED_EDGE('',*,*,#18059,.F.);
#24196=ORIENTED_EDGE('',*,*,#18060,.T.);
#24197=ORIENTED_EDGE('',*,*,#18061,.T.);
#24198=ORIENTED_EDGE('',*,*,#18057,.F.);
#24199=ORIENTED_EDGE('',*,*,#18062,.F.);
#24200=ORIENTED_EDGE('',*,*,#18063,.T.);
#24201=ORIENTED_EDGE('',*,*,#18064,.T.);
#24202=ORIENTED_EDGE('',*,*,#18060,.F.);
#24203=ORIENTED_EDGE('',*,*,#18065,.F.);
#24204=ORIENTED_EDGE('',*,*,#18066,.T.);
#24205=ORIENTED_EDGE('',*,*,#18067,.T.);
#24206=ORIENTED_EDGE('',*,*,#18063,.F.);
#24207=ORIENTED_EDGE('',*,*,#18068,.F.);
#24208=ORIENTED_EDGE('',*,*,#18069,.T.);
#24209=ORIENTED_EDGE('',*,*,#18070,.T.);
#24210=ORIENTED_EDGE('',*,*,#18066,.F.);
#24211=ORIENTED_EDGE('',*,*,#18071,.F.);
#24212=ORIENTED_EDGE('',*,*,#18072,.T.);
#24213=ORIENTED_EDGE('',*,*,#18073,.T.);
#24214=ORIENTED_EDGE('',*,*,#18069,.F.);
#24215=ORIENTED_EDGE('',*,*,#18074,.F.);
#24216=ORIENTED_EDGE('',*,*,#18075,.T.);
#24217=ORIENTED_EDGE('',*,*,#18076,.T.);
#24218=ORIENTED_EDGE('',*,*,#18072,.F.);
#24219=ORIENTED_EDGE('',*,*,#18077,.F.);
#24220=ORIENTED_EDGE('',*,*,#18078,.T.);
#24221=ORIENTED_EDGE('',*,*,#18079,.T.);
#24222=ORIENTED_EDGE('',*,*,#18075,.F.);
#24223=ORIENTED_EDGE('',*,*,#18080,.F.);
#24224=ORIENTED_EDGE('',*,*,#18081,.T.);
#24225=ORIENTED_EDGE('',*,*,#18082,.T.);
#24226=ORIENTED_EDGE('',*,*,#18078,.F.);
#24227=ORIENTED_EDGE('',*,*,#18083,.F.);
#24228=ORIENTED_EDGE('',*,*,#18084,.T.);
#24229=ORIENTED_EDGE('',*,*,#18085,.T.);
#24230=ORIENTED_EDGE('',*,*,#18081,.F.);
#24231=ORIENTED_EDGE('',*,*,#18086,.F.);
#24232=ORIENTED_EDGE('',*,*,#18087,.T.);
#24233=ORIENTED_EDGE('',*,*,#18088,.T.);
#24234=ORIENTED_EDGE('',*,*,#18084,.F.);
#24235=ORIENTED_EDGE('',*,*,#18089,.F.);
#24236=ORIENTED_EDGE('',*,*,#18090,.T.);
#24237=ORIENTED_EDGE('',*,*,#18091,.T.);
#24238=ORIENTED_EDGE('',*,*,#18087,.F.);
#24239=ORIENTED_EDGE('',*,*,#18092,.F.);
#24240=ORIENTED_EDGE('',*,*,#18093,.T.);
#24241=ORIENTED_EDGE('',*,*,#18094,.T.);
#24242=ORIENTED_EDGE('',*,*,#18090,.F.);
#24243=ORIENTED_EDGE('',*,*,#18095,.F.);
#24244=ORIENTED_EDGE('',*,*,#18096,.T.);
#24245=ORIENTED_EDGE('',*,*,#18097,.T.);
#24246=ORIENTED_EDGE('',*,*,#18093,.F.);
#24247=ORIENTED_EDGE('',*,*,#18098,.F.);
#24248=ORIENTED_EDGE('',*,*,#18099,.T.);
#24249=ORIENTED_EDGE('',*,*,#18100,.T.);
#24250=ORIENTED_EDGE('',*,*,#18096,.F.);
#24251=ORIENTED_EDGE('',*,*,#18101,.F.);
#24252=ORIENTED_EDGE('',*,*,#18102,.T.);
#24253=ORIENTED_EDGE('',*,*,#18103,.T.);
#24254=ORIENTED_EDGE('',*,*,#18099,.F.);
#24255=ORIENTED_EDGE('',*,*,#18104,.F.);
#24256=ORIENTED_EDGE('',*,*,#18105,.T.);
#24257=ORIENTED_EDGE('',*,*,#18106,.T.);
#24258=ORIENTED_EDGE('',*,*,#18102,.F.);
#24259=ORIENTED_EDGE('',*,*,#18107,.F.);
#24260=ORIENTED_EDGE('',*,*,#18108,.T.);
#24261=ORIENTED_EDGE('',*,*,#18109,.T.);
#24262=ORIENTED_EDGE('',*,*,#18105,.F.);
#24263=ORIENTED_EDGE('',*,*,#18110,.F.);
#24264=ORIENTED_EDGE('',*,*,#18111,.T.);
#24265=ORIENTED_EDGE('',*,*,#18112,.T.);
#24266=ORIENTED_EDGE('',*,*,#18108,.F.);
#24267=ORIENTED_EDGE('',*,*,#18113,.F.);
#24268=ORIENTED_EDGE('',*,*,#18114,.T.);
#24269=ORIENTED_EDGE('',*,*,#18115,.T.);
#24270=ORIENTED_EDGE('',*,*,#18111,.F.);
#24271=ORIENTED_EDGE('',*,*,#18116,.F.);
#24272=ORIENTED_EDGE('',*,*,#18117,.T.);
#24273=ORIENTED_EDGE('',*,*,#18118,.T.);
#24274=ORIENTED_EDGE('',*,*,#18114,.F.);
#24275=ORIENTED_EDGE('',*,*,#18119,.F.);
#24276=ORIENTED_EDGE('',*,*,#18120,.T.);
#24277=ORIENTED_EDGE('',*,*,#18121,.T.);
#24278=ORIENTED_EDGE('',*,*,#18117,.F.);
#24279=ORIENTED_EDGE('',*,*,#18122,.F.);
#24280=ORIENTED_EDGE('',*,*,#18123,.T.);
#24281=ORIENTED_EDGE('',*,*,#18124,.T.);
#24282=ORIENTED_EDGE('',*,*,#18120,.F.);
#24283=ORIENTED_EDGE('',*,*,#18125,.F.);
#24284=ORIENTED_EDGE('',*,*,#18126,.T.);
#24285=ORIENTED_EDGE('',*,*,#18127,.T.);
#24286=ORIENTED_EDGE('',*,*,#18123,.F.);
#24287=ORIENTED_EDGE('',*,*,#18128,.F.);
#24288=ORIENTED_EDGE('',*,*,#18043,.T.);
#24289=ORIENTED_EDGE('',*,*,#18129,.T.);
#24290=ORIENTED_EDGE('',*,*,#18126,.F.);
#24291=ORIENTED_EDGE('',*,*,#18129,.F.);
#24292=ORIENTED_EDGE('',*,*,#18042,.F.);
#24293=ORIENTED_EDGE('',*,*,#18046,.F.);
#24294=ORIENTED_EDGE('',*,*,#18049,.F.);
#24295=ORIENTED_EDGE('',*,*,#18052,.F.);
#24296=ORIENTED_EDGE('',*,*,#18055,.F.);
#24297=ORIENTED_EDGE('',*,*,#18058,.F.);
#24298=ORIENTED_EDGE('',*,*,#18061,.F.);
#24299=ORIENTED_EDGE('',*,*,#18064,.F.);
#24300=ORIENTED_EDGE('',*,*,#18067,.F.);
#24301=ORIENTED_EDGE('',*,*,#18070,.F.);
#24302=ORIENTED_EDGE('',*,*,#18073,.F.);
#24303=ORIENTED_EDGE('',*,*,#18076,.F.);
#24304=ORIENTED_EDGE('',*,*,#18079,.F.);
#24305=ORIENTED_EDGE('',*,*,#18082,.F.);
#24306=ORIENTED_EDGE('',*,*,#18085,.F.);
#24307=ORIENTED_EDGE('',*,*,#18088,.F.);
#24308=ORIENTED_EDGE('',*,*,#18091,.F.);
#24309=ORIENTED_EDGE('',*,*,#18094,.F.);
#24310=ORIENTED_EDGE('',*,*,#18097,.F.);
#24311=ORIENTED_EDGE('',*,*,#18100,.F.);
#24312=ORIENTED_EDGE('',*,*,#18103,.F.);
#24313=ORIENTED_EDGE('',*,*,#18106,.F.);
#24314=ORIENTED_EDGE('',*,*,#18109,.F.);
#24315=ORIENTED_EDGE('',*,*,#18112,.F.);
#24316=ORIENTED_EDGE('',*,*,#18115,.F.);
#24317=ORIENTED_EDGE('',*,*,#18118,.F.);
#24318=ORIENTED_EDGE('',*,*,#18121,.F.);
#24319=ORIENTED_EDGE('',*,*,#18124,.F.);
#24320=ORIENTED_EDGE('',*,*,#18127,.F.);
#24321=ORIENTED_EDGE('',*,*,#17980,.T.);
#24322=ORIENTED_EDGE('',*,*,#18002,.T.);
#24323=ORIENTED_EDGE('',*,*,#17999,.T.);
#24324=ORIENTED_EDGE('',*,*,#17996,.T.);
#24325=ORIENTED_EDGE('',*,*,#17993,.T.);
#24326=ORIENTED_EDGE('',*,*,#17990,.T.);
#24327=ORIENTED_EDGE('',*,*,#17987,.T.);
#24328=ORIENTED_EDGE('',*,*,#17984,.T.);
#24329=ORIENTED_EDGE('',*,*,#18130,.F.);
#24330=ORIENTED_EDGE('',*,*,#18131,.T.);
#24331=ORIENTED_EDGE('',*,*,#18132,.T.);
#24332=ORIENTED_EDGE('',*,*,#18133,.F.);
#24333=ORIENTED_EDGE('',*,*,#18134,.F.);
#24334=ORIENTED_EDGE('',*,*,#18135,.T.);
#24335=ORIENTED_EDGE('',*,*,#18136,.T.);
#24336=ORIENTED_EDGE('',*,*,#18131,.F.);
#24337=ORIENTED_EDGE('',*,*,#18137,.F.);
#24338=ORIENTED_EDGE('',*,*,#18138,.T.);
#24339=ORIENTED_EDGE('',*,*,#18139,.T.);
#24340=ORIENTED_EDGE('',*,*,#18135,.F.);
#24341=ORIENTED_EDGE('',*,*,#18140,.F.);
#24342=ORIENTED_EDGE('',*,*,#18141,.T.);
#24343=ORIENTED_EDGE('',*,*,#18142,.T.);
#24344=ORIENTED_EDGE('',*,*,#18138,.F.);
#24345=ORIENTED_EDGE('',*,*,#18143,.F.);
#24346=ORIENTED_EDGE('',*,*,#18144,.T.);
#24347=ORIENTED_EDGE('',*,*,#18145,.T.);
#24348=ORIENTED_EDGE('',*,*,#18141,.F.);
#24349=ORIENTED_EDGE('',*,*,#18146,.F.);
#24350=ORIENTED_EDGE('',*,*,#18147,.T.);
#24351=ORIENTED_EDGE('',*,*,#18148,.T.);
#24352=ORIENTED_EDGE('',*,*,#18144,.F.);
#24353=ORIENTED_EDGE('',*,*,#18149,.F.);
#24354=ORIENTED_EDGE('',*,*,#18150,.T.);
#24355=ORIENTED_EDGE('',*,*,#18151,.T.);
#24356=ORIENTED_EDGE('',*,*,#18147,.F.);
#24357=ORIENTED_EDGE('',*,*,#18152,.F.);
#24358=ORIENTED_EDGE('',*,*,#18133,.T.);
#24359=ORIENTED_EDGE('',*,*,#18153,.T.);
#24360=ORIENTED_EDGE('',*,*,#18150,.F.);
#24361=ORIENTED_EDGE('',*,*,#18154,.F.);
#24362=ORIENTED_EDGE('',*,*,#18155,.T.);
#24363=ORIENTED_EDGE('',*,*,#18156,.T.);
#24364=ORIENTED_EDGE('',*,*,#18157,.F.);
#24365=ORIENTED_EDGE('',*,*,#18158,.F.);
#24366=ORIENTED_EDGE('',*,*,#18159,.T.);
#24367=ORIENTED_EDGE('',*,*,#18160,.T.);
#24368=ORIENTED_EDGE('',*,*,#18155,.F.);
#24369=ORIENTED_EDGE('',*,*,#18161,.F.);
#24370=ORIENTED_EDGE('',*,*,#18162,.T.);
#24371=ORIENTED_EDGE('',*,*,#18163,.T.);
#24372=ORIENTED_EDGE('',*,*,#18159,.F.);
#24373=ORIENTED_EDGE('',*,*,#18164,.F.);
#24374=ORIENTED_EDGE('',*,*,#18165,.T.);
#24375=ORIENTED_EDGE('',*,*,#18166,.T.);
#24376=ORIENTED_EDGE('',*,*,#18162,.F.);
#24377=ORIENTED_EDGE('',*,*,#18167,.F.);
#24378=ORIENTED_EDGE('',*,*,#18168,.T.);
#24379=ORIENTED_EDGE('',*,*,#18169,.T.);
#24380=ORIENTED_EDGE('',*,*,#18165,.F.);
#24381=ORIENTED_EDGE('',*,*,#18170,.F.);
#24382=ORIENTED_EDGE('',*,*,#18171,.T.);
#24383=ORIENTED_EDGE('',*,*,#18172,.T.);
#24384=ORIENTED_EDGE('',*,*,#18168,.F.);
#24385=ORIENTED_EDGE('',*,*,#18173,.F.);
#24386=ORIENTED_EDGE('',*,*,#18174,.T.);
#24387=ORIENTED_EDGE('',*,*,#18175,.T.);
#24388=ORIENTED_EDGE('',*,*,#18171,.F.);
#24389=ORIENTED_EDGE('',*,*,#18176,.F.);
#24390=ORIENTED_EDGE('',*,*,#18177,.T.);
#24391=ORIENTED_EDGE('',*,*,#18178,.T.);
#24392=ORIENTED_EDGE('',*,*,#18174,.F.);
#24393=ORIENTED_EDGE('',*,*,#18179,.F.);
#24394=ORIENTED_EDGE('',*,*,#18180,.T.);
#24395=ORIENTED_EDGE('',*,*,#18181,.T.);
#24396=ORIENTED_EDGE('',*,*,#18177,.F.);
#24397=ORIENTED_EDGE('',*,*,#18182,.F.);
#24398=ORIENTED_EDGE('',*,*,#18183,.T.);
#24399=ORIENTED_EDGE('',*,*,#18184,.T.);
#24400=ORIENTED_EDGE('',*,*,#18180,.F.);
#24401=ORIENTED_EDGE('',*,*,#18185,.F.);
#24402=ORIENTED_EDGE('',*,*,#18186,.T.);
#24403=ORIENTED_EDGE('',*,*,#18187,.T.);
#24404=ORIENTED_EDGE('',*,*,#18183,.F.);
#24405=ORIENTED_EDGE('',*,*,#18188,.F.);
#24406=ORIENTED_EDGE('',*,*,#18157,.T.);
#24407=ORIENTED_EDGE('',*,*,#18189,.T.);
#24408=ORIENTED_EDGE('',*,*,#18186,.F.);
#24409=ORIENTED_EDGE('',*,*,#18189,.F.);
#24410=ORIENTED_EDGE('',*,*,#18156,.F.);
#24411=ORIENTED_EDGE('',*,*,#18160,.F.);
#24412=ORIENTED_EDGE('',*,*,#18163,.F.);
#24413=ORIENTED_EDGE('',*,*,#18166,.F.);
#24414=ORIENTED_EDGE('',*,*,#18169,.F.);
#24415=ORIENTED_EDGE('',*,*,#18172,.F.);
#24416=ORIENTED_EDGE('',*,*,#18175,.F.);
#24417=ORIENTED_EDGE('',*,*,#18178,.F.);
#24418=ORIENTED_EDGE('',*,*,#18181,.F.);
#24419=ORIENTED_EDGE('',*,*,#18184,.F.);
#24420=ORIENTED_EDGE('',*,*,#18187,.F.);
#24421=ORIENTED_EDGE('',*,*,#18153,.F.);
#24422=ORIENTED_EDGE('',*,*,#18132,.F.);
#24423=ORIENTED_EDGE('',*,*,#18136,.F.);
#24424=ORIENTED_EDGE('',*,*,#18139,.F.);
#24425=ORIENTED_EDGE('',*,*,#18142,.F.);
#24426=ORIENTED_EDGE('',*,*,#18145,.F.);
#24427=ORIENTED_EDGE('',*,*,#18148,.F.);
#24428=ORIENTED_EDGE('',*,*,#18151,.F.);
#24429=ORIENTED_EDGE('',*,*,#18190,.F.);
#24430=ORIENTED_EDGE('',*,*,#18191,.T.);
#24431=ORIENTED_EDGE('',*,*,#18192,.T.);
#24432=ORIENTED_EDGE('',*,*,#18193,.F.);
#24433=ORIENTED_EDGE('',*,*,#18194,.F.);
#24434=ORIENTED_EDGE('',*,*,#18195,.T.);
#24435=ORIENTED_EDGE('',*,*,#18196,.T.);
#24436=ORIENTED_EDGE('',*,*,#18191,.F.);
#24437=ORIENTED_EDGE('',*,*,#18197,.F.);
#24438=ORIENTED_EDGE('',*,*,#18193,.T.);
#24439=ORIENTED_EDGE('',*,*,#18198,.T.);
#24440=ORIENTED_EDGE('',*,*,#18195,.F.);
#24441=ORIENTED_EDGE('',*,*,#18199,.F.);
#24442=ORIENTED_EDGE('',*,*,#18200,.T.);
#24443=ORIENTED_EDGE('',*,*,#18201,.T.);
#24444=ORIENTED_EDGE('',*,*,#18202,.F.);
#24445=ORIENTED_EDGE('',*,*,#18203,.F.);
#24446=ORIENTED_EDGE('',*,*,#18204,.T.);
#24447=ORIENTED_EDGE('',*,*,#18205,.T.);
#24448=ORIENTED_EDGE('',*,*,#18200,.F.);
#24449=ORIENTED_EDGE('',*,*,#18206,.F.);
#24450=ORIENTED_EDGE('',*,*,#18207,.T.);
#24451=ORIENTED_EDGE('',*,*,#18208,.T.);
#24452=ORIENTED_EDGE('',*,*,#18204,.F.);
#24453=ORIENTED_EDGE('',*,*,#18209,.F.);
#24454=ORIENTED_EDGE('',*,*,#18210,.T.);
#24455=ORIENTED_EDGE('',*,*,#18211,.T.);
#24456=ORIENTED_EDGE('',*,*,#18207,.F.);
#24457=ORIENTED_EDGE('',*,*,#18212,.F.);
#24458=ORIENTED_EDGE('',*,*,#18213,.T.);
#24459=ORIENTED_EDGE('',*,*,#18214,.T.);
#24460=ORIENTED_EDGE('',*,*,#18210,.F.);
#24461=ORIENTED_EDGE('',*,*,#18215,.F.);
#24462=ORIENTED_EDGE('',*,*,#18216,.T.);
#24463=ORIENTED_EDGE('',*,*,#18217,.T.);
#24464=ORIENTED_EDGE('',*,*,#18213,.F.);
#24465=ORIENTED_EDGE('',*,*,#18218,.F.);
#24466=ORIENTED_EDGE('',*,*,#18219,.T.);
#24467=ORIENTED_EDGE('',*,*,#18220,.T.);
#24468=ORIENTED_EDGE('',*,*,#18216,.F.);
#24469=ORIENTED_EDGE('',*,*,#18221,.F.);
#24470=ORIENTED_EDGE('',*,*,#18222,.T.);
#24471=ORIENTED_EDGE('',*,*,#18223,.T.);
#24472=ORIENTED_EDGE('',*,*,#18219,.F.);
#24473=ORIENTED_EDGE('',*,*,#18224,.F.);
#24474=ORIENTED_EDGE('',*,*,#18225,.T.);
#24475=ORIENTED_EDGE('',*,*,#18226,.T.);
#24476=ORIENTED_EDGE('',*,*,#18222,.F.);
#24477=ORIENTED_EDGE('',*,*,#18227,.F.);
#24478=ORIENTED_EDGE('',*,*,#18228,.T.);
#24479=ORIENTED_EDGE('',*,*,#18229,.T.);
#24480=ORIENTED_EDGE('',*,*,#18225,.F.);
#24481=ORIENTED_EDGE('',*,*,#18230,.F.);
#24482=ORIENTED_EDGE('',*,*,#18202,.T.);
#24483=ORIENTED_EDGE('',*,*,#18231,.T.);
#24484=ORIENTED_EDGE('',*,*,#18228,.F.);
#24485=ORIENTED_EDGE('',*,*,#18231,.F.);
#24486=ORIENTED_EDGE('',*,*,#18201,.F.);
#24487=ORIENTED_EDGE('',*,*,#18205,.F.);
#24488=ORIENTED_EDGE('',*,*,#18208,.F.);
#24489=ORIENTED_EDGE('',*,*,#18211,.F.);
#24490=ORIENTED_EDGE('',*,*,#18214,.F.);
#24491=ORIENTED_EDGE('',*,*,#18217,.F.);
#24492=ORIENTED_EDGE('',*,*,#18220,.F.);
#24493=ORIENTED_EDGE('',*,*,#18223,.F.);
#24494=ORIENTED_EDGE('',*,*,#18226,.F.);
#24495=ORIENTED_EDGE('',*,*,#18229,.F.);
#24496=ORIENTED_EDGE('',*,*,#18198,.F.);
#24497=ORIENTED_EDGE('',*,*,#18192,.F.);
#24498=ORIENTED_EDGE('',*,*,#18196,.F.);
#24499=ORIENTED_EDGE('',*,*,#18190,.T.);
#24500=ORIENTED_EDGE('',*,*,#18197,.T.);
#24501=ORIENTED_EDGE('',*,*,#18194,.T.);
#24502=ORIENTED_EDGE('',*,*,#18130,.T.);
#24503=ORIENTED_EDGE('',*,*,#18152,.T.);
#24504=ORIENTED_EDGE('',*,*,#18149,.T.);
#24505=ORIENTED_EDGE('',*,*,#18146,.T.);
#24506=ORIENTED_EDGE('',*,*,#18143,.T.);
#24507=ORIENTED_EDGE('',*,*,#18140,.T.);
#24508=ORIENTED_EDGE('',*,*,#18137,.T.);
#24509=ORIENTED_EDGE('',*,*,#18134,.T.);
#24510=ORIENTED_EDGE('',*,*,#18232,.F.);
#24511=ORIENTED_EDGE('',*,*,#18233,.T.);
#24512=ORIENTED_EDGE('',*,*,#18234,.T.);
#24513=ORIENTED_EDGE('',*,*,#18235,.F.);
#24514=ORIENTED_EDGE('',*,*,#18236,.F.);
#24515=ORIENTED_EDGE('',*,*,#18237,.T.);
#24516=ORIENTED_EDGE('',*,*,#18238,.T.);
#24517=ORIENTED_EDGE('',*,*,#18233,.F.);
#24518=ORIENTED_EDGE('',*,*,#18239,.F.);
#24519=ORIENTED_EDGE('',*,*,#18240,.T.);
#24520=ORIENTED_EDGE('',*,*,#18241,.T.);
#24521=ORIENTED_EDGE('',*,*,#18237,.F.);
#24522=ORIENTED_EDGE('',*,*,#18242,.F.);
#24523=ORIENTED_EDGE('',*,*,#18235,.T.);
#24524=ORIENTED_EDGE('',*,*,#18243,.T.);
#24525=ORIENTED_EDGE('',*,*,#18240,.F.);
#24526=ORIENTED_EDGE('',*,*,#18243,.F.);
#24527=ORIENTED_EDGE('',*,*,#18234,.F.);
#24528=ORIENTED_EDGE('',*,*,#18238,.F.);
#24529=ORIENTED_EDGE('',*,*,#18241,.F.);
#24530=ORIENTED_EDGE('',*,*,#18244,.F.);
#24531=ORIENTED_EDGE('',*,*,#18245,.T.);
#24532=ORIENTED_EDGE('',*,*,#18246,.T.);
#24533=ORIENTED_EDGE('',*,*,#18247,.F.);
#24534=ORIENTED_EDGE('',*,*,#18248,.F.);
#24535=ORIENTED_EDGE('',*,*,#18249,.T.);
#24536=ORIENTED_EDGE('',*,*,#18250,.T.);
#24537=ORIENTED_EDGE('',*,*,#18245,.F.);
#24538=ORIENTED_EDGE('',*,*,#18251,.F.);
#24539=ORIENTED_EDGE('',*,*,#18252,.T.);
#24540=ORIENTED_EDGE('',*,*,#18253,.T.);
#24541=ORIENTED_EDGE('',*,*,#18249,.F.);
#24542=ORIENTED_EDGE('',*,*,#18254,.F.);
#24543=ORIENTED_EDGE('',*,*,#18247,.T.);
#24544=ORIENTED_EDGE('',*,*,#18255,.T.);
#24545=ORIENTED_EDGE('',*,*,#18252,.F.);
#24546=ORIENTED_EDGE('',*,*,#18255,.F.);
#24547=ORIENTED_EDGE('',*,*,#18246,.F.);
#24548=ORIENTED_EDGE('',*,*,#18250,.F.);
#24549=ORIENTED_EDGE('',*,*,#18253,.F.);
#24550=ORIENTED_EDGE('',*,*,#18256,.F.);
#24551=ORIENTED_EDGE('',*,*,#18257,.T.);
#24552=ORIENTED_EDGE('',*,*,#18258,.T.);
#24553=ORIENTED_EDGE('',*,*,#18259,.F.);
#24554=ORIENTED_EDGE('',*,*,#18260,.F.);
#24555=ORIENTED_EDGE('',*,*,#18261,.T.);
#24556=ORIENTED_EDGE('',*,*,#18262,.T.);
#24557=ORIENTED_EDGE('',*,*,#18257,.F.);
#24558=ORIENTED_EDGE('',*,*,#18263,.F.);
#24559=ORIENTED_EDGE('',*,*,#18264,.T.);
#24560=ORIENTED_EDGE('',*,*,#18265,.T.);
#24561=ORIENTED_EDGE('',*,*,#18261,.F.);
#24562=ORIENTED_EDGE('',*,*,#18266,.F.);
#24563=ORIENTED_EDGE('',*,*,#18259,.T.);
#24564=ORIENTED_EDGE('',*,*,#18267,.T.);
#24565=ORIENTED_EDGE('',*,*,#18264,.F.);
#24566=ORIENTED_EDGE('',*,*,#18267,.F.);
#24567=ORIENTED_EDGE('',*,*,#18258,.F.);
#24568=ORIENTED_EDGE('',*,*,#18262,.F.);
#24569=ORIENTED_EDGE('',*,*,#18265,.F.);
#24570=ORIENTED_EDGE('',*,*,#18268,.F.);
#24571=ORIENTED_EDGE('',*,*,#18269,.T.);
#24572=ORIENTED_EDGE('',*,*,#18270,.T.);
#24573=ORIENTED_EDGE('',*,*,#18271,.F.);
#24574=ORIENTED_EDGE('',*,*,#18272,.F.);
#24575=ORIENTED_EDGE('',*,*,#18273,.T.);
#24576=ORIENTED_EDGE('',*,*,#18274,.T.);
#24577=ORIENTED_EDGE('',*,*,#18269,.F.);
#24578=ORIENTED_EDGE('',*,*,#18275,.F.);
#24579=ORIENTED_EDGE('',*,*,#18276,.T.);
#24580=ORIENTED_EDGE('',*,*,#18277,.T.);
#24581=ORIENTED_EDGE('',*,*,#18273,.F.);
#24582=ORIENTED_EDGE('',*,*,#18278,.F.);
#24583=ORIENTED_EDGE('',*,*,#18271,.T.);
#24584=ORIENTED_EDGE('',*,*,#18279,.T.);
#24585=ORIENTED_EDGE('',*,*,#18276,.F.);
#24586=ORIENTED_EDGE('',*,*,#18279,.F.);
#24587=ORIENTED_EDGE('',*,*,#18270,.F.);
#24588=ORIENTED_EDGE('',*,*,#18274,.F.);
#24589=ORIENTED_EDGE('',*,*,#18277,.F.);
#24590=ORIENTED_EDGE('',*,*,#18280,.F.);
#24591=ORIENTED_EDGE('',*,*,#18281,.T.);
#24592=ORIENTED_EDGE('',*,*,#18282,.T.);
#24593=ORIENTED_EDGE('',*,*,#18283,.F.);
#24594=ORIENTED_EDGE('',*,*,#18284,.F.);
#24595=ORIENTED_EDGE('',*,*,#18285,.T.);
#24596=ORIENTED_EDGE('',*,*,#18286,.T.);
#24597=ORIENTED_EDGE('',*,*,#18281,.F.);
#24598=ORIENTED_EDGE('',*,*,#18287,.F.);
#24599=ORIENTED_EDGE('',*,*,#18288,.T.);
#24600=ORIENTED_EDGE('',*,*,#18289,.T.);
#24601=ORIENTED_EDGE('',*,*,#18285,.F.);
#24602=ORIENTED_EDGE('',*,*,#18290,.F.);
#24603=ORIENTED_EDGE('',*,*,#18283,.T.);
#24604=ORIENTED_EDGE('',*,*,#18291,.T.);
#24605=ORIENTED_EDGE('',*,*,#18288,.F.);
#24606=ORIENTED_EDGE('',*,*,#18291,.F.);
#24607=ORIENTED_EDGE('',*,*,#18282,.F.);
#24608=ORIENTED_EDGE('',*,*,#18286,.F.);
#24609=ORIENTED_EDGE('',*,*,#18289,.F.);
#24610=ORIENTED_EDGE('',*,*,#18292,.F.);
#24611=ORIENTED_EDGE('',*,*,#18293,.T.);
#24612=ORIENTED_EDGE('',*,*,#18294,.T.);
#24613=ORIENTED_EDGE('',*,*,#18295,.F.);
#24614=ORIENTED_EDGE('',*,*,#18296,.F.);
#24615=ORIENTED_EDGE('',*,*,#18297,.T.);
#24616=ORIENTED_EDGE('',*,*,#18298,.T.);
#24617=ORIENTED_EDGE('',*,*,#18293,.F.);
#24618=ORIENTED_EDGE('',*,*,#18299,.F.);
#24619=ORIENTED_EDGE('',*,*,#18300,.T.);
#24620=ORIENTED_EDGE('',*,*,#18301,.T.);
#24621=ORIENTED_EDGE('',*,*,#18297,.F.);
#24622=ORIENTED_EDGE('',*,*,#18302,.F.);
#24623=ORIENTED_EDGE('',*,*,#18295,.T.);
#24624=ORIENTED_EDGE('',*,*,#18303,.T.);
#24625=ORIENTED_EDGE('',*,*,#18300,.F.);
#24626=ORIENTED_EDGE('',*,*,#18303,.F.);
#24627=ORIENTED_EDGE('',*,*,#18294,.F.);
#24628=ORIENTED_EDGE('',*,*,#18298,.F.);
#24629=ORIENTED_EDGE('',*,*,#18301,.F.);
#24630=ORIENTED_EDGE('',*,*,#18304,.F.);
#24631=ORIENTED_EDGE('',*,*,#18305,.T.);
#24632=ORIENTED_EDGE('',*,*,#18306,.T.);
#24633=ORIENTED_EDGE('',*,*,#18307,.F.);
#24634=ORIENTED_EDGE('',*,*,#18308,.F.);
#24635=ORIENTED_EDGE('',*,*,#18309,.T.);
#24636=ORIENTED_EDGE('',*,*,#18310,.T.);
#24637=ORIENTED_EDGE('',*,*,#18305,.F.);
#24638=ORIENTED_EDGE('',*,*,#18311,.F.);
#24639=ORIENTED_EDGE('',*,*,#18312,.T.);
#24640=ORIENTED_EDGE('',*,*,#18313,.T.);
#24641=ORIENTED_EDGE('',*,*,#18309,.F.);
#24642=ORIENTED_EDGE('',*,*,#18314,.F.);
#24643=ORIENTED_EDGE('',*,*,#18307,.T.);
#24644=ORIENTED_EDGE('',*,*,#18315,.T.);
#24645=ORIENTED_EDGE('',*,*,#18312,.F.);
#24646=ORIENTED_EDGE('',*,*,#18315,.F.);
#24647=ORIENTED_EDGE('',*,*,#18306,.F.);
#24648=ORIENTED_EDGE('',*,*,#18310,.F.);
#24649=ORIENTED_EDGE('',*,*,#18313,.F.);
#24650=ORIENTED_EDGE('',*,*,#18316,.F.);
#24651=ORIENTED_EDGE('',*,*,#18317,.T.);
#24652=ORIENTED_EDGE('',*,*,#18318,.T.);
#24653=ORIENTED_EDGE('',*,*,#18319,.F.);
#24654=ORIENTED_EDGE('',*,*,#18320,.F.);
#24655=ORIENTED_EDGE('',*,*,#18321,.T.);
#24656=ORIENTED_EDGE('',*,*,#18322,.T.);
#24657=ORIENTED_EDGE('',*,*,#18317,.F.);
#24658=ORIENTED_EDGE('',*,*,#18323,.F.);
#24659=ORIENTED_EDGE('',*,*,#18324,.T.);
#24660=ORIENTED_EDGE('',*,*,#18325,.T.);
#24661=ORIENTED_EDGE('',*,*,#18321,.F.);
#24662=ORIENTED_EDGE('',*,*,#18326,.F.);
#24663=ORIENTED_EDGE('',*,*,#18319,.T.);
#24664=ORIENTED_EDGE('',*,*,#18327,.T.);
#24665=ORIENTED_EDGE('',*,*,#18324,.F.);
#24666=ORIENTED_EDGE('',*,*,#18327,.F.);
#24667=ORIENTED_EDGE('',*,*,#18318,.F.);
#24668=ORIENTED_EDGE('',*,*,#18322,.F.);
#24669=ORIENTED_EDGE('',*,*,#18325,.F.);
#24670=ORIENTED_EDGE('',*,*,#18328,.F.);
#24671=ORIENTED_EDGE('',*,*,#18329,.T.);
#24672=ORIENTED_EDGE('',*,*,#18330,.T.);
#24673=ORIENTED_EDGE('',*,*,#18331,.F.);
#24674=ORIENTED_EDGE('',*,*,#18332,.F.);
#24675=ORIENTED_EDGE('',*,*,#18333,.T.);
#24676=ORIENTED_EDGE('',*,*,#18334,.T.);
#24677=ORIENTED_EDGE('',*,*,#18329,.F.);
#24678=ORIENTED_EDGE('',*,*,#18335,.F.);
#24679=ORIENTED_EDGE('',*,*,#18336,.T.);
#24680=ORIENTED_EDGE('',*,*,#18337,.T.);
#24681=ORIENTED_EDGE('',*,*,#18333,.F.);
#24682=ORIENTED_EDGE('',*,*,#18338,.F.);
#24683=ORIENTED_EDGE('',*,*,#18331,.T.);
#24684=ORIENTED_EDGE('',*,*,#18339,.T.);
#24685=ORIENTED_EDGE('',*,*,#18336,.F.);
#24686=ORIENTED_EDGE('',*,*,#18339,.F.);
#24687=ORIENTED_EDGE('',*,*,#18330,.F.);
#24688=ORIENTED_EDGE('',*,*,#18334,.F.);
#24689=ORIENTED_EDGE('',*,*,#18337,.F.);
#24690=ORIENTED_EDGE('',*,*,#18340,.F.);
#24691=ORIENTED_EDGE('',*,*,#18341,.T.);
#24692=ORIENTED_EDGE('',*,*,#18342,.T.);
#24693=ORIENTED_EDGE('',*,*,#18343,.F.);
#24694=ORIENTED_EDGE('',*,*,#18344,.F.);
#24695=ORIENTED_EDGE('',*,*,#18345,.T.);
#24696=ORIENTED_EDGE('',*,*,#18346,.T.);
#24697=ORIENTED_EDGE('',*,*,#18341,.F.);
#24698=ORIENTED_EDGE('',*,*,#18347,.F.);
#24699=ORIENTED_EDGE('',*,*,#18348,.T.);
#24700=ORIENTED_EDGE('',*,*,#18349,.T.);
#24701=ORIENTED_EDGE('',*,*,#18345,.F.);
#24702=ORIENTED_EDGE('',*,*,#18350,.F.);
#24703=ORIENTED_EDGE('',*,*,#18343,.T.);
#24704=ORIENTED_EDGE('',*,*,#18351,.T.);
#24705=ORIENTED_EDGE('',*,*,#18348,.F.);
#24706=ORIENTED_EDGE('',*,*,#18351,.F.);
#24707=ORIENTED_EDGE('',*,*,#18342,.F.);
#24708=ORIENTED_EDGE('',*,*,#18346,.F.);
#24709=ORIENTED_EDGE('',*,*,#18349,.F.);
#24710=ORIENTED_EDGE('',*,*,#18352,.F.);
#24711=ORIENTED_EDGE('',*,*,#18353,.T.);
#24712=ORIENTED_EDGE('',*,*,#18354,.T.);
#24713=ORIENTED_EDGE('',*,*,#18355,.F.);
#24714=ORIENTED_EDGE('',*,*,#18356,.F.);
#24715=ORIENTED_EDGE('',*,*,#18357,.T.);
#24716=ORIENTED_EDGE('',*,*,#18358,.T.);
#24717=ORIENTED_EDGE('',*,*,#18353,.F.);
#24718=ORIENTED_EDGE('',*,*,#18359,.F.);
#24719=ORIENTED_EDGE('',*,*,#18360,.T.);
#24720=ORIENTED_EDGE('',*,*,#18361,.T.);
#24721=ORIENTED_EDGE('',*,*,#18357,.F.);
#24722=ORIENTED_EDGE('',*,*,#18362,.F.);
#24723=ORIENTED_EDGE('',*,*,#18355,.T.);
#24724=ORIENTED_EDGE('',*,*,#18363,.T.);
#24725=ORIENTED_EDGE('',*,*,#18360,.F.);
#24726=ORIENTED_EDGE('',*,*,#18363,.F.);
#24727=ORIENTED_EDGE('',*,*,#18354,.F.);
#24728=ORIENTED_EDGE('',*,*,#18358,.F.);
#24729=ORIENTED_EDGE('',*,*,#18361,.F.);
#24730=ORIENTED_EDGE('',*,*,#18364,.F.);
#24731=ORIENTED_EDGE('',*,*,#18365,.T.);
#24732=ORIENTED_EDGE('',*,*,#18366,.T.);
#24733=ORIENTED_EDGE('',*,*,#18367,.F.);
#24734=ORIENTED_EDGE('',*,*,#18368,.F.);
#24735=ORIENTED_EDGE('',*,*,#18369,.T.);
#24736=ORIENTED_EDGE('',*,*,#18370,.T.);
#24737=ORIENTED_EDGE('',*,*,#18365,.F.);
#24738=ORIENTED_EDGE('',*,*,#18371,.F.);
#24739=ORIENTED_EDGE('',*,*,#18372,.T.);
#24740=ORIENTED_EDGE('',*,*,#18373,.T.);
#24741=ORIENTED_EDGE('',*,*,#18369,.F.);
#24742=ORIENTED_EDGE('',*,*,#18374,.F.);
#24743=ORIENTED_EDGE('',*,*,#18367,.T.);
#24744=ORIENTED_EDGE('',*,*,#18375,.T.);
#24745=ORIENTED_EDGE('',*,*,#18372,.F.);
#24746=ORIENTED_EDGE('',*,*,#18375,.F.);
#24747=ORIENTED_EDGE('',*,*,#18366,.F.);
#24748=ORIENTED_EDGE('',*,*,#18370,.F.);
#24749=ORIENTED_EDGE('',*,*,#18373,.F.);
#24750=ORIENTED_EDGE('',*,*,#18376,.F.);
#24751=ORIENTED_EDGE('',*,*,#18377,.T.);
#24752=ORIENTED_EDGE('',*,*,#18378,.T.);
#24753=ORIENTED_EDGE('',*,*,#18379,.F.);
#24754=ORIENTED_EDGE('',*,*,#18380,.F.);
#24755=ORIENTED_EDGE('',*,*,#18381,.T.);
#24756=ORIENTED_EDGE('',*,*,#18382,.T.);
#24757=ORIENTED_EDGE('',*,*,#18377,.F.);
#24758=ORIENTED_EDGE('',*,*,#18383,.F.);
#24759=ORIENTED_EDGE('',*,*,#18384,.T.);
#24760=ORIENTED_EDGE('',*,*,#18385,.T.);
#24761=ORIENTED_EDGE('',*,*,#18381,.F.);
#24762=ORIENTED_EDGE('',*,*,#18386,.F.);
#24763=ORIENTED_EDGE('',*,*,#18379,.T.);
#24764=ORIENTED_EDGE('',*,*,#18387,.T.);
#24765=ORIENTED_EDGE('',*,*,#18384,.F.);
#24766=ORIENTED_EDGE('',*,*,#18387,.F.);
#24767=ORIENTED_EDGE('',*,*,#18378,.F.);
#24768=ORIENTED_EDGE('',*,*,#18382,.F.);
#24769=ORIENTED_EDGE('',*,*,#18385,.F.);
#24770=ORIENTED_EDGE('',*,*,#18388,.F.);
#24771=ORIENTED_EDGE('',*,*,#18389,.T.);
#24772=ORIENTED_EDGE('',*,*,#18390,.T.);
#24773=ORIENTED_EDGE('',*,*,#18391,.F.);
#24774=ORIENTED_EDGE('',*,*,#18392,.F.);
#24775=ORIENTED_EDGE('',*,*,#18393,.T.);
#24776=ORIENTED_EDGE('',*,*,#18394,.T.);
#24777=ORIENTED_EDGE('',*,*,#18389,.F.);
#24778=ORIENTED_EDGE('',*,*,#18395,.F.);
#24779=ORIENTED_EDGE('',*,*,#18396,.T.);
#24780=ORIENTED_EDGE('',*,*,#18397,.T.);
#24781=ORIENTED_EDGE('',*,*,#18393,.F.);
#24782=ORIENTED_EDGE('',*,*,#18398,.F.);
#24783=ORIENTED_EDGE('',*,*,#18391,.T.);
#24784=ORIENTED_EDGE('',*,*,#18399,.T.);
#24785=ORIENTED_EDGE('',*,*,#18396,.F.);
#24786=ORIENTED_EDGE('',*,*,#18399,.F.);
#24787=ORIENTED_EDGE('',*,*,#18390,.F.);
#24788=ORIENTED_EDGE('',*,*,#18394,.F.);
#24789=ORIENTED_EDGE('',*,*,#18397,.F.);
#24790=ORIENTED_EDGE('',*,*,#18400,.F.);
#24791=ORIENTED_EDGE('',*,*,#18401,.T.);
#24792=ORIENTED_EDGE('',*,*,#18402,.T.);
#24793=ORIENTED_EDGE('',*,*,#18403,.F.);
#24794=ORIENTED_EDGE('',*,*,#18404,.F.);
#24795=ORIENTED_EDGE('',*,*,#18405,.T.);
#24796=ORIENTED_EDGE('',*,*,#18406,.T.);
#24797=ORIENTED_EDGE('',*,*,#18401,.F.);
#24798=ORIENTED_EDGE('',*,*,#18407,.F.);
#24799=ORIENTED_EDGE('',*,*,#18408,.T.);
#24800=ORIENTED_EDGE('',*,*,#18409,.T.);
#24801=ORIENTED_EDGE('',*,*,#18405,.F.);
#24802=ORIENTED_EDGE('',*,*,#18410,.F.);
#24803=ORIENTED_EDGE('',*,*,#18403,.T.);
#24804=ORIENTED_EDGE('',*,*,#18411,.T.);
#24805=ORIENTED_EDGE('',*,*,#18408,.F.);
#24806=ORIENTED_EDGE('',*,*,#18411,.F.);
#24807=ORIENTED_EDGE('',*,*,#18402,.F.);
#24808=ORIENTED_EDGE('',*,*,#18406,.F.);
#24809=ORIENTED_EDGE('',*,*,#18409,.F.);
#24810=ORIENTED_EDGE('',*,*,#18412,.F.);
#24811=ORIENTED_EDGE('',*,*,#18413,.T.);
#24812=ORIENTED_EDGE('',*,*,#18414,.T.);
#24813=ORIENTED_EDGE('',*,*,#18415,.F.);
#24814=ORIENTED_EDGE('',*,*,#18416,.F.);
#24815=ORIENTED_EDGE('',*,*,#18417,.T.);
#24816=ORIENTED_EDGE('',*,*,#18418,.T.);
#24817=ORIENTED_EDGE('',*,*,#18413,.F.);
#24818=ORIENTED_EDGE('',*,*,#18419,.F.);
#24819=ORIENTED_EDGE('',*,*,#18420,.T.);
#24820=ORIENTED_EDGE('',*,*,#18421,.T.);
#24821=ORIENTED_EDGE('',*,*,#18417,.F.);
#24822=ORIENTED_EDGE('',*,*,#18422,.F.);
#24823=ORIENTED_EDGE('',*,*,#18415,.T.);
#24824=ORIENTED_EDGE('',*,*,#18423,.T.);
#24825=ORIENTED_EDGE('',*,*,#18420,.F.);
#24826=ORIENTED_EDGE('',*,*,#18423,.F.);
#24827=ORIENTED_EDGE('',*,*,#18414,.F.);
#24828=ORIENTED_EDGE('',*,*,#18418,.F.);
#24829=ORIENTED_EDGE('',*,*,#18421,.F.);
#24830=ORIENTED_EDGE('',*,*,#18424,.F.);
#24831=ORIENTED_EDGE('',*,*,#18425,.T.);
#24832=ORIENTED_EDGE('',*,*,#18426,.T.);
#24833=ORIENTED_EDGE('',*,*,#18427,.F.);
#24834=ORIENTED_EDGE('',*,*,#18428,.F.);
#24835=ORIENTED_EDGE('',*,*,#18429,.T.);
#24836=ORIENTED_EDGE('',*,*,#18430,.T.);
#24837=ORIENTED_EDGE('',*,*,#18425,.F.);
#24838=ORIENTED_EDGE('',*,*,#18431,.F.);
#24839=ORIENTED_EDGE('',*,*,#18432,.T.);
#24840=ORIENTED_EDGE('',*,*,#18433,.T.);
#24841=ORIENTED_EDGE('',*,*,#18429,.F.);
#24842=ORIENTED_EDGE('',*,*,#18434,.F.);
#24843=ORIENTED_EDGE('',*,*,#18427,.T.);
#24844=ORIENTED_EDGE('',*,*,#18435,.T.);
#24845=ORIENTED_EDGE('',*,*,#18432,.F.);
#24846=ORIENTED_EDGE('',*,*,#18435,.F.);
#24847=ORIENTED_EDGE('',*,*,#18426,.F.);
#24848=ORIENTED_EDGE('',*,*,#18430,.F.);
#24849=ORIENTED_EDGE('',*,*,#18433,.F.);
#24850=ORIENTED_EDGE('',*,*,#18436,.F.);
#24851=ORIENTED_EDGE('',*,*,#18437,.T.);
#24852=ORIENTED_EDGE('',*,*,#18438,.T.);
#24853=ORIENTED_EDGE('',*,*,#18439,.F.);
#24854=ORIENTED_EDGE('',*,*,#18440,.F.);
#24855=ORIENTED_EDGE('',*,*,#18441,.T.);
#24856=ORIENTED_EDGE('',*,*,#18442,.T.);
#24857=ORIENTED_EDGE('',*,*,#18437,.F.);
#24858=ORIENTED_EDGE('',*,*,#18443,.F.);
#24859=ORIENTED_EDGE('',*,*,#18444,.T.);
#24860=ORIENTED_EDGE('',*,*,#18445,.T.);
#24861=ORIENTED_EDGE('',*,*,#18441,.F.);
#24862=ORIENTED_EDGE('',*,*,#18446,.F.);
#24863=ORIENTED_EDGE('',*,*,#18439,.T.);
#24864=ORIENTED_EDGE('',*,*,#18447,.T.);
#24865=ORIENTED_EDGE('',*,*,#18444,.F.);
#24866=ORIENTED_EDGE('',*,*,#18447,.F.);
#24867=ORIENTED_EDGE('',*,*,#18438,.F.);
#24868=ORIENTED_EDGE('',*,*,#18442,.F.);
#24869=ORIENTED_EDGE('',*,*,#18445,.F.);
#24870=ORIENTED_EDGE('',*,*,#18448,.F.);
#24871=ORIENTED_EDGE('',*,*,#18449,.T.);
#24872=ORIENTED_EDGE('',*,*,#18450,.T.);
#24873=ORIENTED_EDGE('',*,*,#18451,.F.);
#24874=ORIENTED_EDGE('',*,*,#18452,.F.);
#24875=ORIENTED_EDGE('',*,*,#18453,.T.);
#24876=ORIENTED_EDGE('',*,*,#18454,.T.);
#24877=ORIENTED_EDGE('',*,*,#18449,.F.);
#24878=ORIENTED_EDGE('',*,*,#18455,.F.);
#24879=ORIENTED_EDGE('',*,*,#18456,.T.);
#24880=ORIENTED_EDGE('',*,*,#18457,.T.);
#24881=ORIENTED_EDGE('',*,*,#18453,.F.);
#24882=ORIENTED_EDGE('',*,*,#18458,.F.);
#24883=ORIENTED_EDGE('',*,*,#18451,.T.);
#24884=ORIENTED_EDGE('',*,*,#18459,.T.);
#24885=ORIENTED_EDGE('',*,*,#18456,.F.);
#24886=ORIENTED_EDGE('',*,*,#18459,.F.);
#24887=ORIENTED_EDGE('',*,*,#18450,.F.);
#24888=ORIENTED_EDGE('',*,*,#18454,.F.);
#24889=ORIENTED_EDGE('',*,*,#18457,.F.);
#24890=ORIENTED_EDGE('',*,*,#18460,.F.);
#24891=ORIENTED_EDGE('',*,*,#18461,.T.);
#24892=ORIENTED_EDGE('',*,*,#18462,.T.);
#24893=ORIENTED_EDGE('',*,*,#18463,.F.);
#24894=ORIENTED_EDGE('',*,*,#18464,.F.);
#24895=ORIENTED_EDGE('',*,*,#18465,.T.);
#24896=ORIENTED_EDGE('',*,*,#18466,.T.);
#24897=ORIENTED_EDGE('',*,*,#18461,.F.);
#24898=ORIENTED_EDGE('',*,*,#18467,.F.);
#24899=ORIENTED_EDGE('',*,*,#18468,.T.);
#24900=ORIENTED_EDGE('',*,*,#18469,.T.);
#24901=ORIENTED_EDGE('',*,*,#18465,.F.);
#24902=ORIENTED_EDGE('',*,*,#18470,.F.);
#24903=ORIENTED_EDGE('',*,*,#18463,.T.);
#24904=ORIENTED_EDGE('',*,*,#18471,.T.);
#24905=ORIENTED_EDGE('',*,*,#18468,.F.);
#24906=ORIENTED_EDGE('',*,*,#18471,.F.);
#24907=ORIENTED_EDGE('',*,*,#18462,.F.);
#24908=ORIENTED_EDGE('',*,*,#18466,.F.);
#24909=ORIENTED_EDGE('',*,*,#18469,.F.);
#24910=ORIENTED_EDGE('',*,*,#18472,.F.);
#24911=ORIENTED_EDGE('',*,*,#18473,.T.);
#24912=ORIENTED_EDGE('',*,*,#18474,.T.);
#24913=ORIENTED_EDGE('',*,*,#18475,.F.);
#24914=ORIENTED_EDGE('',*,*,#18476,.F.);
#24915=ORIENTED_EDGE('',*,*,#18477,.T.);
#24916=ORIENTED_EDGE('',*,*,#18478,.T.);
#24917=ORIENTED_EDGE('',*,*,#18473,.F.);
#24918=ORIENTED_EDGE('',*,*,#18479,.F.);
#24919=ORIENTED_EDGE('',*,*,#18480,.T.);
#24920=ORIENTED_EDGE('',*,*,#18481,.T.);
#24921=ORIENTED_EDGE('',*,*,#18477,.F.);
#24922=ORIENTED_EDGE('',*,*,#18482,.F.);
#24923=ORIENTED_EDGE('',*,*,#18475,.T.);
#24924=ORIENTED_EDGE('',*,*,#18483,.T.);
#24925=ORIENTED_EDGE('',*,*,#18480,.F.);
#24926=ORIENTED_EDGE('',*,*,#18483,.F.);
#24927=ORIENTED_EDGE('',*,*,#18474,.F.);
#24928=ORIENTED_EDGE('',*,*,#18478,.F.);
#24929=ORIENTED_EDGE('',*,*,#18481,.F.);
#24930=ORIENTED_EDGE('',*,*,#18484,.F.);
#24931=ORIENTED_EDGE('',*,*,#18485,.T.);
#24932=ORIENTED_EDGE('',*,*,#18486,.T.);
#24933=ORIENTED_EDGE('',*,*,#18487,.F.);
#24934=ORIENTED_EDGE('',*,*,#18488,.F.);
#24935=ORIENTED_EDGE('',*,*,#18489,.T.);
#24936=ORIENTED_EDGE('',*,*,#18490,.T.);
#24937=ORIENTED_EDGE('',*,*,#18485,.F.);
#24938=ORIENTED_EDGE('',*,*,#18491,.F.);
#24939=ORIENTED_EDGE('',*,*,#18492,.T.);
#24940=ORIENTED_EDGE('',*,*,#18493,.T.);
#24941=ORIENTED_EDGE('',*,*,#18489,.F.);
#24942=ORIENTED_EDGE('',*,*,#18494,.F.);
#24943=ORIENTED_EDGE('',*,*,#18487,.T.);
#24944=ORIENTED_EDGE('',*,*,#18495,.T.);
#24945=ORIENTED_EDGE('',*,*,#18492,.F.);
#24946=ORIENTED_EDGE('',*,*,#18495,.F.);
#24947=ORIENTED_EDGE('',*,*,#18486,.F.);
#24948=ORIENTED_EDGE('',*,*,#18490,.F.);
#24949=ORIENTED_EDGE('',*,*,#18493,.F.);
#24950=ORIENTED_EDGE('',*,*,#18496,.F.);
#24951=ORIENTED_EDGE('',*,*,#18497,.T.);
#24952=ORIENTED_EDGE('',*,*,#18498,.T.);
#24953=ORIENTED_EDGE('',*,*,#18499,.F.);
#24954=ORIENTED_EDGE('',*,*,#18500,.F.);
#24955=ORIENTED_EDGE('',*,*,#18501,.T.);
#24956=ORIENTED_EDGE('',*,*,#18502,.T.);
#24957=ORIENTED_EDGE('',*,*,#18497,.F.);
#24958=ORIENTED_EDGE('',*,*,#18503,.F.);
#24959=ORIENTED_EDGE('',*,*,#18504,.T.);
#24960=ORIENTED_EDGE('',*,*,#18505,.T.);
#24961=ORIENTED_EDGE('',*,*,#18501,.F.);
#24962=ORIENTED_EDGE('',*,*,#18506,.F.);
#24963=ORIENTED_EDGE('',*,*,#18499,.T.);
#24964=ORIENTED_EDGE('',*,*,#18507,.T.);
#24965=ORIENTED_EDGE('',*,*,#18504,.F.);
#24966=ORIENTED_EDGE('',*,*,#18507,.F.);
#24967=ORIENTED_EDGE('',*,*,#18498,.F.);
#24968=ORIENTED_EDGE('',*,*,#18502,.F.);
#24969=ORIENTED_EDGE('',*,*,#18505,.F.);
#24970=ORIENTED_EDGE('',*,*,#18508,.F.);
#24971=ORIENTED_EDGE('',*,*,#18509,.T.);
#24972=ORIENTED_EDGE('',*,*,#18510,.T.);
#24973=ORIENTED_EDGE('',*,*,#18511,.F.);
#24974=ORIENTED_EDGE('',*,*,#18512,.F.);
#24975=ORIENTED_EDGE('',*,*,#18513,.T.);
#24976=ORIENTED_EDGE('',*,*,#18514,.T.);
#24977=ORIENTED_EDGE('',*,*,#18509,.F.);
#24978=ORIENTED_EDGE('',*,*,#18515,.F.);
#24979=ORIENTED_EDGE('',*,*,#18516,.T.);
#24980=ORIENTED_EDGE('',*,*,#18517,.T.);
#24981=ORIENTED_EDGE('',*,*,#18513,.F.);
#24982=ORIENTED_EDGE('',*,*,#18518,.F.);
#24983=ORIENTED_EDGE('',*,*,#18511,.T.);
#24984=ORIENTED_EDGE('',*,*,#18519,.T.);
#24985=ORIENTED_EDGE('',*,*,#18516,.F.);
#24986=ORIENTED_EDGE('',*,*,#18519,.F.);
#24987=ORIENTED_EDGE('',*,*,#18510,.F.);
#24988=ORIENTED_EDGE('',*,*,#18514,.F.);
#24989=ORIENTED_EDGE('',*,*,#18517,.F.);
#24990=ORIENTED_EDGE('',*,*,#18520,.F.);
#24991=ORIENTED_EDGE('',*,*,#18521,.T.);
#24992=ORIENTED_EDGE('',*,*,#18522,.T.);
#24993=ORIENTED_EDGE('',*,*,#18523,.F.);
#24994=ORIENTED_EDGE('',*,*,#18524,.F.);
#24995=ORIENTED_EDGE('',*,*,#18525,.T.);
#24996=ORIENTED_EDGE('',*,*,#18526,.T.);
#24997=ORIENTED_EDGE('',*,*,#18521,.F.);
#24998=ORIENTED_EDGE('',*,*,#18527,.F.);
#24999=ORIENTED_EDGE('',*,*,#18528,.T.);
#25000=ORIENTED_EDGE('',*,*,#18529,.T.);
#25001=ORIENTED_EDGE('',*,*,#18525,.F.);
#25002=ORIENTED_EDGE('',*,*,#18530,.F.);
#25003=ORIENTED_EDGE('',*,*,#18523,.T.);
#25004=ORIENTED_EDGE('',*,*,#18531,.T.);
#25005=ORIENTED_EDGE('',*,*,#18528,.F.);
#25006=ORIENTED_EDGE('',*,*,#18531,.F.);
#25007=ORIENTED_EDGE('',*,*,#18522,.F.);
#25008=ORIENTED_EDGE('',*,*,#18526,.F.);
#25009=ORIENTED_EDGE('',*,*,#18529,.F.);
#25010=ORIENTED_EDGE('',*,*,#18532,.F.);
#25011=ORIENTED_EDGE('',*,*,#18533,.T.);
#25012=ORIENTED_EDGE('',*,*,#18534,.T.);
#25013=ORIENTED_EDGE('',*,*,#18535,.F.);
#25014=ORIENTED_EDGE('',*,*,#18536,.F.);
#25015=ORIENTED_EDGE('',*,*,#18537,.T.);
#25016=ORIENTED_EDGE('',*,*,#18538,.T.);
#25017=ORIENTED_EDGE('',*,*,#18533,.F.);
#25018=ORIENTED_EDGE('',*,*,#18539,.F.);
#25019=ORIENTED_EDGE('',*,*,#18540,.T.);
#25020=ORIENTED_EDGE('',*,*,#18541,.T.);
#25021=ORIENTED_EDGE('',*,*,#18537,.F.);
#25022=ORIENTED_EDGE('',*,*,#18542,.F.);
#25023=ORIENTED_EDGE('',*,*,#18535,.T.);
#25024=ORIENTED_EDGE('',*,*,#18543,.T.);
#25025=ORIENTED_EDGE('',*,*,#18540,.F.);
#25026=ORIENTED_EDGE('',*,*,#18543,.F.);
#25027=ORIENTED_EDGE('',*,*,#18534,.F.);
#25028=ORIENTED_EDGE('',*,*,#18538,.F.);
#25029=ORIENTED_EDGE('',*,*,#18541,.F.);
#25030=ORIENTED_EDGE('',*,*,#18544,.F.);
#25031=ORIENTED_EDGE('',*,*,#18545,.T.);
#25032=ORIENTED_EDGE('',*,*,#18546,.T.);
#25033=ORIENTED_EDGE('',*,*,#18547,.F.);
#25034=ORIENTED_EDGE('',*,*,#18548,.F.);
#25035=ORIENTED_EDGE('',*,*,#18549,.T.);
#25036=ORIENTED_EDGE('',*,*,#18550,.T.);
#25037=ORIENTED_EDGE('',*,*,#18545,.F.);
#25038=ORIENTED_EDGE('',*,*,#18551,.F.);
#25039=ORIENTED_EDGE('',*,*,#18552,.T.);
#25040=ORIENTED_EDGE('',*,*,#18553,.T.);
#25041=ORIENTED_EDGE('',*,*,#18549,.F.);
#25042=ORIENTED_EDGE('',*,*,#18554,.F.);
#25043=ORIENTED_EDGE('',*,*,#18547,.T.);
#25044=ORIENTED_EDGE('',*,*,#18555,.T.);
#25045=ORIENTED_EDGE('',*,*,#18552,.F.);
#25046=ORIENTED_EDGE('',*,*,#18555,.F.);
#25047=ORIENTED_EDGE('',*,*,#18546,.F.);
#25048=ORIENTED_EDGE('',*,*,#18550,.F.);
#25049=ORIENTED_EDGE('',*,*,#18553,.F.);
#25050=ORIENTED_EDGE('',*,*,#18556,.F.);
#25051=ORIENTED_EDGE('',*,*,#18557,.T.);
#25052=ORIENTED_EDGE('',*,*,#18558,.T.);
#25053=ORIENTED_EDGE('',*,*,#18559,.F.);
#25054=ORIENTED_EDGE('',*,*,#18560,.F.);
#25055=ORIENTED_EDGE('',*,*,#18561,.T.);
#25056=ORIENTED_EDGE('',*,*,#18562,.T.);
#25057=ORIENTED_EDGE('',*,*,#18557,.F.);
#25058=ORIENTED_EDGE('',*,*,#18563,.F.);
#25059=ORIENTED_EDGE('',*,*,#18564,.T.);
#25060=ORIENTED_EDGE('',*,*,#18565,.T.);
#25061=ORIENTED_EDGE('',*,*,#18561,.F.);
#25062=ORIENTED_EDGE('',*,*,#18566,.F.);
#25063=ORIENTED_EDGE('',*,*,#18559,.T.);
#25064=ORIENTED_EDGE('',*,*,#18567,.T.);
#25065=ORIENTED_EDGE('',*,*,#18564,.F.);
#25066=ORIENTED_EDGE('',*,*,#18567,.F.);
#25067=ORIENTED_EDGE('',*,*,#18558,.F.);
#25068=ORIENTED_EDGE('',*,*,#18562,.F.);
#25069=ORIENTED_EDGE('',*,*,#18565,.F.);
#25070=ORIENTED_EDGE('',*,*,#18568,.F.);
#25071=ORIENTED_EDGE('',*,*,#18569,.T.);
#25072=ORIENTED_EDGE('',*,*,#18570,.T.);
#25073=ORIENTED_EDGE('',*,*,#18571,.F.);
#25074=ORIENTED_EDGE('',*,*,#18572,.F.);
#25075=ORIENTED_EDGE('',*,*,#18573,.T.);
#25076=ORIENTED_EDGE('',*,*,#18574,.T.);
#25077=ORIENTED_EDGE('',*,*,#18569,.F.);
#25078=ORIENTED_EDGE('',*,*,#18575,.F.);
#25079=ORIENTED_EDGE('',*,*,#18576,.T.);
#25080=ORIENTED_EDGE('',*,*,#18577,.T.);
#25081=ORIENTED_EDGE('',*,*,#18573,.F.);
#25082=ORIENTED_EDGE('',*,*,#18578,.F.);
#25083=ORIENTED_EDGE('',*,*,#18571,.T.);
#25084=ORIENTED_EDGE('',*,*,#18579,.T.);
#25085=ORIENTED_EDGE('',*,*,#18576,.F.);
#25086=ORIENTED_EDGE('',*,*,#18579,.F.);
#25087=ORIENTED_EDGE('',*,*,#18570,.F.);
#25088=ORIENTED_EDGE('',*,*,#18574,.F.);
#25089=ORIENTED_EDGE('',*,*,#18577,.F.);
#25090=ORIENTED_EDGE('',*,*,#18580,.F.);
#25091=ORIENTED_EDGE('',*,*,#18581,.T.);
#25092=ORIENTED_EDGE('',*,*,#18582,.T.);
#25093=ORIENTED_EDGE('',*,*,#18583,.F.);
#25094=ORIENTED_EDGE('',*,*,#18584,.F.);
#25095=ORIENTED_EDGE('',*,*,#18585,.T.);
#25096=ORIENTED_EDGE('',*,*,#18586,.T.);
#25097=ORIENTED_EDGE('',*,*,#18581,.F.);
#25098=ORIENTED_EDGE('',*,*,#18587,.F.);
#25099=ORIENTED_EDGE('',*,*,#18588,.T.);
#25100=ORIENTED_EDGE('',*,*,#18589,.T.);
#25101=ORIENTED_EDGE('',*,*,#18585,.F.);
#25102=ORIENTED_EDGE('',*,*,#18590,.F.);
#25103=ORIENTED_EDGE('',*,*,#18583,.T.);
#25104=ORIENTED_EDGE('',*,*,#18591,.T.);
#25105=ORIENTED_EDGE('',*,*,#18588,.F.);
#25106=ORIENTED_EDGE('',*,*,#18591,.F.);
#25107=ORIENTED_EDGE('',*,*,#18582,.F.);
#25108=ORIENTED_EDGE('',*,*,#18586,.F.);
#25109=ORIENTED_EDGE('',*,*,#18589,.F.);
#25110=ORIENTED_EDGE('',*,*,#18592,.F.);
#25111=ORIENTED_EDGE('',*,*,#18593,.T.);
#25112=ORIENTED_EDGE('',*,*,#18594,.T.);
#25113=ORIENTED_EDGE('',*,*,#18595,.F.);
#25114=ORIENTED_EDGE('',*,*,#18596,.F.);
#25115=ORIENTED_EDGE('',*,*,#18597,.T.);
#25116=ORIENTED_EDGE('',*,*,#18598,.T.);
#25117=ORIENTED_EDGE('',*,*,#18593,.F.);
#25118=ORIENTED_EDGE('',*,*,#18599,.F.);
#25119=ORIENTED_EDGE('',*,*,#18600,.T.);
#25120=ORIENTED_EDGE('',*,*,#18601,.T.);
#25121=ORIENTED_EDGE('',*,*,#18597,.F.);
#25122=ORIENTED_EDGE('',*,*,#18602,.F.);
#25123=ORIENTED_EDGE('',*,*,#18595,.T.);
#25124=ORIENTED_EDGE('',*,*,#18603,.T.);
#25125=ORIENTED_EDGE('',*,*,#18600,.F.);
#25126=ORIENTED_EDGE('',*,*,#18603,.F.);
#25127=ORIENTED_EDGE('',*,*,#18594,.F.);
#25128=ORIENTED_EDGE('',*,*,#18598,.F.);
#25129=ORIENTED_EDGE('',*,*,#18601,.F.);
#25130=ORIENTED_EDGE('',*,*,#18604,.F.);
#25131=ORIENTED_EDGE('',*,*,#18605,.T.);
#25132=ORIENTED_EDGE('',*,*,#18606,.T.);
#25133=ORIENTED_EDGE('',*,*,#18607,.F.);
#25134=ORIENTED_EDGE('',*,*,#18608,.F.);
#25135=ORIENTED_EDGE('',*,*,#18609,.T.);
#25136=ORIENTED_EDGE('',*,*,#18610,.T.);
#25137=ORIENTED_EDGE('',*,*,#18605,.F.);
#25138=ORIENTED_EDGE('',*,*,#18611,.F.);
#25139=ORIENTED_EDGE('',*,*,#18612,.T.);
#25140=ORIENTED_EDGE('',*,*,#18613,.T.);
#25141=ORIENTED_EDGE('',*,*,#18609,.F.);
#25142=ORIENTED_EDGE('',*,*,#18614,.F.);
#25143=ORIENTED_EDGE('',*,*,#18607,.T.);
#25144=ORIENTED_EDGE('',*,*,#18615,.T.);
#25145=ORIENTED_EDGE('',*,*,#18612,.F.);
#25146=ORIENTED_EDGE('',*,*,#18615,.F.);
#25147=ORIENTED_EDGE('',*,*,#18606,.F.);
#25148=ORIENTED_EDGE('',*,*,#18610,.F.);
#25149=ORIENTED_EDGE('',*,*,#18613,.F.);
#25150=ORIENTED_EDGE('',*,*,#18616,.F.);
#25151=ORIENTED_EDGE('',*,*,#18617,.T.);
#25152=ORIENTED_EDGE('',*,*,#18618,.T.);
#25153=ORIENTED_EDGE('',*,*,#18619,.F.);
#25154=ORIENTED_EDGE('',*,*,#18620,.F.);
#25155=ORIENTED_EDGE('',*,*,#18621,.T.);
#25156=ORIENTED_EDGE('',*,*,#18622,.T.);
#25157=ORIENTED_EDGE('',*,*,#18617,.F.);
#25158=ORIENTED_EDGE('',*,*,#18623,.F.);
#25159=ORIENTED_EDGE('',*,*,#18624,.T.);
#25160=ORIENTED_EDGE('',*,*,#18625,.T.);
#25161=ORIENTED_EDGE('',*,*,#18621,.F.);
#25162=ORIENTED_EDGE('',*,*,#18626,.F.);
#25163=ORIENTED_EDGE('',*,*,#18619,.T.);
#25164=ORIENTED_EDGE('',*,*,#18627,.T.);
#25165=ORIENTED_EDGE('',*,*,#18624,.F.);
#25166=ORIENTED_EDGE('',*,*,#18627,.F.);
#25167=ORIENTED_EDGE('',*,*,#18618,.F.);
#25168=ORIENTED_EDGE('',*,*,#18622,.F.);
#25169=ORIENTED_EDGE('',*,*,#18625,.F.);
#25170=ORIENTED_EDGE('',*,*,#18628,.F.);
#25171=ORIENTED_EDGE('',*,*,#18629,.T.);
#25172=ORIENTED_EDGE('',*,*,#18630,.T.);
#25173=ORIENTED_EDGE('',*,*,#18631,.F.);
#25174=ORIENTED_EDGE('',*,*,#18632,.F.);
#25175=ORIENTED_EDGE('',*,*,#18633,.T.);
#25176=ORIENTED_EDGE('',*,*,#18634,.T.);
#25177=ORIENTED_EDGE('',*,*,#18629,.F.);
#25178=ORIENTED_EDGE('',*,*,#18635,.F.);
#25179=ORIENTED_EDGE('',*,*,#18636,.T.);
#25180=ORIENTED_EDGE('',*,*,#18637,.T.);
#25181=ORIENTED_EDGE('',*,*,#18633,.F.);
#25182=ORIENTED_EDGE('',*,*,#18638,.F.);
#25183=ORIENTED_EDGE('',*,*,#18631,.T.);
#25184=ORIENTED_EDGE('',*,*,#18639,.T.);
#25185=ORIENTED_EDGE('',*,*,#18636,.F.);
#25186=ORIENTED_EDGE('',*,*,#18639,.F.);
#25187=ORIENTED_EDGE('',*,*,#18630,.F.);
#25188=ORIENTED_EDGE('',*,*,#18634,.F.);
#25189=ORIENTED_EDGE('',*,*,#18637,.F.);
#25190=ORIENTED_EDGE('',*,*,#18640,.F.);
#25191=ORIENTED_EDGE('',*,*,#18641,.T.);
#25192=ORIENTED_EDGE('',*,*,#18642,.T.);
#25193=ORIENTED_EDGE('',*,*,#18643,.F.);
#25194=ORIENTED_EDGE('',*,*,#18644,.F.);
#25195=ORIENTED_EDGE('',*,*,#18645,.T.);
#25196=ORIENTED_EDGE('',*,*,#18646,.T.);
#25197=ORIENTED_EDGE('',*,*,#18641,.F.);
#25198=ORIENTED_EDGE('',*,*,#18647,.F.);
#25199=ORIENTED_EDGE('',*,*,#18648,.T.);
#25200=ORIENTED_EDGE('',*,*,#18649,.T.);
#25201=ORIENTED_EDGE('',*,*,#18645,.F.);
#25202=ORIENTED_EDGE('',*,*,#18650,.F.);
#25203=ORIENTED_EDGE('',*,*,#18643,.T.);
#25204=ORIENTED_EDGE('',*,*,#18651,.T.);
#25205=ORIENTED_EDGE('',*,*,#18648,.F.);
#25206=ORIENTED_EDGE('',*,*,#18651,.F.);
#25207=ORIENTED_EDGE('',*,*,#18642,.F.);
#25208=ORIENTED_EDGE('',*,*,#18646,.F.);
#25209=ORIENTED_EDGE('',*,*,#18649,.F.);
#25210=ORIENTED_EDGE('',*,*,#18652,.F.);
#25211=ORIENTED_EDGE('',*,*,#18653,.T.);
#25212=ORIENTED_EDGE('',*,*,#18654,.T.);
#25213=ORIENTED_EDGE('',*,*,#18655,.F.);
#25214=ORIENTED_EDGE('',*,*,#18656,.F.);
#25215=ORIENTED_EDGE('',*,*,#18657,.T.);
#25216=ORIENTED_EDGE('',*,*,#18658,.T.);
#25217=ORIENTED_EDGE('',*,*,#18653,.F.);
#25218=ORIENTED_EDGE('',*,*,#18659,.F.);
#25219=ORIENTED_EDGE('',*,*,#18660,.T.);
#25220=ORIENTED_EDGE('',*,*,#18661,.T.);
#25221=ORIENTED_EDGE('',*,*,#18657,.F.);
#25222=ORIENTED_EDGE('',*,*,#18662,.F.);
#25223=ORIENTED_EDGE('',*,*,#18655,.T.);
#25224=ORIENTED_EDGE('',*,*,#18663,.T.);
#25225=ORIENTED_EDGE('',*,*,#18660,.F.);
#25226=ORIENTED_EDGE('',*,*,#18663,.F.);
#25227=ORIENTED_EDGE('',*,*,#18654,.F.);
#25228=ORIENTED_EDGE('',*,*,#18658,.F.);
#25229=ORIENTED_EDGE('',*,*,#18661,.F.);
#25230=ORIENTED_EDGE('',*,*,#18664,.F.);
#25231=ORIENTED_EDGE('',*,*,#18665,.T.);
#25232=ORIENTED_EDGE('',*,*,#18666,.T.);
#25233=ORIENTED_EDGE('',*,*,#18667,.F.);
#25234=ORIENTED_EDGE('',*,*,#18668,.F.);
#25235=ORIENTED_EDGE('',*,*,#18669,.T.);
#25236=ORIENTED_EDGE('',*,*,#18670,.T.);
#25237=ORIENTED_EDGE('',*,*,#18665,.F.);
#25238=ORIENTED_EDGE('',*,*,#18671,.F.);
#25239=ORIENTED_EDGE('',*,*,#18672,.T.);
#25240=ORIENTED_EDGE('',*,*,#18673,.T.);
#25241=ORIENTED_EDGE('',*,*,#18669,.F.);
#25242=ORIENTED_EDGE('',*,*,#18674,.F.);
#25243=ORIENTED_EDGE('',*,*,#18667,.T.);
#25244=ORIENTED_EDGE('',*,*,#18675,.T.);
#25245=ORIENTED_EDGE('',*,*,#18672,.F.);
#25246=ORIENTED_EDGE('',*,*,#18675,.F.);
#25247=ORIENTED_EDGE('',*,*,#18666,.F.);
#25248=ORIENTED_EDGE('',*,*,#18670,.F.);
#25249=ORIENTED_EDGE('',*,*,#18673,.F.);
#25250=ORIENTED_EDGE('',*,*,#18676,.F.);
#25251=ORIENTED_EDGE('',*,*,#18677,.T.);
#25252=ORIENTED_EDGE('',*,*,#18678,.T.);
#25253=ORIENTED_EDGE('',*,*,#18679,.F.);
#25254=ORIENTED_EDGE('',*,*,#18680,.F.);
#25255=ORIENTED_EDGE('',*,*,#18681,.T.);
#25256=ORIENTED_EDGE('',*,*,#18682,.T.);
#25257=ORIENTED_EDGE('',*,*,#18677,.F.);
#25258=ORIENTED_EDGE('',*,*,#18683,.F.);
#25259=ORIENTED_EDGE('',*,*,#18684,.T.);
#25260=ORIENTED_EDGE('',*,*,#18685,.T.);
#25261=ORIENTED_EDGE('',*,*,#18681,.F.);
#25262=ORIENTED_EDGE('',*,*,#18686,.F.);
#25263=ORIENTED_EDGE('',*,*,#18679,.T.);
#25264=ORIENTED_EDGE('',*,*,#18687,.T.);
#25265=ORIENTED_EDGE('',*,*,#18684,.F.);
#25266=ORIENTED_EDGE('',*,*,#18687,.F.);
#25267=ORIENTED_EDGE('',*,*,#18678,.F.);
#25268=ORIENTED_EDGE('',*,*,#18682,.F.);
#25269=ORIENTED_EDGE('',*,*,#18685,.F.);
#25270=ORIENTED_EDGE('',*,*,#18688,.F.);
#25271=ORIENTED_EDGE('',*,*,#18689,.T.);
#25272=ORIENTED_EDGE('',*,*,#18690,.T.);
#25273=ORIENTED_EDGE('',*,*,#18691,.F.);
#25274=ORIENTED_EDGE('',*,*,#18692,.F.);
#25275=ORIENTED_EDGE('',*,*,#18693,.T.);
#25276=ORIENTED_EDGE('',*,*,#18694,.T.);
#25277=ORIENTED_EDGE('',*,*,#18689,.F.);
#25278=ORIENTED_EDGE('',*,*,#18695,.F.);
#25279=ORIENTED_EDGE('',*,*,#18696,.T.);
#25280=ORIENTED_EDGE('',*,*,#18697,.T.);
#25281=ORIENTED_EDGE('',*,*,#18693,.F.);
#25282=ORIENTED_EDGE('',*,*,#18698,.F.);
#25283=ORIENTED_EDGE('',*,*,#18691,.T.);
#25284=ORIENTED_EDGE('',*,*,#18699,.T.);
#25285=ORIENTED_EDGE('',*,*,#18696,.F.);
#25286=ORIENTED_EDGE('',*,*,#18699,.F.);
#25287=ORIENTED_EDGE('',*,*,#18690,.F.);
#25288=ORIENTED_EDGE('',*,*,#18694,.F.);
#25289=ORIENTED_EDGE('',*,*,#18697,.F.);
#25290=ORIENTED_EDGE('',*,*,#18700,.F.);
#25291=ORIENTED_EDGE('',*,*,#18701,.T.);
#25292=ORIENTED_EDGE('',*,*,#18702,.T.);
#25293=ORIENTED_EDGE('',*,*,#18703,.F.);
#25294=ORIENTED_EDGE('',*,*,#18704,.F.);
#25295=ORIENTED_EDGE('',*,*,#18705,.T.);
#25296=ORIENTED_EDGE('',*,*,#18706,.T.);
#25297=ORIENTED_EDGE('',*,*,#18701,.F.);
#25298=ORIENTED_EDGE('',*,*,#18707,.F.);
#25299=ORIENTED_EDGE('',*,*,#18708,.T.);
#25300=ORIENTED_EDGE('',*,*,#18709,.T.);
#25301=ORIENTED_EDGE('',*,*,#18705,.F.);
#25302=ORIENTED_EDGE('',*,*,#18710,.F.);
#25303=ORIENTED_EDGE('',*,*,#18703,.T.);
#25304=ORIENTED_EDGE('',*,*,#18711,.T.);
#25305=ORIENTED_EDGE('',*,*,#18708,.F.);
#25306=ORIENTED_EDGE('',*,*,#18711,.F.);
#25307=ORIENTED_EDGE('',*,*,#18702,.F.);
#25308=ORIENTED_EDGE('',*,*,#18706,.F.);
#25309=ORIENTED_EDGE('',*,*,#18709,.F.);
#25310=ORIENTED_EDGE('',*,*,#18712,.F.);
#25311=ORIENTED_EDGE('',*,*,#18713,.T.);
#25312=ORIENTED_EDGE('',*,*,#18714,.T.);
#25313=ORIENTED_EDGE('',*,*,#18715,.F.);
#25314=ORIENTED_EDGE('',*,*,#18716,.F.);
#25315=ORIENTED_EDGE('',*,*,#18717,.T.);
#25316=ORIENTED_EDGE('',*,*,#18718,.T.);
#25317=ORIENTED_EDGE('',*,*,#18713,.F.);
#25318=ORIENTED_EDGE('',*,*,#18719,.F.);
#25319=ORIENTED_EDGE('',*,*,#18720,.T.);
#25320=ORIENTED_EDGE('',*,*,#18721,.T.);
#25321=ORIENTED_EDGE('',*,*,#18717,.F.);
#25322=ORIENTED_EDGE('',*,*,#18722,.F.);
#25323=ORIENTED_EDGE('',*,*,#18715,.T.);
#25324=ORIENTED_EDGE('',*,*,#18723,.T.);
#25325=ORIENTED_EDGE('',*,*,#18720,.F.);
#25326=ORIENTED_EDGE('',*,*,#18723,.F.);
#25327=ORIENTED_EDGE('',*,*,#18714,.F.);
#25328=ORIENTED_EDGE('',*,*,#18718,.F.);
#25329=ORIENTED_EDGE('',*,*,#18721,.F.);
#25330=ORIENTED_EDGE('',*,*,#18724,.F.);
#25331=ORIENTED_EDGE('',*,*,#18725,.T.);
#25332=ORIENTED_EDGE('',*,*,#18726,.T.);
#25333=ORIENTED_EDGE('',*,*,#18727,.F.);
#25334=ORIENTED_EDGE('',*,*,#18728,.F.);
#25335=ORIENTED_EDGE('',*,*,#18729,.T.);
#25336=ORIENTED_EDGE('',*,*,#18730,.T.);
#25337=ORIENTED_EDGE('',*,*,#18725,.F.);
#25338=ORIENTED_EDGE('',*,*,#18731,.F.);
#25339=ORIENTED_EDGE('',*,*,#18732,.T.);
#25340=ORIENTED_EDGE('',*,*,#18733,.T.);
#25341=ORIENTED_EDGE('',*,*,#18729,.F.);
#25342=ORIENTED_EDGE('',*,*,#18734,.F.);
#25343=ORIENTED_EDGE('',*,*,#18727,.T.);
#25344=ORIENTED_EDGE('',*,*,#18735,.T.);
#25345=ORIENTED_EDGE('',*,*,#18732,.F.);
#25346=ORIENTED_EDGE('',*,*,#18735,.F.);
#25347=ORIENTED_EDGE('',*,*,#18726,.F.);
#25348=ORIENTED_EDGE('',*,*,#18730,.F.);
#25349=ORIENTED_EDGE('',*,*,#18733,.F.);
#25350=ORIENTED_EDGE('',*,*,#18736,.F.);
#25351=ORIENTED_EDGE('',*,*,#18737,.T.);
#25352=ORIENTED_EDGE('',*,*,#18738,.T.);
#25353=ORIENTED_EDGE('',*,*,#18739,.F.);
#25354=ORIENTED_EDGE('',*,*,#18740,.F.);
#25355=ORIENTED_EDGE('',*,*,#18741,.T.);
#25356=ORIENTED_EDGE('',*,*,#18742,.T.);
#25357=ORIENTED_EDGE('',*,*,#18737,.F.);
#25358=ORIENTED_EDGE('',*,*,#18743,.F.);
#25359=ORIENTED_EDGE('',*,*,#18744,.T.);
#25360=ORIENTED_EDGE('',*,*,#18745,.T.);
#25361=ORIENTED_EDGE('',*,*,#18741,.F.);
#25362=ORIENTED_EDGE('',*,*,#18746,.F.);
#25363=ORIENTED_EDGE('',*,*,#18739,.T.);
#25364=ORIENTED_EDGE('',*,*,#18747,.T.);
#25365=ORIENTED_EDGE('',*,*,#18744,.F.);
#25366=ORIENTED_EDGE('',*,*,#18747,.F.);
#25367=ORIENTED_EDGE('',*,*,#18738,.F.);
#25368=ORIENTED_EDGE('',*,*,#18742,.F.);
#25369=ORIENTED_EDGE('',*,*,#18745,.F.);
#25370=ORIENTED_EDGE('',*,*,#18748,.F.);
#25371=ORIENTED_EDGE('',*,*,#18749,.T.);
#25372=ORIENTED_EDGE('',*,*,#18750,.T.);
#25373=ORIENTED_EDGE('',*,*,#18751,.F.);
#25374=ORIENTED_EDGE('',*,*,#18752,.F.);
#25375=ORIENTED_EDGE('',*,*,#18753,.T.);
#25376=ORIENTED_EDGE('',*,*,#18754,.T.);
#25377=ORIENTED_EDGE('',*,*,#18749,.F.);
#25378=ORIENTED_EDGE('',*,*,#18755,.F.);
#25379=ORIENTED_EDGE('',*,*,#18756,.T.);
#25380=ORIENTED_EDGE('',*,*,#18757,.T.);
#25381=ORIENTED_EDGE('',*,*,#18753,.F.);
#25382=ORIENTED_EDGE('',*,*,#18758,.F.);
#25383=ORIENTED_EDGE('',*,*,#18751,.T.);
#25384=ORIENTED_EDGE('',*,*,#18759,.T.);
#25385=ORIENTED_EDGE('',*,*,#18756,.F.);
#25386=ORIENTED_EDGE('',*,*,#18759,.F.);
#25387=ORIENTED_EDGE('',*,*,#18750,.F.);
#25388=ORIENTED_EDGE('',*,*,#18754,.F.);
#25389=ORIENTED_EDGE('',*,*,#18757,.F.);
#25390=ORIENTED_EDGE('',*,*,#18760,.F.);
#25391=ORIENTED_EDGE('',*,*,#18761,.T.);
#25392=ORIENTED_EDGE('',*,*,#18762,.T.);
#25393=ORIENTED_EDGE('',*,*,#18763,.F.);
#25394=ORIENTED_EDGE('',*,*,#18764,.F.);
#25395=ORIENTED_EDGE('',*,*,#18765,.T.);
#25396=ORIENTED_EDGE('',*,*,#18766,.T.);
#25397=ORIENTED_EDGE('',*,*,#18761,.F.);
#25398=ORIENTED_EDGE('',*,*,#18767,.F.);
#25399=ORIENTED_EDGE('',*,*,#18768,.T.);
#25400=ORIENTED_EDGE('',*,*,#18769,.T.);
#25401=ORIENTED_EDGE('',*,*,#18765,.F.);
#25402=ORIENTED_EDGE('',*,*,#18770,.F.);
#25403=ORIENTED_EDGE('',*,*,#18763,.T.);
#25404=ORIENTED_EDGE('',*,*,#18771,.T.);
#25405=ORIENTED_EDGE('',*,*,#18768,.F.);
#25406=ORIENTED_EDGE('',*,*,#18771,.F.);
#25407=ORIENTED_EDGE('',*,*,#18762,.F.);
#25408=ORIENTED_EDGE('',*,*,#18766,.F.);
#25409=ORIENTED_EDGE('',*,*,#18769,.F.);
#25410=ORIENTED_EDGE('',*,*,#18772,.F.);
#25411=ORIENTED_EDGE('',*,*,#18773,.T.);
#25412=ORIENTED_EDGE('',*,*,#18774,.T.);
#25413=ORIENTED_EDGE('',*,*,#18775,.F.);
#25414=ORIENTED_EDGE('',*,*,#18776,.F.);
#25415=ORIENTED_EDGE('',*,*,#18777,.T.);
#25416=ORIENTED_EDGE('',*,*,#18778,.T.);
#25417=ORIENTED_EDGE('',*,*,#18773,.F.);
#25418=ORIENTED_EDGE('',*,*,#18779,.F.);
#25419=ORIENTED_EDGE('',*,*,#18780,.T.);
#25420=ORIENTED_EDGE('',*,*,#18781,.T.);
#25421=ORIENTED_EDGE('',*,*,#18777,.F.);
#25422=ORIENTED_EDGE('',*,*,#18782,.F.);
#25423=ORIENTED_EDGE('',*,*,#18775,.T.);
#25424=ORIENTED_EDGE('',*,*,#18783,.T.);
#25425=ORIENTED_EDGE('',*,*,#18780,.F.);
#25426=ORIENTED_EDGE('',*,*,#18783,.F.);
#25427=ORIENTED_EDGE('',*,*,#18774,.F.);
#25428=ORIENTED_EDGE('',*,*,#18778,.F.);
#25429=ORIENTED_EDGE('',*,*,#18781,.F.);
#25430=ORIENTED_EDGE('',*,*,#18784,.F.);
#25431=ORIENTED_EDGE('',*,*,#18785,.T.);
#25432=ORIENTED_EDGE('',*,*,#18786,.T.);
#25433=ORIENTED_EDGE('',*,*,#18787,.F.);
#25434=ORIENTED_EDGE('',*,*,#18788,.F.);
#25435=ORIENTED_EDGE('',*,*,#18789,.T.);
#25436=ORIENTED_EDGE('',*,*,#18790,.T.);
#25437=ORIENTED_EDGE('',*,*,#18785,.F.);
#25438=ORIENTED_EDGE('',*,*,#18791,.F.);
#25439=ORIENTED_EDGE('',*,*,#18792,.T.);
#25440=ORIENTED_EDGE('',*,*,#18793,.T.);
#25441=ORIENTED_EDGE('',*,*,#18789,.F.);
#25442=ORIENTED_EDGE('',*,*,#18794,.F.);
#25443=ORIENTED_EDGE('',*,*,#18787,.T.);
#25444=ORIENTED_EDGE('',*,*,#18795,.T.);
#25445=ORIENTED_EDGE('',*,*,#18792,.F.);
#25446=ORIENTED_EDGE('',*,*,#18795,.F.);
#25447=ORIENTED_EDGE('',*,*,#18786,.F.);
#25448=ORIENTED_EDGE('',*,*,#18790,.F.);
#25449=ORIENTED_EDGE('',*,*,#18793,.F.);
#25450=ORIENTED_EDGE('',*,*,#18796,.F.);
#25451=ORIENTED_EDGE('',*,*,#18797,.T.);
#25452=ORIENTED_EDGE('',*,*,#18798,.T.);
#25453=ORIENTED_EDGE('',*,*,#18799,.F.);
#25454=ORIENTED_EDGE('',*,*,#18800,.F.);
#25455=ORIENTED_EDGE('',*,*,#18801,.T.);
#25456=ORIENTED_EDGE('',*,*,#18802,.T.);
#25457=ORIENTED_EDGE('',*,*,#18797,.F.);
#25458=ORIENTED_EDGE('',*,*,#18803,.F.);
#25459=ORIENTED_EDGE('',*,*,#18804,.T.);
#25460=ORIENTED_EDGE('',*,*,#18805,.T.);
#25461=ORIENTED_EDGE('',*,*,#18801,.F.);
#25462=ORIENTED_EDGE('',*,*,#18806,.F.);
#25463=ORIENTED_EDGE('',*,*,#18799,.T.);
#25464=ORIENTED_EDGE('',*,*,#18807,.T.);
#25465=ORIENTED_EDGE('',*,*,#18804,.F.);
#25466=ORIENTED_EDGE('',*,*,#18807,.F.);
#25467=ORIENTED_EDGE('',*,*,#18798,.F.);
#25468=ORIENTED_EDGE('',*,*,#18802,.F.);
#25469=ORIENTED_EDGE('',*,*,#18805,.F.);
#25470=ORIENTED_EDGE('',*,*,#18808,.F.);
#25471=ORIENTED_EDGE('',*,*,#18809,.T.);
#25472=ORIENTED_EDGE('',*,*,#18810,.T.);
#25473=ORIENTED_EDGE('',*,*,#18811,.F.);
#25474=ORIENTED_EDGE('',*,*,#18812,.F.);
#25475=ORIENTED_EDGE('',*,*,#18813,.T.);
#25476=ORIENTED_EDGE('',*,*,#18814,.T.);
#25477=ORIENTED_EDGE('',*,*,#18809,.F.);
#25478=ORIENTED_EDGE('',*,*,#18815,.F.);
#25479=ORIENTED_EDGE('',*,*,#18816,.T.);
#25480=ORIENTED_EDGE('',*,*,#18817,.T.);
#25481=ORIENTED_EDGE('',*,*,#18813,.F.);
#25482=ORIENTED_EDGE('',*,*,#18818,.F.);
#25483=ORIENTED_EDGE('',*,*,#18811,.T.);
#25484=ORIENTED_EDGE('',*,*,#18819,.T.);
#25485=ORIENTED_EDGE('',*,*,#18816,.F.);
#25486=ORIENTED_EDGE('',*,*,#18819,.F.);
#25487=ORIENTED_EDGE('',*,*,#18810,.F.);
#25488=ORIENTED_EDGE('',*,*,#18814,.F.);
#25489=ORIENTED_EDGE('',*,*,#18817,.F.);
#25490=ORIENTED_EDGE('',*,*,#18820,.F.);
#25491=ORIENTED_EDGE('',*,*,#18821,.T.);
#25492=ORIENTED_EDGE('',*,*,#18822,.T.);
#25493=ORIENTED_EDGE('',*,*,#18823,.F.);
#25494=ORIENTED_EDGE('',*,*,#18824,.F.);
#25495=ORIENTED_EDGE('',*,*,#18825,.T.);
#25496=ORIENTED_EDGE('',*,*,#18826,.T.);
#25497=ORIENTED_EDGE('',*,*,#18821,.F.);
#25498=ORIENTED_EDGE('',*,*,#18827,.F.);
#25499=ORIENTED_EDGE('',*,*,#18828,.T.);
#25500=ORIENTED_EDGE('',*,*,#18829,.T.);
#25501=ORIENTED_EDGE('',*,*,#18825,.F.);
#25502=ORIENTED_EDGE('',*,*,#18830,.F.);
#25503=ORIENTED_EDGE('',*,*,#18823,.T.);
#25504=ORIENTED_EDGE('',*,*,#18831,.T.);
#25505=ORIENTED_EDGE('',*,*,#18828,.F.);
#25506=ORIENTED_EDGE('',*,*,#18831,.F.);
#25507=ORIENTED_EDGE('',*,*,#18822,.F.);
#25508=ORIENTED_EDGE('',*,*,#18826,.F.);
#25509=ORIENTED_EDGE('',*,*,#18829,.F.);
#25510=ORIENTED_EDGE('',*,*,#18832,.F.);
#25511=ORIENTED_EDGE('',*,*,#18833,.T.);
#25512=ORIENTED_EDGE('',*,*,#18834,.T.);
#25513=ORIENTED_EDGE('',*,*,#18835,.F.);
#25514=ORIENTED_EDGE('',*,*,#18836,.F.);
#25515=ORIENTED_EDGE('',*,*,#18837,.T.);
#25516=ORIENTED_EDGE('',*,*,#18838,.T.);
#25517=ORIENTED_EDGE('',*,*,#18833,.F.);
#25518=ORIENTED_EDGE('',*,*,#18839,.F.);
#25519=ORIENTED_EDGE('',*,*,#18840,.T.);
#25520=ORIENTED_EDGE('',*,*,#18841,.T.);
#25521=ORIENTED_EDGE('',*,*,#18837,.F.);
#25522=ORIENTED_EDGE('',*,*,#18842,.F.);
#25523=ORIENTED_EDGE('',*,*,#18835,.T.);
#25524=ORIENTED_EDGE('',*,*,#18843,.T.);
#25525=ORIENTED_EDGE('',*,*,#18840,.F.);
#25526=ORIENTED_EDGE('',*,*,#18843,.F.);
#25527=ORIENTED_EDGE('',*,*,#18834,.F.);
#25528=ORIENTED_EDGE('',*,*,#18838,.F.);
#25529=ORIENTED_EDGE('',*,*,#18841,.F.);
#25530=ORIENTED_EDGE('',*,*,#18844,.F.);
#25531=ORIENTED_EDGE('',*,*,#18845,.T.);
#25532=ORIENTED_EDGE('',*,*,#18846,.T.);
#25533=ORIENTED_EDGE('',*,*,#18847,.F.);
#25534=ORIENTED_EDGE('',*,*,#18848,.F.);
#25535=ORIENTED_EDGE('',*,*,#18849,.T.);
#25536=ORIENTED_EDGE('',*,*,#18850,.T.);
#25537=ORIENTED_EDGE('',*,*,#18845,.F.);
#25538=ORIENTED_EDGE('',*,*,#18851,.F.);
#25539=ORIENTED_EDGE('',*,*,#18852,.T.);
#25540=ORIENTED_EDGE('',*,*,#18853,.T.);
#25541=ORIENTED_EDGE('',*,*,#18849,.F.);
#25542=ORIENTED_EDGE('',*,*,#18854,.F.);
#25543=ORIENTED_EDGE('',*,*,#18847,.T.);
#25544=ORIENTED_EDGE('',*,*,#18855,.T.);
#25545=ORIENTED_EDGE('',*,*,#18852,.F.);
#25546=ORIENTED_EDGE('',*,*,#18855,.F.);
#25547=ORIENTED_EDGE('',*,*,#18846,.F.);
#25548=ORIENTED_EDGE('',*,*,#18850,.F.);
#25549=ORIENTED_EDGE('',*,*,#18853,.F.);
#25550=ORIENTED_EDGE('',*,*,#18856,.F.);
#25551=ORIENTED_EDGE('',*,*,#18857,.T.);
#25552=ORIENTED_EDGE('',*,*,#18858,.T.);
#25553=ORIENTED_EDGE('',*,*,#18859,.F.);
#25554=ORIENTED_EDGE('',*,*,#18860,.F.);
#25555=ORIENTED_EDGE('',*,*,#18861,.T.);
#25556=ORIENTED_EDGE('',*,*,#18862,.T.);
#25557=ORIENTED_EDGE('',*,*,#18857,.F.);
#25558=ORIENTED_EDGE('',*,*,#18863,.F.);
#25559=ORIENTED_EDGE('',*,*,#18864,.T.);
#25560=ORIENTED_EDGE('',*,*,#18865,.T.);
#25561=ORIENTED_EDGE('',*,*,#18861,.F.);
#25562=ORIENTED_EDGE('',*,*,#18866,.F.);
#25563=ORIENTED_EDGE('',*,*,#18859,.T.);
#25564=ORIENTED_EDGE('',*,*,#18867,.T.);
#25565=ORIENTED_EDGE('',*,*,#18864,.F.);
#25566=ORIENTED_EDGE('',*,*,#18867,.F.);
#25567=ORIENTED_EDGE('',*,*,#18858,.F.);
#25568=ORIENTED_EDGE('',*,*,#18862,.F.);
#25569=ORIENTED_EDGE('',*,*,#18865,.F.);
#25570=ORIENTED_EDGE('',*,*,#18868,.F.);
#25571=ORIENTED_EDGE('',*,*,#18869,.T.);
#25572=ORIENTED_EDGE('',*,*,#18870,.T.);
#25573=ORIENTED_EDGE('',*,*,#18871,.F.);
#25574=ORIENTED_EDGE('',*,*,#18872,.F.);
#25575=ORIENTED_EDGE('',*,*,#18873,.T.);
#25576=ORIENTED_EDGE('',*,*,#18874,.T.);
#25577=ORIENTED_EDGE('',*,*,#18869,.F.);
#25578=ORIENTED_EDGE('',*,*,#18875,.F.);
#25579=ORIENTED_EDGE('',*,*,#18876,.T.);
#25580=ORIENTED_EDGE('',*,*,#18877,.T.);
#25581=ORIENTED_EDGE('',*,*,#18873,.F.);
#25582=ORIENTED_EDGE('',*,*,#18878,.F.);
#25583=ORIENTED_EDGE('',*,*,#18871,.T.);
#25584=ORIENTED_EDGE('',*,*,#18879,.T.);
#25585=ORIENTED_EDGE('',*,*,#18876,.F.);
#25586=ORIENTED_EDGE('',*,*,#18879,.F.);
#25587=ORIENTED_EDGE('',*,*,#18870,.F.);
#25588=ORIENTED_EDGE('',*,*,#18874,.F.);
#25589=ORIENTED_EDGE('',*,*,#18877,.F.);
#25590=ORIENTED_EDGE('',*,*,#18880,.F.);
#25591=ORIENTED_EDGE('',*,*,#18881,.T.);
#25592=ORIENTED_EDGE('',*,*,#18882,.T.);
#25593=ORIENTED_EDGE('',*,*,#18883,.F.);
#25594=ORIENTED_EDGE('',*,*,#18884,.F.);
#25595=ORIENTED_EDGE('',*,*,#18885,.T.);
#25596=ORIENTED_EDGE('',*,*,#18886,.T.);
#25597=ORIENTED_EDGE('',*,*,#18881,.F.);
#25598=ORIENTED_EDGE('',*,*,#18887,.F.);
#25599=ORIENTED_EDGE('',*,*,#18888,.T.);
#25600=ORIENTED_EDGE('',*,*,#18889,.T.);
#25601=ORIENTED_EDGE('',*,*,#18885,.F.);
#25602=ORIENTED_EDGE('',*,*,#18890,.F.);
#25603=ORIENTED_EDGE('',*,*,#18883,.T.);
#25604=ORIENTED_EDGE('',*,*,#18891,.T.);
#25605=ORIENTED_EDGE('',*,*,#18888,.F.);
#25606=ORIENTED_EDGE('',*,*,#18891,.F.);
#25607=ORIENTED_EDGE('',*,*,#18882,.F.);
#25608=ORIENTED_EDGE('',*,*,#18886,.F.);
#25609=ORIENTED_EDGE('',*,*,#18889,.F.);
#25610=ORIENTED_EDGE('',*,*,#18892,.F.);
#25611=ORIENTED_EDGE('',*,*,#18893,.T.);
#25612=ORIENTED_EDGE('',*,*,#18894,.T.);
#25613=ORIENTED_EDGE('',*,*,#18895,.F.);
#25614=ORIENTED_EDGE('',*,*,#18896,.F.);
#25615=ORIENTED_EDGE('',*,*,#18897,.T.);
#25616=ORIENTED_EDGE('',*,*,#18898,.T.);
#25617=ORIENTED_EDGE('',*,*,#18893,.F.);
#25618=ORIENTED_EDGE('',*,*,#18899,.F.);
#25619=ORIENTED_EDGE('',*,*,#18900,.T.);
#25620=ORIENTED_EDGE('',*,*,#18901,.T.);
#25621=ORIENTED_EDGE('',*,*,#18897,.F.);
#25622=ORIENTED_EDGE('',*,*,#18902,.F.);
#25623=ORIENTED_EDGE('',*,*,#18895,.T.);
#25624=ORIENTED_EDGE('',*,*,#18903,.T.);
#25625=ORIENTED_EDGE('',*,*,#18900,.F.);
#25626=ORIENTED_EDGE('',*,*,#18903,.F.);
#25627=ORIENTED_EDGE('',*,*,#18894,.F.);
#25628=ORIENTED_EDGE('',*,*,#18898,.F.);
#25629=ORIENTED_EDGE('',*,*,#18901,.F.);
#25630=ORIENTED_EDGE('',*,*,#18904,.F.);
#25631=ORIENTED_EDGE('',*,*,#18905,.T.);
#25632=ORIENTED_EDGE('',*,*,#18906,.T.);
#25633=ORIENTED_EDGE('',*,*,#18907,.F.);
#25634=ORIENTED_EDGE('',*,*,#18908,.F.);
#25635=ORIENTED_EDGE('',*,*,#18909,.T.);
#25636=ORIENTED_EDGE('',*,*,#18910,.T.);
#25637=ORIENTED_EDGE('',*,*,#18905,.F.);
#25638=ORIENTED_EDGE('',*,*,#18911,.F.);
#25639=ORIENTED_EDGE('',*,*,#18912,.T.);
#25640=ORIENTED_EDGE('',*,*,#18913,.T.);
#25641=ORIENTED_EDGE('',*,*,#18909,.F.);
#25642=ORIENTED_EDGE('',*,*,#18914,.F.);
#25643=ORIENTED_EDGE('',*,*,#18907,.T.);
#25644=ORIENTED_EDGE('',*,*,#18915,.T.);
#25645=ORIENTED_EDGE('',*,*,#18912,.F.);
#25646=ORIENTED_EDGE('',*,*,#18915,.F.);
#25647=ORIENTED_EDGE('',*,*,#18906,.F.);
#25648=ORIENTED_EDGE('',*,*,#18910,.F.);
#25649=ORIENTED_EDGE('',*,*,#18913,.F.);
#25650=ORIENTED_EDGE('',*,*,#18916,.F.);
#25651=ORIENTED_EDGE('',*,*,#18917,.T.);
#25652=ORIENTED_EDGE('',*,*,#18918,.T.);
#25653=ORIENTED_EDGE('',*,*,#18919,.F.);
#25654=ORIENTED_EDGE('',*,*,#18920,.F.);
#25655=ORIENTED_EDGE('',*,*,#18921,.T.);
#25656=ORIENTED_EDGE('',*,*,#18922,.T.);
#25657=ORIENTED_EDGE('',*,*,#18917,.F.);
#25658=ORIENTED_EDGE('',*,*,#18923,.F.);
#25659=ORIENTED_EDGE('',*,*,#18924,.T.);
#25660=ORIENTED_EDGE('',*,*,#18925,.T.);
#25661=ORIENTED_EDGE('',*,*,#18921,.F.);
#25662=ORIENTED_EDGE('',*,*,#18926,.F.);
#25663=ORIENTED_EDGE('',*,*,#18919,.T.);
#25664=ORIENTED_EDGE('',*,*,#18927,.T.);
#25665=ORIENTED_EDGE('',*,*,#18924,.F.);
#25666=ORIENTED_EDGE('',*,*,#18927,.F.);
#25667=ORIENTED_EDGE('',*,*,#18918,.F.);
#25668=ORIENTED_EDGE('',*,*,#18922,.F.);
#25669=ORIENTED_EDGE('',*,*,#18925,.F.);
#25670=ORIENTED_EDGE('',*,*,#18928,.F.);
#25671=ORIENTED_EDGE('',*,*,#18929,.T.);
#25672=ORIENTED_EDGE('',*,*,#18930,.T.);
#25673=ORIENTED_EDGE('',*,*,#18931,.F.);
#25674=ORIENTED_EDGE('',*,*,#18932,.F.);
#25675=ORIENTED_EDGE('',*,*,#18933,.T.);
#25676=ORIENTED_EDGE('',*,*,#18934,.T.);
#25677=ORIENTED_EDGE('',*,*,#18929,.F.);
#25678=ORIENTED_EDGE('',*,*,#18935,.F.);
#25679=ORIENTED_EDGE('',*,*,#18936,.T.);
#25680=ORIENTED_EDGE('',*,*,#18937,.T.);
#25681=ORIENTED_EDGE('',*,*,#18933,.F.);
#25682=ORIENTED_EDGE('',*,*,#18938,.F.);
#25683=ORIENTED_EDGE('',*,*,#18931,.T.);
#25684=ORIENTED_EDGE('',*,*,#18939,.T.);
#25685=ORIENTED_EDGE('',*,*,#18936,.F.);
#25686=ORIENTED_EDGE('',*,*,#18939,.F.);
#25687=ORIENTED_EDGE('',*,*,#18930,.F.);
#25688=ORIENTED_EDGE('',*,*,#18934,.F.);
#25689=ORIENTED_EDGE('',*,*,#18937,.F.);
#25690=ORIENTED_EDGE('',*,*,#18940,.F.);
#25691=ORIENTED_EDGE('',*,*,#18941,.T.);
#25692=ORIENTED_EDGE('',*,*,#18942,.T.);
#25693=ORIENTED_EDGE('',*,*,#18943,.F.);
#25694=ORIENTED_EDGE('',*,*,#18944,.F.);
#25695=ORIENTED_EDGE('',*,*,#18945,.T.);
#25696=ORIENTED_EDGE('',*,*,#18946,.T.);
#25697=ORIENTED_EDGE('',*,*,#18941,.F.);
#25698=ORIENTED_EDGE('',*,*,#18947,.F.);
#25699=ORIENTED_EDGE('',*,*,#18948,.T.);
#25700=ORIENTED_EDGE('',*,*,#18949,.T.);
#25701=ORIENTED_EDGE('',*,*,#18945,.F.);
#25702=ORIENTED_EDGE('',*,*,#18950,.F.);
#25703=ORIENTED_EDGE('',*,*,#18943,.T.);
#25704=ORIENTED_EDGE('',*,*,#18951,.T.);
#25705=ORIENTED_EDGE('',*,*,#18948,.F.);
#25706=ORIENTED_EDGE('',*,*,#18951,.F.);
#25707=ORIENTED_EDGE('',*,*,#18942,.F.);
#25708=ORIENTED_EDGE('',*,*,#18946,.F.);
#25709=ORIENTED_EDGE('',*,*,#18949,.F.);
#25710=ORIENTED_EDGE('',*,*,#18952,.F.);
#25711=ORIENTED_EDGE('',*,*,#18953,.T.);
#25712=ORIENTED_EDGE('',*,*,#18954,.T.);
#25713=ORIENTED_EDGE('',*,*,#18955,.F.);
#25714=ORIENTED_EDGE('',*,*,#18956,.F.);
#25715=ORIENTED_EDGE('',*,*,#18957,.T.);
#25716=ORIENTED_EDGE('',*,*,#18958,.T.);
#25717=ORIENTED_EDGE('',*,*,#18953,.F.);
#25718=ORIENTED_EDGE('',*,*,#18959,.F.);
#25719=ORIENTED_EDGE('',*,*,#18960,.T.);
#25720=ORIENTED_EDGE('',*,*,#18961,.T.);
#25721=ORIENTED_EDGE('',*,*,#18957,.F.);
#25722=ORIENTED_EDGE('',*,*,#18962,.F.);
#25723=ORIENTED_EDGE('',*,*,#18955,.T.);
#25724=ORIENTED_EDGE('',*,*,#18963,.T.);
#25725=ORIENTED_EDGE('',*,*,#18960,.F.);
#25726=ORIENTED_EDGE('',*,*,#18963,.F.);
#25727=ORIENTED_EDGE('',*,*,#18954,.F.);
#25728=ORIENTED_EDGE('',*,*,#18958,.F.);
#25729=ORIENTED_EDGE('',*,*,#18961,.F.);
#25730=ORIENTED_EDGE('',*,*,#18964,.F.);
#25731=ORIENTED_EDGE('',*,*,#18965,.T.);
#25732=ORIENTED_EDGE('',*,*,#18966,.T.);
#25733=ORIENTED_EDGE('',*,*,#18967,.F.);
#25734=ORIENTED_EDGE('',*,*,#18968,.F.);
#25735=ORIENTED_EDGE('',*,*,#18969,.T.);
#25736=ORIENTED_EDGE('',*,*,#18970,.T.);
#25737=ORIENTED_EDGE('',*,*,#18965,.F.);
#25738=ORIENTED_EDGE('',*,*,#18971,.F.);
#25739=ORIENTED_EDGE('',*,*,#18972,.T.);
#25740=ORIENTED_EDGE('',*,*,#18973,.T.);
#25741=ORIENTED_EDGE('',*,*,#18969,.F.);
#25742=ORIENTED_EDGE('',*,*,#18974,.F.);
#25743=ORIENTED_EDGE('',*,*,#18967,.T.);
#25744=ORIENTED_EDGE('',*,*,#18975,.T.);
#25745=ORIENTED_EDGE('',*,*,#18972,.F.);
#25746=ORIENTED_EDGE('',*,*,#18975,.F.);
#25747=ORIENTED_EDGE('',*,*,#18966,.F.);
#25748=ORIENTED_EDGE('',*,*,#18970,.F.);
#25749=ORIENTED_EDGE('',*,*,#18973,.F.);
#25750=ORIENTED_EDGE('',*,*,#18976,.F.);
#25751=ORIENTED_EDGE('',*,*,#18977,.T.);
#25752=ORIENTED_EDGE('',*,*,#18978,.T.);
#25753=ORIENTED_EDGE('',*,*,#18979,.F.);
#25754=ORIENTED_EDGE('',*,*,#18980,.F.);
#25755=ORIENTED_EDGE('',*,*,#18981,.T.);
#25756=ORIENTED_EDGE('',*,*,#18982,.T.);
#25757=ORIENTED_EDGE('',*,*,#18977,.F.);
#25758=ORIENTED_EDGE('',*,*,#18983,.F.);
#25759=ORIENTED_EDGE('',*,*,#18984,.T.);
#25760=ORIENTED_EDGE('',*,*,#18985,.T.);
#25761=ORIENTED_EDGE('',*,*,#18981,.F.);
#25762=ORIENTED_EDGE('',*,*,#18986,.F.);
#25763=ORIENTED_EDGE('',*,*,#18979,.T.);
#25764=ORIENTED_EDGE('',*,*,#18987,.T.);
#25765=ORIENTED_EDGE('',*,*,#18984,.F.);
#25766=ORIENTED_EDGE('',*,*,#18987,.F.);
#25767=ORIENTED_EDGE('',*,*,#18978,.F.);
#25768=ORIENTED_EDGE('',*,*,#18982,.F.);
#25769=ORIENTED_EDGE('',*,*,#18985,.F.);
#25770=ORIENTED_EDGE('',*,*,#18988,.F.);
#25771=ORIENTED_EDGE('',*,*,#18989,.T.);
#25772=ORIENTED_EDGE('',*,*,#18990,.T.);
#25773=ORIENTED_EDGE('',*,*,#18991,.F.);
#25774=ORIENTED_EDGE('',*,*,#18992,.F.);
#25775=ORIENTED_EDGE('',*,*,#18993,.T.);
#25776=ORIENTED_EDGE('',*,*,#18994,.T.);
#25777=ORIENTED_EDGE('',*,*,#18989,.F.);
#25778=ORIENTED_EDGE('',*,*,#18995,.F.);
#25779=ORIENTED_EDGE('',*,*,#18996,.T.);
#25780=ORIENTED_EDGE('',*,*,#18997,.T.);
#25781=ORIENTED_EDGE('',*,*,#18993,.F.);
#25782=ORIENTED_EDGE('',*,*,#18998,.F.);
#25783=ORIENTED_EDGE('',*,*,#18991,.T.);
#25784=ORIENTED_EDGE('',*,*,#18999,.T.);
#25785=ORIENTED_EDGE('',*,*,#18996,.F.);
#25786=ORIENTED_EDGE('',*,*,#18999,.F.);
#25787=ORIENTED_EDGE('',*,*,#18990,.F.);
#25788=ORIENTED_EDGE('',*,*,#18994,.F.);
#25789=ORIENTED_EDGE('',*,*,#18997,.F.);
#25790=ORIENTED_EDGE('',*,*,#19000,.F.);
#25791=ORIENTED_EDGE('',*,*,#19001,.T.);
#25792=ORIENTED_EDGE('',*,*,#19002,.T.);
#25793=ORIENTED_EDGE('',*,*,#19003,.F.);
#25794=ORIENTED_EDGE('',*,*,#19004,.F.);
#25795=ORIENTED_EDGE('',*,*,#19005,.T.);
#25796=ORIENTED_EDGE('',*,*,#19006,.T.);
#25797=ORIENTED_EDGE('',*,*,#19001,.F.);
#25798=ORIENTED_EDGE('',*,*,#19007,.F.);
#25799=ORIENTED_EDGE('',*,*,#19008,.T.);
#25800=ORIENTED_EDGE('',*,*,#19009,.T.);
#25801=ORIENTED_EDGE('',*,*,#19005,.F.);
#25802=ORIENTED_EDGE('',*,*,#19010,.F.);
#25803=ORIENTED_EDGE('',*,*,#19003,.T.);
#25804=ORIENTED_EDGE('',*,*,#19011,.T.);
#25805=ORIENTED_EDGE('',*,*,#19008,.F.);
#25806=ORIENTED_EDGE('',*,*,#19011,.F.);
#25807=ORIENTED_EDGE('',*,*,#19002,.F.);
#25808=ORIENTED_EDGE('',*,*,#19006,.F.);
#25809=ORIENTED_EDGE('',*,*,#19009,.F.);
#25810=ORIENTED_EDGE('',*,*,#19012,.F.);
#25811=ORIENTED_EDGE('',*,*,#19013,.T.);
#25812=ORIENTED_EDGE('',*,*,#19014,.T.);
#25813=ORIENTED_EDGE('',*,*,#19015,.F.);
#25814=ORIENTED_EDGE('',*,*,#19016,.F.);
#25815=ORIENTED_EDGE('',*,*,#19017,.T.);
#25816=ORIENTED_EDGE('',*,*,#19018,.T.);
#25817=ORIENTED_EDGE('',*,*,#19013,.F.);
#25818=ORIENTED_EDGE('',*,*,#19019,.F.);
#25819=ORIENTED_EDGE('',*,*,#19020,.T.);
#25820=ORIENTED_EDGE('',*,*,#19021,.T.);
#25821=ORIENTED_EDGE('',*,*,#19017,.F.);
#25822=ORIENTED_EDGE('',*,*,#19022,.F.);
#25823=ORIENTED_EDGE('',*,*,#19015,.T.);
#25824=ORIENTED_EDGE('',*,*,#19023,.T.);
#25825=ORIENTED_EDGE('',*,*,#19020,.F.);
#25826=ORIENTED_EDGE('',*,*,#19023,.F.);
#25827=ORIENTED_EDGE('',*,*,#19014,.F.);
#25828=ORIENTED_EDGE('',*,*,#19018,.F.);
#25829=ORIENTED_EDGE('',*,*,#19021,.F.);
#25830=ORIENTED_EDGE('',*,*,#19024,.F.);
#25831=ORIENTED_EDGE('',*,*,#19025,.T.);
#25832=ORIENTED_EDGE('',*,*,#19026,.T.);
#25833=ORIENTED_EDGE('',*,*,#19027,.F.);
#25834=ORIENTED_EDGE('',*,*,#19028,.F.);
#25835=ORIENTED_EDGE('',*,*,#19029,.T.);
#25836=ORIENTED_EDGE('',*,*,#19030,.T.);
#25837=ORIENTED_EDGE('',*,*,#19025,.F.);
#25838=ORIENTED_EDGE('',*,*,#19031,.F.);
#25839=ORIENTED_EDGE('',*,*,#19032,.T.);
#25840=ORIENTED_EDGE('',*,*,#19033,.T.);
#25841=ORIENTED_EDGE('',*,*,#19029,.F.);
#25842=ORIENTED_EDGE('',*,*,#19034,.F.);
#25843=ORIENTED_EDGE('',*,*,#19027,.T.);
#25844=ORIENTED_EDGE('',*,*,#19035,.T.);
#25845=ORIENTED_EDGE('',*,*,#19032,.F.);
#25846=ORIENTED_EDGE('',*,*,#19035,.F.);
#25847=ORIENTED_EDGE('',*,*,#19026,.F.);
#25848=ORIENTED_EDGE('',*,*,#19030,.F.);
#25849=ORIENTED_EDGE('',*,*,#19033,.F.);
#25850=ORIENTED_EDGE('',*,*,#19036,.F.);
#25851=ORIENTED_EDGE('',*,*,#19037,.T.);
#25852=ORIENTED_EDGE('',*,*,#19038,.T.);
#25853=ORIENTED_EDGE('',*,*,#19039,.F.);
#25854=ORIENTED_EDGE('',*,*,#19040,.F.);
#25855=ORIENTED_EDGE('',*,*,#19041,.T.);
#25856=ORIENTED_EDGE('',*,*,#19042,.T.);
#25857=ORIENTED_EDGE('',*,*,#19037,.F.);
#25858=ORIENTED_EDGE('',*,*,#19043,.F.);
#25859=ORIENTED_EDGE('',*,*,#19044,.T.);
#25860=ORIENTED_EDGE('',*,*,#19045,.T.);
#25861=ORIENTED_EDGE('',*,*,#19041,.F.);
#25862=ORIENTED_EDGE('',*,*,#19046,.F.);
#25863=ORIENTED_EDGE('',*,*,#19039,.T.);
#25864=ORIENTED_EDGE('',*,*,#19047,.T.);
#25865=ORIENTED_EDGE('',*,*,#19044,.F.);
#25866=ORIENTED_EDGE('',*,*,#19047,.F.);
#25867=ORIENTED_EDGE('',*,*,#19038,.F.);
#25868=ORIENTED_EDGE('',*,*,#19042,.F.);
#25869=ORIENTED_EDGE('',*,*,#19045,.F.);
#25870=ORIENTED_EDGE('',*,*,#19048,.F.);
#25871=ORIENTED_EDGE('',*,*,#19049,.T.);
#25872=ORIENTED_EDGE('',*,*,#19050,.T.);
#25873=ORIENTED_EDGE('',*,*,#19051,.F.);
#25874=ORIENTED_EDGE('',*,*,#19052,.F.);
#25875=ORIENTED_EDGE('',*,*,#19053,.T.);
#25876=ORIENTED_EDGE('',*,*,#19054,.T.);
#25877=ORIENTED_EDGE('',*,*,#19049,.F.);
#25878=ORIENTED_EDGE('',*,*,#19055,.F.);
#25879=ORIENTED_EDGE('',*,*,#19056,.T.);
#25880=ORIENTED_EDGE('',*,*,#19057,.T.);
#25881=ORIENTED_EDGE('',*,*,#19053,.F.);
#25882=ORIENTED_EDGE('',*,*,#19058,.F.);
#25883=ORIENTED_EDGE('',*,*,#19051,.T.);
#25884=ORIENTED_EDGE('',*,*,#19059,.T.);
#25885=ORIENTED_EDGE('',*,*,#19056,.F.);
#25886=ORIENTED_EDGE('',*,*,#19059,.F.);
#25887=ORIENTED_EDGE('',*,*,#19050,.F.);
#25888=ORIENTED_EDGE('',*,*,#19054,.F.);
#25889=ORIENTED_EDGE('',*,*,#19057,.F.);
#25890=ORIENTED_EDGE('',*,*,#19060,.F.);
#25891=ORIENTED_EDGE('',*,*,#19061,.T.);
#25892=ORIENTED_EDGE('',*,*,#19062,.T.);
#25893=ORIENTED_EDGE('',*,*,#19063,.F.);
#25894=ORIENTED_EDGE('',*,*,#19064,.F.);
#25895=ORIENTED_EDGE('',*,*,#19065,.T.);
#25896=ORIENTED_EDGE('',*,*,#19066,.T.);
#25897=ORIENTED_EDGE('',*,*,#19061,.F.);
#25898=ORIENTED_EDGE('',*,*,#19067,.F.);
#25899=ORIENTED_EDGE('',*,*,#19068,.T.);
#25900=ORIENTED_EDGE('',*,*,#19069,.T.);
#25901=ORIENTED_EDGE('',*,*,#19065,.F.);
#25902=ORIENTED_EDGE('',*,*,#19070,.F.);
#25903=ORIENTED_EDGE('',*,*,#19063,.T.);
#25904=ORIENTED_EDGE('',*,*,#19071,.T.);
#25905=ORIENTED_EDGE('',*,*,#19068,.F.);
#25906=ORIENTED_EDGE('',*,*,#19071,.F.);
#25907=ORIENTED_EDGE('',*,*,#19062,.F.);
#25908=ORIENTED_EDGE('',*,*,#19066,.F.);
#25909=ORIENTED_EDGE('',*,*,#19069,.F.);
#25910=ORIENTED_EDGE('',*,*,#19072,.F.);
#25911=ORIENTED_EDGE('',*,*,#19073,.T.);
#25912=ORIENTED_EDGE('',*,*,#19074,.T.);
#25913=ORIENTED_EDGE('',*,*,#19075,.F.);
#25914=ORIENTED_EDGE('',*,*,#19076,.F.);
#25915=ORIENTED_EDGE('',*,*,#19077,.T.);
#25916=ORIENTED_EDGE('',*,*,#19078,.T.);
#25917=ORIENTED_EDGE('',*,*,#19073,.F.);
#25918=ORIENTED_EDGE('',*,*,#19079,.F.);
#25919=ORIENTED_EDGE('',*,*,#19080,.T.);
#25920=ORIENTED_EDGE('',*,*,#19081,.T.);
#25921=ORIENTED_EDGE('',*,*,#19077,.F.);
#25922=ORIENTED_EDGE('',*,*,#19082,.F.);
#25923=ORIENTED_EDGE('',*,*,#19075,.T.);
#25924=ORIENTED_EDGE('',*,*,#19083,.T.);
#25925=ORIENTED_EDGE('',*,*,#19080,.F.);
#25926=ORIENTED_EDGE('',*,*,#19083,.F.);
#25927=ORIENTED_EDGE('',*,*,#19074,.F.);
#25928=ORIENTED_EDGE('',*,*,#19078,.F.);
#25929=ORIENTED_EDGE('',*,*,#19081,.F.);
#25930=ORIENTED_EDGE('',*,*,#19084,.F.);
#25931=ORIENTED_EDGE('',*,*,#19085,.T.);
#25932=ORIENTED_EDGE('',*,*,#19086,.T.);
#25933=ORIENTED_EDGE('',*,*,#19087,.F.);
#25934=ORIENTED_EDGE('',*,*,#19088,.F.);
#25935=ORIENTED_EDGE('',*,*,#19089,.T.);
#25936=ORIENTED_EDGE('',*,*,#19090,.T.);
#25937=ORIENTED_EDGE('',*,*,#19085,.F.);
#25938=ORIENTED_EDGE('',*,*,#19091,.F.);
#25939=ORIENTED_EDGE('',*,*,#19092,.T.);
#25940=ORIENTED_EDGE('',*,*,#19093,.T.);
#25941=ORIENTED_EDGE('',*,*,#19089,.F.);
#25942=ORIENTED_EDGE('',*,*,#19094,.F.);
#25943=ORIENTED_EDGE('',*,*,#19087,.T.);
#25944=ORIENTED_EDGE('',*,*,#19095,.T.);
#25945=ORIENTED_EDGE('',*,*,#19092,.F.);
#25946=ORIENTED_EDGE('',*,*,#19095,.F.);
#25947=ORIENTED_EDGE('',*,*,#19086,.F.);
#25948=ORIENTED_EDGE('',*,*,#19090,.F.);
#25949=ORIENTED_EDGE('',*,*,#19093,.F.);
#25950=ORIENTED_EDGE('',*,*,#19096,.F.);
#25951=ORIENTED_EDGE('',*,*,#19097,.T.);
#25952=ORIENTED_EDGE('',*,*,#19098,.T.);
#25953=ORIENTED_EDGE('',*,*,#19099,.F.);
#25954=ORIENTED_EDGE('',*,*,#19100,.F.);
#25955=ORIENTED_EDGE('',*,*,#19101,.T.);
#25956=ORIENTED_EDGE('',*,*,#19102,.T.);
#25957=ORIENTED_EDGE('',*,*,#19097,.F.);
#25958=ORIENTED_EDGE('',*,*,#19103,.F.);
#25959=ORIENTED_EDGE('',*,*,#19104,.T.);
#25960=ORIENTED_EDGE('',*,*,#19105,.T.);
#25961=ORIENTED_EDGE('',*,*,#19101,.F.);
#25962=ORIENTED_EDGE('',*,*,#19106,.F.);
#25963=ORIENTED_EDGE('',*,*,#19099,.T.);
#25964=ORIENTED_EDGE('',*,*,#19107,.T.);
#25965=ORIENTED_EDGE('',*,*,#19104,.F.);
#25966=ORIENTED_EDGE('',*,*,#19107,.F.);
#25967=ORIENTED_EDGE('',*,*,#19098,.F.);
#25968=ORIENTED_EDGE('',*,*,#19102,.F.);
#25969=ORIENTED_EDGE('',*,*,#19105,.F.);
#25970=ORIENTED_EDGE('',*,*,#19108,.F.);
#25971=ORIENTED_EDGE('',*,*,#19109,.T.);
#25972=ORIENTED_EDGE('',*,*,#19110,.T.);
#25973=ORIENTED_EDGE('',*,*,#19111,.F.);
#25974=ORIENTED_EDGE('',*,*,#19112,.F.);
#25975=ORIENTED_EDGE('',*,*,#19113,.T.);
#25976=ORIENTED_EDGE('',*,*,#19114,.T.);
#25977=ORIENTED_EDGE('',*,*,#19109,.F.);
#25978=ORIENTED_EDGE('',*,*,#19115,.F.);
#25979=ORIENTED_EDGE('',*,*,#19116,.T.);
#25980=ORIENTED_EDGE('',*,*,#19117,.T.);
#25981=ORIENTED_EDGE('',*,*,#19113,.F.);
#25982=ORIENTED_EDGE('',*,*,#19118,.F.);
#25983=ORIENTED_EDGE('',*,*,#19111,.T.);
#25984=ORIENTED_EDGE('',*,*,#19119,.T.);
#25985=ORIENTED_EDGE('',*,*,#19116,.F.);
#25986=ORIENTED_EDGE('',*,*,#19119,.F.);
#25987=ORIENTED_EDGE('',*,*,#19110,.F.);
#25988=ORIENTED_EDGE('',*,*,#19114,.F.);
#25989=ORIENTED_EDGE('',*,*,#19117,.F.);
#25990=ORIENTED_EDGE('',*,*,#19120,.F.);
#25991=ORIENTED_EDGE('',*,*,#19121,.T.);
#25992=ORIENTED_EDGE('',*,*,#19122,.T.);
#25993=ORIENTED_EDGE('',*,*,#19123,.F.);
#25994=ORIENTED_EDGE('',*,*,#19124,.F.);
#25995=ORIENTED_EDGE('',*,*,#19125,.T.);
#25996=ORIENTED_EDGE('',*,*,#19126,.T.);
#25997=ORIENTED_EDGE('',*,*,#19121,.F.);
#25998=ORIENTED_EDGE('',*,*,#19127,.F.);
#25999=ORIENTED_EDGE('',*,*,#19128,.T.);
#26000=ORIENTED_EDGE('',*,*,#19129,.T.);
#26001=ORIENTED_EDGE('',*,*,#19125,.F.);
#26002=ORIENTED_EDGE('',*,*,#19130,.F.);
#26003=ORIENTED_EDGE('',*,*,#19123,.T.);
#26004=ORIENTED_EDGE('',*,*,#19131,.T.);
#26005=ORIENTED_EDGE('',*,*,#19128,.F.);
#26006=ORIENTED_EDGE('',*,*,#19131,.F.);
#26007=ORIENTED_EDGE('',*,*,#19122,.F.);
#26008=ORIENTED_EDGE('',*,*,#19126,.F.);
#26009=ORIENTED_EDGE('',*,*,#19129,.F.);
#26010=ORIENTED_EDGE('',*,*,#19132,.F.);
#26011=ORIENTED_EDGE('',*,*,#19133,.T.);
#26012=ORIENTED_EDGE('',*,*,#19134,.T.);
#26013=ORIENTED_EDGE('',*,*,#19135,.F.);
#26014=ORIENTED_EDGE('',*,*,#19136,.F.);
#26015=ORIENTED_EDGE('',*,*,#19137,.T.);
#26016=ORIENTED_EDGE('',*,*,#19138,.T.);
#26017=ORIENTED_EDGE('',*,*,#19133,.F.);
#26018=ORIENTED_EDGE('',*,*,#19139,.F.);
#26019=ORIENTED_EDGE('',*,*,#19140,.T.);
#26020=ORIENTED_EDGE('',*,*,#19141,.T.);
#26021=ORIENTED_EDGE('',*,*,#19137,.F.);
#26022=ORIENTED_EDGE('',*,*,#19142,.F.);
#26023=ORIENTED_EDGE('',*,*,#19135,.T.);
#26024=ORIENTED_EDGE('',*,*,#19143,.T.);
#26025=ORIENTED_EDGE('',*,*,#19140,.F.);
#26026=ORIENTED_EDGE('',*,*,#19143,.F.);
#26027=ORIENTED_EDGE('',*,*,#19134,.F.);
#26028=ORIENTED_EDGE('',*,*,#19138,.F.);
#26029=ORIENTED_EDGE('',*,*,#19141,.F.);
#26030=ORIENTED_EDGE('',*,*,#19144,.F.);
#26031=ORIENTED_EDGE('',*,*,#19145,.T.);
#26032=ORIENTED_EDGE('',*,*,#19146,.T.);
#26033=ORIENTED_EDGE('',*,*,#19147,.F.);
#26034=ORIENTED_EDGE('',*,*,#19148,.F.);
#26035=ORIENTED_EDGE('',*,*,#19149,.T.);
#26036=ORIENTED_EDGE('',*,*,#19150,.T.);
#26037=ORIENTED_EDGE('',*,*,#19145,.F.);
#26038=ORIENTED_EDGE('',*,*,#19151,.F.);
#26039=ORIENTED_EDGE('',*,*,#19152,.T.);
#26040=ORIENTED_EDGE('',*,*,#19153,.T.);
#26041=ORIENTED_EDGE('',*,*,#19149,.F.);
#26042=ORIENTED_EDGE('',*,*,#19154,.F.);
#26043=ORIENTED_EDGE('',*,*,#19147,.T.);
#26044=ORIENTED_EDGE('',*,*,#19155,.T.);
#26045=ORIENTED_EDGE('',*,*,#19152,.F.);
#26046=ORIENTED_EDGE('',*,*,#19155,.F.);
#26047=ORIENTED_EDGE('',*,*,#19146,.F.);
#26048=ORIENTED_EDGE('',*,*,#19150,.F.);
#26049=ORIENTED_EDGE('',*,*,#19153,.F.);
#26050=ORIENTED_EDGE('',*,*,#19156,.F.);
#26051=ORIENTED_EDGE('',*,*,#19157,.T.);
#26052=ORIENTED_EDGE('',*,*,#19158,.T.);
#26053=ORIENTED_EDGE('',*,*,#19159,.F.);
#26054=ORIENTED_EDGE('',*,*,#19160,.F.);
#26055=ORIENTED_EDGE('',*,*,#19161,.T.);
#26056=ORIENTED_EDGE('',*,*,#19162,.T.);
#26057=ORIENTED_EDGE('',*,*,#19157,.F.);
#26058=ORIENTED_EDGE('',*,*,#19163,.F.);
#26059=ORIENTED_EDGE('',*,*,#19164,.T.);
#26060=ORIENTED_EDGE('',*,*,#19165,.T.);
#26061=ORIENTED_EDGE('',*,*,#19161,.F.);
#26062=ORIENTED_EDGE('',*,*,#19166,.F.);
#26063=ORIENTED_EDGE('',*,*,#19159,.T.);
#26064=ORIENTED_EDGE('',*,*,#19167,.T.);
#26065=ORIENTED_EDGE('',*,*,#19164,.F.);
#26066=ORIENTED_EDGE('',*,*,#19167,.F.);
#26067=ORIENTED_EDGE('',*,*,#19158,.F.);
#26068=ORIENTED_EDGE('',*,*,#19162,.F.);
#26069=ORIENTED_EDGE('',*,*,#19165,.F.);
#26070=ORIENTED_EDGE('',*,*,#19168,.F.);
#26071=ORIENTED_EDGE('',*,*,#19169,.T.);
#26072=ORIENTED_EDGE('',*,*,#19170,.T.);
#26073=ORIENTED_EDGE('',*,*,#19171,.F.);
#26074=ORIENTED_EDGE('',*,*,#19172,.F.);
#26075=ORIENTED_EDGE('',*,*,#19173,.T.);
#26076=ORIENTED_EDGE('',*,*,#19174,.T.);
#26077=ORIENTED_EDGE('',*,*,#19169,.F.);
#26078=ORIENTED_EDGE('',*,*,#19175,.F.);
#26079=ORIENTED_EDGE('',*,*,#19176,.T.);
#26080=ORIENTED_EDGE('',*,*,#19177,.T.);
#26081=ORIENTED_EDGE('',*,*,#19173,.F.);
#26082=ORIENTED_EDGE('',*,*,#19178,.F.);
#26083=ORIENTED_EDGE('',*,*,#19171,.T.);
#26084=ORIENTED_EDGE('',*,*,#19179,.T.);
#26085=ORIENTED_EDGE('',*,*,#19176,.F.);
#26086=ORIENTED_EDGE('',*,*,#19179,.F.);
#26087=ORIENTED_EDGE('',*,*,#19170,.F.);
#26088=ORIENTED_EDGE('',*,*,#19174,.F.);
#26089=ORIENTED_EDGE('',*,*,#19177,.F.);
#26090=ORIENTED_EDGE('',*,*,#19180,.F.);
#26091=ORIENTED_EDGE('',*,*,#19181,.T.);
#26092=ORIENTED_EDGE('',*,*,#19182,.T.);
#26093=ORIENTED_EDGE('',*,*,#19183,.F.);
#26094=ORIENTED_EDGE('',*,*,#19184,.F.);
#26095=ORIENTED_EDGE('',*,*,#19185,.T.);
#26096=ORIENTED_EDGE('',*,*,#19186,.T.);
#26097=ORIENTED_EDGE('',*,*,#19181,.F.);
#26098=ORIENTED_EDGE('',*,*,#19187,.F.);
#26099=ORIENTED_EDGE('',*,*,#19188,.T.);
#26100=ORIENTED_EDGE('',*,*,#19189,.T.);
#26101=ORIENTED_EDGE('',*,*,#19185,.F.);
#26102=ORIENTED_EDGE('',*,*,#19190,.F.);
#26103=ORIENTED_EDGE('',*,*,#19183,.T.);
#26104=ORIENTED_EDGE('',*,*,#19191,.T.);
#26105=ORIENTED_EDGE('',*,*,#19188,.F.);
#26106=ORIENTED_EDGE('',*,*,#19191,.F.);
#26107=ORIENTED_EDGE('',*,*,#19182,.F.);
#26108=ORIENTED_EDGE('',*,*,#19186,.F.);
#26109=ORIENTED_EDGE('',*,*,#19189,.F.);
#26110=ORIENTED_EDGE('',*,*,#19192,.F.);
#26111=ORIENTED_EDGE('',*,*,#19193,.T.);
#26112=ORIENTED_EDGE('',*,*,#19194,.T.);
#26113=ORIENTED_EDGE('',*,*,#19195,.F.);
#26114=ORIENTED_EDGE('',*,*,#19196,.F.);
#26115=ORIENTED_EDGE('',*,*,#19197,.T.);
#26116=ORIENTED_EDGE('',*,*,#19198,.T.);
#26117=ORIENTED_EDGE('',*,*,#19193,.F.);
#26118=ORIENTED_EDGE('',*,*,#19199,.F.);
#26119=ORIENTED_EDGE('',*,*,#19200,.T.);
#26120=ORIENTED_EDGE('',*,*,#19201,.T.);
#26121=ORIENTED_EDGE('',*,*,#19197,.F.);
#26122=ORIENTED_EDGE('',*,*,#19202,.F.);
#26123=ORIENTED_EDGE('',*,*,#19195,.T.);
#26124=ORIENTED_EDGE('',*,*,#19203,.T.);
#26125=ORIENTED_EDGE('',*,*,#19200,.F.);
#26126=ORIENTED_EDGE('',*,*,#19203,.F.);
#26127=ORIENTED_EDGE('',*,*,#19194,.F.);
#26128=ORIENTED_EDGE('',*,*,#19198,.F.);
#26129=ORIENTED_EDGE('',*,*,#19201,.F.);
#26130=ORIENTED_EDGE('',*,*,#19204,.F.);
#26131=ORIENTED_EDGE('',*,*,#19205,.T.);
#26132=ORIENTED_EDGE('',*,*,#19206,.T.);
#26133=ORIENTED_EDGE('',*,*,#19207,.F.);
#26134=ORIENTED_EDGE('',*,*,#19208,.F.);
#26135=ORIENTED_EDGE('',*,*,#19209,.T.);
#26136=ORIENTED_EDGE('',*,*,#19210,.T.);
#26137=ORIENTED_EDGE('',*,*,#19205,.F.);
#26138=ORIENTED_EDGE('',*,*,#19211,.F.);
#26139=ORIENTED_EDGE('',*,*,#19212,.T.);
#26140=ORIENTED_EDGE('',*,*,#19213,.T.);
#26141=ORIENTED_EDGE('',*,*,#19209,.F.);
#26142=ORIENTED_EDGE('',*,*,#19214,.F.);
#26143=ORIENTED_EDGE('',*,*,#19207,.T.);
#26144=ORIENTED_EDGE('',*,*,#19215,.T.);
#26145=ORIENTED_EDGE('',*,*,#19212,.F.);
#26146=ORIENTED_EDGE('',*,*,#19215,.F.);
#26147=ORIENTED_EDGE('',*,*,#19206,.F.);
#26148=ORIENTED_EDGE('',*,*,#19210,.F.);
#26149=ORIENTED_EDGE('',*,*,#19213,.F.);
#26150=ORIENTED_EDGE('',*,*,#19216,.F.);
#26151=ORIENTED_EDGE('',*,*,#19217,.T.);
#26152=ORIENTED_EDGE('',*,*,#19218,.T.);
#26153=ORIENTED_EDGE('',*,*,#19219,.F.);
#26154=ORIENTED_EDGE('',*,*,#19220,.F.);
#26155=ORIENTED_EDGE('',*,*,#19221,.T.);
#26156=ORIENTED_EDGE('',*,*,#19222,.T.);
#26157=ORIENTED_EDGE('',*,*,#19217,.F.);
#26158=ORIENTED_EDGE('',*,*,#19223,.F.);
#26159=ORIENTED_EDGE('',*,*,#19224,.T.);
#26160=ORIENTED_EDGE('',*,*,#19225,.T.);
#26161=ORIENTED_EDGE('',*,*,#19221,.F.);
#26162=ORIENTED_EDGE('',*,*,#19226,.F.);
#26163=ORIENTED_EDGE('',*,*,#19219,.T.);
#26164=ORIENTED_EDGE('',*,*,#19227,.T.);
#26165=ORIENTED_EDGE('',*,*,#19224,.F.);
#26166=ORIENTED_EDGE('',*,*,#19227,.F.);
#26167=ORIENTED_EDGE('',*,*,#19218,.F.);
#26168=ORIENTED_EDGE('',*,*,#19222,.F.);
#26169=ORIENTED_EDGE('',*,*,#19225,.F.);
#26170=ORIENTED_EDGE('',*,*,#19228,.F.);
#26171=ORIENTED_EDGE('',*,*,#19229,.T.);
#26172=ORIENTED_EDGE('',*,*,#19230,.T.);
#26173=ORIENTED_EDGE('',*,*,#19231,.F.);
#26174=ORIENTED_EDGE('',*,*,#19232,.F.);
#26175=ORIENTED_EDGE('',*,*,#19233,.T.);
#26176=ORIENTED_EDGE('',*,*,#19234,.T.);
#26177=ORIENTED_EDGE('',*,*,#19229,.F.);
#26178=ORIENTED_EDGE('',*,*,#19235,.F.);
#26179=ORIENTED_EDGE('',*,*,#19236,.T.);
#26180=ORIENTED_EDGE('',*,*,#19237,.T.);
#26181=ORIENTED_EDGE('',*,*,#19233,.F.);
#26182=ORIENTED_EDGE('',*,*,#19238,.F.);
#26183=ORIENTED_EDGE('',*,*,#19231,.T.);
#26184=ORIENTED_EDGE('',*,*,#19239,.T.);
#26185=ORIENTED_EDGE('',*,*,#19236,.F.);
#26186=ORIENTED_EDGE('',*,*,#19239,.F.);
#26187=ORIENTED_EDGE('',*,*,#19230,.F.);
#26188=ORIENTED_EDGE('',*,*,#19234,.F.);
#26189=ORIENTED_EDGE('',*,*,#19237,.F.);
#26190=ORIENTED_EDGE('',*,*,#19240,.F.);
#26191=ORIENTED_EDGE('',*,*,#19241,.T.);
#26192=ORIENTED_EDGE('',*,*,#19242,.T.);
#26193=ORIENTED_EDGE('',*,*,#19243,.F.);
#26194=ORIENTED_EDGE('',*,*,#19244,.F.);
#26195=ORIENTED_EDGE('',*,*,#19245,.T.);
#26196=ORIENTED_EDGE('',*,*,#19246,.T.);
#26197=ORIENTED_EDGE('',*,*,#19241,.F.);
#26198=ORIENTED_EDGE('',*,*,#19247,.F.);
#26199=ORIENTED_EDGE('',*,*,#19248,.T.);
#26200=ORIENTED_EDGE('',*,*,#19249,.T.);
#26201=ORIENTED_EDGE('',*,*,#19245,.F.);
#26202=ORIENTED_EDGE('',*,*,#19250,.F.);
#26203=ORIENTED_EDGE('',*,*,#19243,.T.);
#26204=ORIENTED_EDGE('',*,*,#19251,.T.);
#26205=ORIENTED_EDGE('',*,*,#19248,.F.);
#26206=ORIENTED_EDGE('',*,*,#19251,.F.);
#26207=ORIENTED_EDGE('',*,*,#19242,.F.);
#26208=ORIENTED_EDGE('',*,*,#19246,.F.);
#26209=ORIENTED_EDGE('',*,*,#19249,.F.);
#26210=ORIENTED_EDGE('',*,*,#19252,.F.);
#26211=ORIENTED_EDGE('',*,*,#19253,.T.);
#26212=ORIENTED_EDGE('',*,*,#19254,.F.);
#26213=ORIENTED_EDGE('',*,*,#19253,.F.);
#26214=ORIENTED_EDGE('',*,*,#19255,.F.);
#26215=ORIENTED_EDGE('',*,*,#19256,.T.);
#26216=ORIENTED_EDGE('',*,*,#19257,.F.);
#26217=ORIENTED_EDGE('',*,*,#19256,.F.);
#26218=ORIENTED_EDGE('',*,*,#19258,.T.);
#26219=ORIENTED_EDGE('',*,*,#19259,.T.);
#26220=ORIENTED_EDGE('',*,*,#19260,.F.);
#26221=ORIENTED_EDGE('',*,*,#19261,.F.);
#26222=ORIENTED_EDGE('',*,*,#19262,.T.);
#26223=ORIENTED_EDGE('',*,*,#19261,.T.);
#26224=ORIENTED_EDGE('',*,*,#19263,.F.);
#26225=ORIENTED_EDGE('',*,*,#19264,.F.);
#26226=ORIENTED_EDGE('',*,*,#19265,.T.);
#26227=ORIENTED_EDGE('',*,*,#19264,.T.);
#26228=ORIENTED_EDGE('',*,*,#19266,.F.);
#26229=ORIENTED_EDGE('',*,*,#19267,.F.);
#26230=ORIENTED_EDGE('',*,*,#19268,.T.);
#26231=ORIENTED_EDGE('',*,*,#19267,.T.);
#26232=ORIENTED_EDGE('',*,*,#19269,.F.);
#26233=ORIENTED_EDGE('',*,*,#19270,.F.);
#26234=ORIENTED_EDGE('',*,*,#19271,.T.);
#26235=ORIENTED_EDGE('',*,*,#19270,.T.);
#26236=ORIENTED_EDGE('',*,*,#19272,.F.);
#26237=ORIENTED_EDGE('',*,*,#19273,.F.);
#26238=ORIENTED_EDGE('',*,*,#19274,.T.);
#26239=ORIENTED_EDGE('',*,*,#19273,.T.);
#26240=ORIENTED_EDGE('',*,*,#19275,.F.);
#26241=ORIENTED_EDGE('',*,*,#19276,.F.);
#26242=ORIENTED_EDGE('',*,*,#19277,.T.);
#26243=ORIENTED_EDGE('',*,*,#19276,.T.);
#26244=ORIENTED_EDGE('',*,*,#19278,.F.);
#26245=ORIENTED_EDGE('',*,*,#19279,.F.);
#26246=ORIENTED_EDGE('',*,*,#19280,.T.);
#26247=ORIENTED_EDGE('',*,*,#19279,.T.);
#26248=ORIENTED_EDGE('',*,*,#19281,.F.);
#26249=ORIENTED_EDGE('',*,*,#19259,.F.);
#26250=ORIENTED_EDGE('',*,*,#19281,.T.);
#26251=ORIENTED_EDGE('',*,*,#19278,.T.);
#26252=ORIENTED_EDGE('',*,*,#19275,.T.);
#26253=ORIENTED_EDGE('',*,*,#19272,.T.);
#26254=ORIENTED_EDGE('',*,*,#19269,.T.);
#26255=ORIENTED_EDGE('',*,*,#19266,.T.);
#26256=ORIENTED_EDGE('',*,*,#19263,.T.);
#26257=ORIENTED_EDGE('',*,*,#19260,.T.);
#26258=ORIENTED_EDGE('',*,*,#17368,.T.);
#26259=ORIENTED_EDGE('',*,*,#17402,.T.);
#26260=ORIENTED_EDGE('',*,*,#17399,.T.);
#26261=ORIENTED_EDGE('',*,*,#17396,.T.);
#26262=ORIENTED_EDGE('',*,*,#17393,.T.);
#26263=ORIENTED_EDGE('',*,*,#17390,.T.);
#26264=ORIENTED_EDGE('',*,*,#17387,.T.);
#26265=ORIENTED_EDGE('',*,*,#17384,.T.);
#26266=ORIENTED_EDGE('',*,*,#17381,.T.);
#26267=ORIENTED_EDGE('',*,*,#17378,.T.);
#26268=ORIENTED_EDGE('',*,*,#17375,.T.);
#26269=ORIENTED_EDGE('',*,*,#17372,.T.);
#26270=ORIENTED_EDGE('',*,*,#17404,.T.);
#26271=ORIENTED_EDGE('',*,*,#17492,.T.);
#26272=ORIENTED_EDGE('',*,*,#17489,.T.);
#26273=ORIENTED_EDGE('',*,*,#17486,.T.);
#26274=ORIENTED_EDGE('',*,*,#17483,.T.);
#26275=ORIENTED_EDGE('',*,*,#17480,.T.);
#26276=ORIENTED_EDGE('',*,*,#17477,.T.);
#26277=ORIENTED_EDGE('',*,*,#17474,.T.);
#26278=ORIENTED_EDGE('',*,*,#17471,.T.);
#26279=ORIENTED_EDGE('',*,*,#17468,.T.);
#26280=ORIENTED_EDGE('',*,*,#17465,.T.);
#26281=ORIENTED_EDGE('',*,*,#17462,.T.);
#26282=ORIENTED_EDGE('',*,*,#17459,.T.);
#26283=ORIENTED_EDGE('',*,*,#17456,.T.);
#26284=ORIENTED_EDGE('',*,*,#17453,.T.);
#26285=ORIENTED_EDGE('',*,*,#17450,.T.);
#26286=ORIENTED_EDGE('',*,*,#17447,.T.);
#26287=ORIENTED_EDGE('',*,*,#17444,.T.);
#26288=ORIENTED_EDGE('',*,*,#17441,.T.);
#26289=ORIENTED_EDGE('',*,*,#17438,.T.);
#26290=ORIENTED_EDGE('',*,*,#17435,.T.);
#26291=ORIENTED_EDGE('',*,*,#17432,.T.);
#26292=ORIENTED_EDGE('',*,*,#17429,.T.);
#26293=ORIENTED_EDGE('',*,*,#17426,.T.);
#26294=ORIENTED_EDGE('',*,*,#17423,.T.);
#26295=ORIENTED_EDGE('',*,*,#17420,.T.);
#26296=ORIENTED_EDGE('',*,*,#17417,.T.);
#26297=ORIENTED_EDGE('',*,*,#17414,.T.);
#26298=ORIENTED_EDGE('',*,*,#17411,.T.);
#26299=ORIENTED_EDGE('',*,*,#17408,.T.);
#26300=ORIENTED_EDGE('',*,*,#17644,.T.);
#26301=ORIENTED_EDGE('',*,*,#17678,.T.);
#26302=ORIENTED_EDGE('',*,*,#17675,.T.);
#26303=ORIENTED_EDGE('',*,*,#17672,.T.);
#26304=ORIENTED_EDGE('',*,*,#17669,.T.);
#26305=ORIENTED_EDGE('',*,*,#17666,.T.);
#26306=ORIENTED_EDGE('',*,*,#17663,.T.);
#26307=ORIENTED_EDGE('',*,*,#17660,.T.);
#26308=ORIENTED_EDGE('',*,*,#17657,.T.);
#26309=ORIENTED_EDGE('',*,*,#17654,.T.);
#26310=ORIENTED_EDGE('',*,*,#17651,.T.);
#26311=ORIENTED_EDGE('',*,*,#17648,.T.);
#26312=ORIENTED_EDGE('',*,*,#17680,.T.);
#26313=ORIENTED_EDGE('',*,*,#17705,.T.);
#26314=ORIENTED_EDGE('',*,*,#17702,.T.);
#26315=ORIENTED_EDGE('',*,*,#17699,.T.);
#26316=ORIENTED_EDGE('',*,*,#17696,.T.);
#26317=ORIENTED_EDGE('',*,*,#17693,.T.);
#26318=ORIENTED_EDGE('',*,*,#17690,.T.);
#26319=ORIENTED_EDGE('',*,*,#17687,.T.);
#26320=ORIENTED_EDGE('',*,*,#17684,.T.);
#26321=ORIENTED_EDGE('',*,*,#17791,.T.);
#26322=ORIENTED_EDGE('',*,*,#17825,.T.);
#26323=ORIENTED_EDGE('',*,*,#17822,.T.);
#26324=ORIENTED_EDGE('',*,*,#17819,.T.);
#26325=ORIENTED_EDGE('',*,*,#17816,.T.);
#26326=ORIENTED_EDGE('',*,*,#17813,.T.);
#26327=ORIENTED_EDGE('',*,*,#17810,.T.);
#26328=ORIENTED_EDGE('',*,*,#17807,.T.);
#26329=ORIENTED_EDGE('',*,*,#17804,.T.);
#26330=ORIENTED_EDGE('',*,*,#17801,.T.);
#26331=ORIENTED_EDGE('',*,*,#17798,.T.);
#26332=ORIENTED_EDGE('',*,*,#17795,.T.);
#26333=ORIENTED_EDGE('',*,*,#17827,.T.);
#26334=ORIENTED_EDGE('',*,*,#17852,.T.);
#26335=ORIENTED_EDGE('',*,*,#17849,.T.);
#26336=ORIENTED_EDGE('',*,*,#17846,.T.);
#26337=ORIENTED_EDGE('',*,*,#17843,.T.);
#26338=ORIENTED_EDGE('',*,*,#17840,.T.);
#26339=ORIENTED_EDGE('',*,*,#17837,.T.);
#26340=ORIENTED_EDGE('',*,*,#17834,.T.);
#26341=ORIENTED_EDGE('',*,*,#17831,.T.);
#26342=ORIENTED_EDGE('',*,*,#18004,.T.);
#26343=ORIENTED_EDGE('',*,*,#18038,.T.);
#26344=ORIENTED_EDGE('',*,*,#18035,.T.);
#26345=ORIENTED_EDGE('',*,*,#18032,.T.);
#26346=ORIENTED_EDGE('',*,*,#18029,.T.);
#26347=ORIENTED_EDGE('',*,*,#18026,.T.);
#26348=ORIENTED_EDGE('',*,*,#18023,.T.);
#26349=ORIENTED_EDGE('',*,*,#18020,.T.);
#26350=ORIENTED_EDGE('',*,*,#18017,.T.);
#26351=ORIENTED_EDGE('',*,*,#18014,.T.);
#26352=ORIENTED_EDGE('',*,*,#18011,.T.);
#26353=ORIENTED_EDGE('',*,*,#18008,.T.);
#26354=ORIENTED_EDGE('',*,*,#18040,.T.);
#26355=ORIENTED_EDGE('',*,*,#18128,.T.);
#26356=ORIENTED_EDGE('',*,*,#18125,.T.);
#26357=ORIENTED_EDGE('',*,*,#18122,.T.);
#26358=ORIENTED_EDGE('',*,*,#18119,.T.);
#26359=ORIENTED_EDGE('',*,*,#18116,.T.);
#26360=ORIENTED_EDGE('',*,*,#18113,.T.);
#26361=ORIENTED_EDGE('',*,*,#18110,.T.);
#26362=ORIENTED_EDGE('',*,*,#18107,.T.);
#26363=ORIENTED_EDGE('',*,*,#18104,.T.);
#26364=ORIENTED_EDGE('',*,*,#18101,.T.);
#26365=ORIENTED_EDGE('',*,*,#18098,.T.);
#26366=ORIENTED_EDGE('',*,*,#18095,.T.);
#26367=ORIENTED_EDGE('',*,*,#18092,.T.);
#26368=ORIENTED_EDGE('',*,*,#18089,.T.);
#26369=ORIENTED_EDGE('',*,*,#18086,.T.);
#26370=ORIENTED_EDGE('',*,*,#18083,.T.);
#26371=ORIENTED_EDGE('',*,*,#18080,.T.);
#26372=ORIENTED_EDGE('',*,*,#18077,.T.);
#26373=ORIENTED_EDGE('',*,*,#18074,.T.);
#26374=ORIENTED_EDGE('',*,*,#18071,.T.);
#26375=ORIENTED_EDGE('',*,*,#18068,.T.);
#26376=ORIENTED_EDGE('',*,*,#18065,.T.);
#26377=ORIENTED_EDGE('',*,*,#18062,.T.);
#26378=ORIENTED_EDGE('',*,*,#18059,.T.);
#26379=ORIENTED_EDGE('',*,*,#18056,.T.);
#26380=ORIENTED_EDGE('',*,*,#18053,.T.);
#26381=ORIENTED_EDGE('',*,*,#18050,.T.);
#26382=ORIENTED_EDGE('',*,*,#18047,.T.);
#26383=ORIENTED_EDGE('',*,*,#18044,.T.);
#26384=ORIENTED_EDGE('',*,*,#18232,.T.);
#26385=ORIENTED_EDGE('',*,*,#18242,.T.);
#26386=ORIENTED_EDGE('',*,*,#18239,.T.);
#26387=ORIENTED_EDGE('',*,*,#18236,.T.);
#26388=ORIENTED_EDGE('',*,*,#18244,.T.);
#26389=ORIENTED_EDGE('',*,*,#18254,.T.);
#26390=ORIENTED_EDGE('',*,*,#18251,.T.);
#26391=ORIENTED_EDGE('',*,*,#18248,.T.);
#26392=ORIENTED_EDGE('',*,*,#18256,.T.);
#26393=ORIENTED_EDGE('',*,*,#18266,.T.);
#26394=ORIENTED_EDGE('',*,*,#18263,.T.);
#26395=ORIENTED_EDGE('',*,*,#18260,.T.);
#26396=ORIENTED_EDGE('',*,*,#18268,.T.);
#26397=ORIENTED_EDGE('',*,*,#18278,.T.);
#26398=ORIENTED_EDGE('',*,*,#18275,.T.);
#26399=ORIENTED_EDGE('',*,*,#18272,.T.);
#26400=ORIENTED_EDGE('',*,*,#18280,.T.);
#26401=ORIENTED_EDGE('',*,*,#18290,.T.);
#26402=ORIENTED_EDGE('',*,*,#18287,.T.);
#26403=ORIENTED_EDGE('',*,*,#18284,.T.);
#26404=ORIENTED_EDGE('',*,*,#18292,.T.);
#26405=ORIENTED_EDGE('',*,*,#18302,.T.);
#26406=ORIENTED_EDGE('',*,*,#18299,.T.);
#26407=ORIENTED_EDGE('',*,*,#18296,.T.);
#26408=ORIENTED_EDGE('',*,*,#18304,.T.);
#26409=ORIENTED_EDGE('',*,*,#18314,.T.);
#26410=ORIENTED_EDGE('',*,*,#18311,.T.);
#26411=ORIENTED_EDGE('',*,*,#18308,.T.);
#26412=ORIENTED_EDGE('',*,*,#18316,.T.);
#26413=ORIENTED_EDGE('',*,*,#18326,.T.);
#26414=ORIENTED_EDGE('',*,*,#18323,.T.);
#26415=ORIENTED_EDGE('',*,*,#18320,.T.);
#26416=ORIENTED_EDGE('',*,*,#18328,.T.);
#26417=ORIENTED_EDGE('',*,*,#18338,.T.);
#26418=ORIENTED_EDGE('',*,*,#18335,.T.);
#26419=ORIENTED_EDGE('',*,*,#18332,.T.);
#26420=ORIENTED_EDGE('',*,*,#18340,.T.);
#26421=ORIENTED_EDGE('',*,*,#18350,.T.);
#26422=ORIENTED_EDGE('',*,*,#18347,.T.);
#26423=ORIENTED_EDGE('',*,*,#18344,.T.);
#26424=ORIENTED_EDGE('',*,*,#18352,.T.);
#26425=ORIENTED_EDGE('',*,*,#18362,.T.);
#26426=ORIENTED_EDGE('',*,*,#18359,.T.);
#26427=ORIENTED_EDGE('',*,*,#18356,.T.);
#26428=ORIENTED_EDGE('',*,*,#18364,.T.);
#26429=ORIENTED_EDGE('',*,*,#18374,.T.);
#26430=ORIENTED_EDGE('',*,*,#18371,.T.);
#26431=ORIENTED_EDGE('',*,*,#18368,.T.);
#26432=ORIENTED_EDGE('',*,*,#18376,.T.);
#26433=ORIENTED_EDGE('',*,*,#18386,.T.);
#26434=ORIENTED_EDGE('',*,*,#18383,.T.);
#26435=ORIENTED_EDGE('',*,*,#18380,.T.);
#26436=ORIENTED_EDGE('',*,*,#18388,.T.);
#26437=ORIENTED_EDGE('',*,*,#18398,.T.);
#26438=ORIENTED_EDGE('',*,*,#18395,.T.);
#26439=ORIENTED_EDGE('',*,*,#18392,.T.);
#26440=ORIENTED_EDGE('',*,*,#18400,.T.);
#26441=ORIENTED_EDGE('',*,*,#18410,.T.);
#26442=ORIENTED_EDGE('',*,*,#18407,.T.);
#26443=ORIENTED_EDGE('',*,*,#18404,.T.);
#26444=ORIENTED_EDGE('',*,*,#18412,.T.);
#26445=ORIENTED_EDGE('',*,*,#18422,.T.);
#26446=ORIENTED_EDGE('',*,*,#18419,.T.);
#26447=ORIENTED_EDGE('',*,*,#18416,.T.);
#26448=ORIENTED_EDGE('',*,*,#18424,.T.);
#26449=ORIENTED_EDGE('',*,*,#18434,.T.);
#26450=ORIENTED_EDGE('',*,*,#18431,.T.);
#26451=ORIENTED_EDGE('',*,*,#18428,.T.);
#26452=ORIENTED_EDGE('',*,*,#18436,.T.);
#26453=ORIENTED_EDGE('',*,*,#18446,.T.);
#26454=ORIENTED_EDGE('',*,*,#18443,.T.);
#26455=ORIENTED_EDGE('',*,*,#18440,.T.);
#26456=ORIENTED_EDGE('',*,*,#18448,.T.);
#26457=ORIENTED_EDGE('',*,*,#18458,.T.);
#26458=ORIENTED_EDGE('',*,*,#18455,.T.);
#26459=ORIENTED_EDGE('',*,*,#18452,.T.);
#26460=ORIENTED_EDGE('',*,*,#18460,.T.);
#26461=ORIENTED_EDGE('',*,*,#18470,.T.);
#26462=ORIENTED_EDGE('',*,*,#18467,.T.);
#26463=ORIENTED_EDGE('',*,*,#18464,.T.);
#26464=ORIENTED_EDGE('',*,*,#18472,.T.);
#26465=ORIENTED_EDGE('',*,*,#18482,.T.);
#26466=ORIENTED_EDGE('',*,*,#18479,.T.);
#26467=ORIENTED_EDGE('',*,*,#18476,.T.);
#26468=ORIENTED_EDGE('',*,*,#18484,.T.);
#26469=ORIENTED_EDGE('',*,*,#18494,.T.);
#26470=ORIENTED_EDGE('',*,*,#18491,.T.);
#26471=ORIENTED_EDGE('',*,*,#18488,.T.);
#26472=ORIENTED_EDGE('',*,*,#18496,.T.);
#26473=ORIENTED_EDGE('',*,*,#18506,.T.);
#26474=ORIENTED_EDGE('',*,*,#18503,.T.);
#26475=ORIENTED_EDGE('',*,*,#18500,.T.);
#26476=ORIENTED_EDGE('',*,*,#18508,.T.);
#26477=ORIENTED_EDGE('',*,*,#18518,.T.);
#26478=ORIENTED_EDGE('',*,*,#18515,.T.);
#26479=ORIENTED_EDGE('',*,*,#18512,.T.);
#26480=ORIENTED_EDGE('',*,*,#18520,.T.);
#26481=ORIENTED_EDGE('',*,*,#18530,.T.);
#26482=ORIENTED_EDGE('',*,*,#18527,.T.);
#26483=ORIENTED_EDGE('',*,*,#18524,.T.);
#26484=ORIENTED_EDGE('',*,*,#18532,.T.);
#26485=ORIENTED_EDGE('',*,*,#18542,.T.);
#26486=ORIENTED_EDGE('',*,*,#18539,.T.);
#26487=ORIENTED_EDGE('',*,*,#18536,.T.);
#26488=ORIENTED_EDGE('',*,*,#18544,.T.);
#26489=ORIENTED_EDGE('',*,*,#18554,.T.);
#26490=ORIENTED_EDGE('',*,*,#18551,.T.);
#26491=ORIENTED_EDGE('',*,*,#18548,.T.);
#26492=ORIENTED_EDGE('',*,*,#18556,.T.);
#26493=ORIENTED_EDGE('',*,*,#18566,.T.);
#26494=ORIENTED_EDGE('',*,*,#18563,.T.);
#26495=ORIENTED_EDGE('',*,*,#18560,.T.);
#26496=ORIENTED_EDGE('',*,*,#18568,.T.);
#26497=ORIENTED_EDGE('',*,*,#18578,.T.);
#26498=ORIENTED_EDGE('',*,*,#18575,.T.);
#26499=ORIENTED_EDGE('',*,*,#18572,.T.);
#26500=ORIENTED_EDGE('',*,*,#18580,.T.);
#26501=ORIENTED_EDGE('',*,*,#18590,.T.);
#26502=ORIENTED_EDGE('',*,*,#18587,.T.);
#26503=ORIENTED_EDGE('',*,*,#18584,.T.);
#26504=ORIENTED_EDGE('',*,*,#18592,.T.);
#26505=ORIENTED_EDGE('',*,*,#18602,.T.);
#26506=ORIENTED_EDGE('',*,*,#18599,.T.);
#26507=ORIENTED_EDGE('',*,*,#18596,.T.);
#26508=ORIENTED_EDGE('',*,*,#18604,.T.);
#26509=ORIENTED_EDGE('',*,*,#18614,.T.);
#26510=ORIENTED_EDGE('',*,*,#18611,.T.);
#26511=ORIENTED_EDGE('',*,*,#18608,.T.);
#26512=ORIENTED_EDGE('',*,*,#18616,.T.);
#26513=ORIENTED_EDGE('',*,*,#18626,.T.);
#26514=ORIENTED_EDGE('',*,*,#18623,.T.);
#26515=ORIENTED_EDGE('',*,*,#18620,.T.);
#26516=ORIENTED_EDGE('',*,*,#18628,.T.);
#26517=ORIENTED_EDGE('',*,*,#18638,.T.);
#26518=ORIENTED_EDGE('',*,*,#18635,.T.);
#26519=ORIENTED_EDGE('',*,*,#18632,.T.);
#26520=ORIENTED_EDGE('',*,*,#18640,.T.);
#26521=ORIENTED_EDGE('',*,*,#18650,.T.);
#26522=ORIENTED_EDGE('',*,*,#18647,.T.);
#26523=ORIENTED_EDGE('',*,*,#18644,.T.);
#26524=ORIENTED_EDGE('',*,*,#18652,.T.);
#26525=ORIENTED_EDGE('',*,*,#18662,.T.);
#26526=ORIENTED_EDGE('',*,*,#18659,.T.);
#26527=ORIENTED_EDGE('',*,*,#18656,.T.);
#26528=ORIENTED_EDGE('',*,*,#18664,.T.);
#26529=ORIENTED_EDGE('',*,*,#18674,.T.);
#26530=ORIENTED_EDGE('',*,*,#18671,.T.);
#26531=ORIENTED_EDGE('',*,*,#18668,.T.);
#26532=ORIENTED_EDGE('',*,*,#18676,.T.);
#26533=ORIENTED_EDGE('',*,*,#18686,.T.);
#26534=ORIENTED_EDGE('',*,*,#18683,.T.);
#26535=ORIENTED_EDGE('',*,*,#18680,.T.);
#26536=ORIENTED_EDGE('',*,*,#18688,.T.);
#26537=ORIENTED_EDGE('',*,*,#18698,.T.);
#26538=ORIENTED_EDGE('',*,*,#18695,.T.);
#26539=ORIENTED_EDGE('',*,*,#18692,.T.);
#26540=ORIENTED_EDGE('',*,*,#18700,.T.);
#26541=ORIENTED_EDGE('',*,*,#18710,.T.);
#26542=ORIENTED_EDGE('',*,*,#18707,.T.);
#26543=ORIENTED_EDGE('',*,*,#18704,.T.);
#26544=ORIENTED_EDGE('',*,*,#18712,.T.);
#26545=ORIENTED_EDGE('',*,*,#18722,.T.);
#26546=ORIENTED_EDGE('',*,*,#18719,.T.);
#26547=ORIENTED_EDGE('',*,*,#18716,.T.);
#26548=ORIENTED_EDGE('',*,*,#18724,.T.);
#26549=ORIENTED_EDGE('',*,*,#18734,.T.);
#26550=ORIENTED_EDGE('',*,*,#18731,.T.);
#26551=ORIENTED_EDGE('',*,*,#18728,.T.);
#26552=ORIENTED_EDGE('',*,*,#18736,.T.);
#26553=ORIENTED_EDGE('',*,*,#18746,.T.);
#26554=ORIENTED_EDGE('',*,*,#18743,.T.);
#26555=ORIENTED_EDGE('',*,*,#18740,.T.);
#26556=ORIENTED_EDGE('',*,*,#18748,.T.);
#26557=ORIENTED_EDGE('',*,*,#18758,.T.);
#26558=ORIENTED_EDGE('',*,*,#18755,.T.);
#26559=ORIENTED_EDGE('',*,*,#18752,.T.);
#26560=ORIENTED_EDGE('',*,*,#18760,.T.);
#26561=ORIENTED_EDGE('',*,*,#18770,.T.);
#26562=ORIENTED_EDGE('',*,*,#18767,.T.);
#26563=ORIENTED_EDGE('',*,*,#18764,.T.);
#26564=ORIENTED_EDGE('',*,*,#18772,.T.);
#26565=ORIENTED_EDGE('',*,*,#18782,.T.);
#26566=ORIENTED_EDGE('',*,*,#18779,.T.);
#26567=ORIENTED_EDGE('',*,*,#18776,.T.);
#26568=ORIENTED_EDGE('',*,*,#18784,.T.);
#26569=ORIENTED_EDGE('',*,*,#18794,.T.);
#26570=ORIENTED_EDGE('',*,*,#18791,.T.);
#26571=ORIENTED_EDGE('',*,*,#18788,.T.);
#26572=ORIENTED_EDGE('',*,*,#18796,.T.);
#26573=ORIENTED_EDGE('',*,*,#18806,.T.);
#26574=ORIENTED_EDGE('',*,*,#18803,.T.);
#26575=ORIENTED_EDGE('',*,*,#18800,.T.);
#26576=ORIENTED_EDGE('',*,*,#18808,.T.);
#26577=ORIENTED_EDGE('',*,*,#18818,.T.);
#26578=ORIENTED_EDGE('',*,*,#18815,.T.);
#26579=ORIENTED_EDGE('',*,*,#18812,.T.);
#26580=ORIENTED_EDGE('',*,*,#18820,.T.);
#26581=ORIENTED_EDGE('',*,*,#18830,.T.);
#26582=ORIENTED_EDGE('',*,*,#18827,.T.);
#26583=ORIENTED_EDGE('',*,*,#18824,.T.);
#26584=ORIENTED_EDGE('',*,*,#18832,.T.);
#26585=ORIENTED_EDGE('',*,*,#18842,.T.);
#26586=ORIENTED_EDGE('',*,*,#18839,.T.);
#26587=ORIENTED_EDGE('',*,*,#18836,.T.);
#26588=ORIENTED_EDGE('',*,*,#18844,.T.);
#26589=ORIENTED_EDGE('',*,*,#18854,.T.);
#26590=ORIENTED_EDGE('',*,*,#18851,.T.);
#26591=ORIENTED_EDGE('',*,*,#18848,.T.);
#26592=ORIENTED_EDGE('',*,*,#18856,.T.);
#26593=ORIENTED_EDGE('',*,*,#18866,.T.);
#26594=ORIENTED_EDGE('',*,*,#18863,.T.);
#26595=ORIENTED_EDGE('',*,*,#18860,.T.);
#26596=ORIENTED_EDGE('',*,*,#18868,.T.);
#26597=ORIENTED_EDGE('',*,*,#18878,.T.);
#26598=ORIENTED_EDGE('',*,*,#18875,.T.);
#26599=ORIENTED_EDGE('',*,*,#18872,.T.);
#26600=ORIENTED_EDGE('',*,*,#18880,.T.);
#26601=ORIENTED_EDGE('',*,*,#18890,.T.);
#26602=ORIENTED_EDGE('',*,*,#18887,.T.);
#26603=ORIENTED_EDGE('',*,*,#18884,.T.);
#26604=ORIENTED_EDGE('',*,*,#18892,.T.);
#26605=ORIENTED_EDGE('',*,*,#18902,.T.);
#26606=ORIENTED_EDGE('',*,*,#18899,.T.);
#26607=ORIENTED_EDGE('',*,*,#18896,.T.);
#26608=ORIENTED_EDGE('',*,*,#18904,.T.);
#26609=ORIENTED_EDGE('',*,*,#18914,.T.);
#26610=ORIENTED_EDGE('',*,*,#18911,.T.);
#26611=ORIENTED_EDGE('',*,*,#18908,.T.);
#26612=ORIENTED_EDGE('',*,*,#18916,.T.);
#26613=ORIENTED_EDGE('',*,*,#18926,.T.);
#26614=ORIENTED_EDGE('',*,*,#18923,.T.);
#26615=ORIENTED_EDGE('',*,*,#18920,.T.);
#26616=ORIENTED_EDGE('',*,*,#18928,.T.);
#26617=ORIENTED_EDGE('',*,*,#18938,.T.);
#26618=ORIENTED_EDGE('',*,*,#18935,.T.);
#26619=ORIENTED_EDGE('',*,*,#18932,.T.);
#26620=ORIENTED_EDGE('',*,*,#18940,.T.);
#26621=ORIENTED_EDGE('',*,*,#18950,.T.);
#26622=ORIENTED_EDGE('',*,*,#18947,.T.);
#26623=ORIENTED_EDGE('',*,*,#18944,.T.);
#26624=ORIENTED_EDGE('',*,*,#18952,.T.);
#26625=ORIENTED_EDGE('',*,*,#18962,.T.);
#26626=ORIENTED_EDGE('',*,*,#18959,.T.);
#26627=ORIENTED_EDGE('',*,*,#18956,.T.);
#26628=ORIENTED_EDGE('',*,*,#18964,.T.);
#26629=ORIENTED_EDGE('',*,*,#18974,.T.);
#26630=ORIENTED_EDGE('',*,*,#18971,.T.);
#26631=ORIENTED_EDGE('',*,*,#18968,.T.);
#26632=ORIENTED_EDGE('',*,*,#18976,.T.);
#26633=ORIENTED_EDGE('',*,*,#18986,.T.);
#26634=ORIENTED_EDGE('',*,*,#18983,.T.);
#26635=ORIENTED_EDGE('',*,*,#18980,.T.);
#26636=ORIENTED_EDGE('',*,*,#18988,.T.);
#26637=ORIENTED_EDGE('',*,*,#18998,.T.);
#26638=ORIENTED_EDGE('',*,*,#18995,.T.);
#26639=ORIENTED_EDGE('',*,*,#18992,.T.);
#26640=ORIENTED_EDGE('',*,*,#19000,.T.);
#26641=ORIENTED_EDGE('',*,*,#19010,.T.);
#26642=ORIENTED_EDGE('',*,*,#19007,.T.);
#26643=ORIENTED_EDGE('',*,*,#19004,.T.);
#26644=ORIENTED_EDGE('',*,*,#19012,.T.);
#26645=ORIENTED_EDGE('',*,*,#19022,.T.);
#26646=ORIENTED_EDGE('',*,*,#19019,.T.);
#26647=ORIENTED_EDGE('',*,*,#19016,.T.);
#26648=ORIENTED_EDGE('',*,*,#19024,.T.);
#26649=ORIENTED_EDGE('',*,*,#19034,.T.);
#26650=ORIENTED_EDGE('',*,*,#19031,.T.);
#26651=ORIENTED_EDGE('',*,*,#19028,.T.);
#26652=ORIENTED_EDGE('',*,*,#19036,.T.);
#26653=ORIENTED_EDGE('',*,*,#19046,.T.);
#26654=ORIENTED_EDGE('',*,*,#19043,.T.);
#26655=ORIENTED_EDGE('',*,*,#19040,.T.);
#26656=ORIENTED_EDGE('',*,*,#19048,.T.);
#26657=ORIENTED_EDGE('',*,*,#19058,.T.);
#26658=ORIENTED_EDGE('',*,*,#19055,.T.);
#26659=ORIENTED_EDGE('',*,*,#19052,.T.);
#26660=ORIENTED_EDGE('',*,*,#19060,.T.);
#26661=ORIENTED_EDGE('',*,*,#19070,.T.);
#26662=ORIENTED_EDGE('',*,*,#19067,.T.);
#26663=ORIENTED_EDGE('',*,*,#19064,.T.);
#26664=ORIENTED_EDGE('',*,*,#19072,.T.);
#26665=ORIENTED_EDGE('',*,*,#19082,.T.);
#26666=ORIENTED_EDGE('',*,*,#19079,.T.);
#26667=ORIENTED_EDGE('',*,*,#19076,.T.);
#26668=ORIENTED_EDGE('',*,*,#19084,.T.);
#26669=ORIENTED_EDGE('',*,*,#19094,.T.);
#26670=ORIENTED_EDGE('',*,*,#19091,.T.);
#26671=ORIENTED_EDGE('',*,*,#19088,.T.);
#26672=ORIENTED_EDGE('',*,*,#19096,.T.);
#26673=ORIENTED_EDGE('',*,*,#19106,.T.);
#26674=ORIENTED_EDGE('',*,*,#19103,.T.);
#26675=ORIENTED_EDGE('',*,*,#19100,.T.);
#26676=ORIENTED_EDGE('',*,*,#19108,.T.);
#26677=ORIENTED_EDGE('',*,*,#19118,.T.);
#26678=ORIENTED_EDGE('',*,*,#19115,.T.);
#26679=ORIENTED_EDGE('',*,*,#19112,.T.);
#26680=ORIENTED_EDGE('',*,*,#19120,.T.);
#26681=ORIENTED_EDGE('',*,*,#19130,.T.);
#26682=ORIENTED_EDGE('',*,*,#19127,.T.);
#26683=ORIENTED_EDGE('',*,*,#19124,.T.);
#26684=ORIENTED_EDGE('',*,*,#19132,.T.);
#26685=ORIENTED_EDGE('',*,*,#19142,.T.);
#26686=ORIENTED_EDGE('',*,*,#19139,.T.);
#26687=ORIENTED_EDGE('',*,*,#19136,.T.);
#26688=ORIENTED_EDGE('',*,*,#19144,.T.);
#26689=ORIENTED_EDGE('',*,*,#19154,.T.);
#26690=ORIENTED_EDGE('',*,*,#19151,.T.);
#26691=ORIENTED_EDGE('',*,*,#19148,.T.);
#26692=ORIENTED_EDGE('',*,*,#19156,.T.);
#26693=ORIENTED_EDGE('',*,*,#19166,.T.);
#26694=ORIENTED_EDGE('',*,*,#19163,.T.);
#26695=ORIENTED_EDGE('',*,*,#19160,.T.);
#26696=ORIENTED_EDGE('',*,*,#19168,.T.);
#26697=ORIENTED_EDGE('',*,*,#19178,.T.);
#26698=ORIENTED_EDGE('',*,*,#19175,.T.);
#26699=ORIENTED_EDGE('',*,*,#19172,.T.);
#26700=ORIENTED_EDGE('',*,*,#19180,.T.);
#26701=ORIENTED_EDGE('',*,*,#19190,.T.);
#26702=ORIENTED_EDGE('',*,*,#19187,.T.);
#26703=ORIENTED_EDGE('',*,*,#19184,.T.);
#26704=ORIENTED_EDGE('',*,*,#19192,.T.);
#26705=ORIENTED_EDGE('',*,*,#19202,.T.);
#26706=ORIENTED_EDGE('',*,*,#19199,.T.);
#26707=ORIENTED_EDGE('',*,*,#19196,.T.);
#26708=ORIENTED_EDGE('',*,*,#19204,.T.);
#26709=ORIENTED_EDGE('',*,*,#19214,.T.);
#26710=ORIENTED_EDGE('',*,*,#19211,.T.);
#26711=ORIENTED_EDGE('',*,*,#19208,.T.);
#26712=ORIENTED_EDGE('',*,*,#19216,.T.);
#26713=ORIENTED_EDGE('',*,*,#19226,.T.);
#26714=ORIENTED_EDGE('',*,*,#19223,.T.);
#26715=ORIENTED_EDGE('',*,*,#19220,.T.);
#26716=ORIENTED_EDGE('',*,*,#19228,.T.);
#26717=ORIENTED_EDGE('',*,*,#19238,.T.);
#26718=ORIENTED_EDGE('',*,*,#19235,.T.);
#26719=ORIENTED_EDGE('',*,*,#19232,.T.);
#26720=ORIENTED_EDGE('',*,*,#19240,.T.);
#26721=ORIENTED_EDGE('',*,*,#19250,.T.);
#26722=ORIENTED_EDGE('',*,*,#19247,.T.);
#26723=ORIENTED_EDGE('',*,*,#19244,.T.);
#26724=ORIENTED_EDGE('',*,*,#19254,.T.);
#26725=ORIENTED_EDGE('',*,*,#19257,.T.);
#26726=ORIENTED_EDGE('',*,*,#18199,.T.);
#26727=ORIENTED_EDGE('',*,*,#18230,.T.);
#26728=ORIENTED_EDGE('',*,*,#18227,.T.);
#26729=ORIENTED_EDGE('',*,*,#18224,.T.);
#26730=ORIENTED_EDGE('',*,*,#18221,.T.);
#26731=ORIENTED_EDGE('',*,*,#18218,.T.);
#26732=ORIENTED_EDGE('',*,*,#18215,.T.);
#26733=ORIENTED_EDGE('',*,*,#18212,.T.);
#26734=ORIENTED_EDGE('',*,*,#18209,.T.);
#26735=ORIENTED_EDGE('',*,*,#18206,.T.);
#26736=ORIENTED_EDGE('',*,*,#18203,.T.);
#26737=ORIENTED_EDGE('',*,*,#18154,.T.);
#26738=ORIENTED_EDGE('',*,*,#18188,.T.);
#26739=ORIENTED_EDGE('',*,*,#18185,.T.);
#26740=ORIENTED_EDGE('',*,*,#18182,.T.);
#26741=ORIENTED_EDGE('',*,*,#18179,.T.);
#26742=ORIENTED_EDGE('',*,*,#18176,.T.);
#26743=ORIENTED_EDGE('',*,*,#18173,.T.);
#26744=ORIENTED_EDGE('',*,*,#18170,.T.);
#26745=ORIENTED_EDGE('',*,*,#18167,.T.);
#26746=ORIENTED_EDGE('',*,*,#18164,.T.);
#26747=ORIENTED_EDGE('',*,*,#18161,.T.);
#26748=ORIENTED_EDGE('',*,*,#18158,.T.);
#26749=ORIENTED_EDGE('',*,*,#17914,.T.);
#26750=ORIENTED_EDGE('',*,*,#17978,.T.);
#26751=ORIENTED_EDGE('',*,*,#17975,.T.);
#26752=ORIENTED_EDGE('',*,*,#17972,.T.);
#26753=ORIENTED_EDGE('',*,*,#17969,.T.);
#26754=ORIENTED_EDGE('',*,*,#17966,.T.);
#26755=ORIENTED_EDGE('',*,*,#17963,.T.);
#26756=ORIENTED_EDGE('',*,*,#17960,.T.);
#26757=ORIENTED_EDGE('',*,*,#17957,.T.);
#26758=ORIENTED_EDGE('',*,*,#17954,.T.);
#26759=ORIENTED_EDGE('',*,*,#17951,.T.);
#26760=ORIENTED_EDGE('',*,*,#17948,.T.);
#26761=ORIENTED_EDGE('',*,*,#17945,.T.);
#26762=ORIENTED_EDGE('',*,*,#17942,.T.);
#26763=ORIENTED_EDGE('',*,*,#17939,.T.);
#26764=ORIENTED_EDGE('',*,*,#17936,.T.);
#26765=ORIENTED_EDGE('',*,*,#17933,.T.);
#26766=ORIENTED_EDGE('',*,*,#17930,.T.);
#26767=ORIENTED_EDGE('',*,*,#17927,.T.);
#26768=ORIENTED_EDGE('',*,*,#17924,.T.);
#26769=ORIENTED_EDGE('',*,*,#17921,.T.);
#26770=ORIENTED_EDGE('',*,*,#17918,.T.);
#26771=ORIENTED_EDGE('',*,*,#17878,.T.);
#26772=ORIENTED_EDGE('',*,*,#17912,.T.);
#26773=ORIENTED_EDGE('',*,*,#17909,.T.);
#26774=ORIENTED_EDGE('',*,*,#17906,.T.);
#26775=ORIENTED_EDGE('',*,*,#17903,.T.);
#26776=ORIENTED_EDGE('',*,*,#17900,.T.);
#26777=ORIENTED_EDGE('',*,*,#17897,.T.);
#26778=ORIENTED_EDGE('',*,*,#17894,.T.);
#26779=ORIENTED_EDGE('',*,*,#17891,.T.);
#26780=ORIENTED_EDGE('',*,*,#17888,.T.);
#26781=ORIENTED_EDGE('',*,*,#17885,.T.);
#26782=ORIENTED_EDGE('',*,*,#17882,.T.);
#26783=ORIENTED_EDGE('',*,*,#17731,.T.);
#26784=ORIENTED_EDGE('',*,*,#17765,.T.);
#26785=ORIENTED_EDGE('',*,*,#17762,.T.);
#26786=ORIENTED_EDGE('',*,*,#17759,.T.);
#26787=ORIENTED_EDGE('',*,*,#17756,.T.);
#26788=ORIENTED_EDGE('',*,*,#17753,.T.);
#26789=ORIENTED_EDGE('',*,*,#17750,.T.);
#26790=ORIENTED_EDGE('',*,*,#17747,.T.);
#26791=ORIENTED_EDGE('',*,*,#17744,.T.);
#26792=ORIENTED_EDGE('',*,*,#17741,.T.);
#26793=ORIENTED_EDGE('',*,*,#17738,.T.);
#26794=ORIENTED_EDGE('',*,*,#17735,.T.);
#26795=ORIENTED_EDGE('',*,*,#17554,.T.);
#26796=ORIENTED_EDGE('',*,*,#17618,.T.);
#26797=ORIENTED_EDGE('',*,*,#17615,.T.);
#26798=ORIENTED_EDGE('',*,*,#17612,.T.);
#26799=ORIENTED_EDGE('',*,*,#17609,.T.);
#26800=ORIENTED_EDGE('',*,*,#17606,.T.);
#26801=ORIENTED_EDGE('',*,*,#17603,.T.);
#26802=ORIENTED_EDGE('',*,*,#17600,.T.);
#26803=ORIENTED_EDGE('',*,*,#17597,.T.);
#26804=ORIENTED_EDGE('',*,*,#17594,.T.);
#26805=ORIENTED_EDGE('',*,*,#17591,.T.);
#26806=ORIENTED_EDGE('',*,*,#17588,.T.);
#26807=ORIENTED_EDGE('',*,*,#17585,.T.);
#26808=ORIENTED_EDGE('',*,*,#17582,.T.);
#26809=ORIENTED_EDGE('',*,*,#17579,.T.);
#26810=ORIENTED_EDGE('',*,*,#17576,.T.);
#26811=ORIENTED_EDGE('',*,*,#17573,.T.);
#26812=ORIENTED_EDGE('',*,*,#17570,.T.);
#26813=ORIENTED_EDGE('',*,*,#17567,.T.);
#26814=ORIENTED_EDGE('',*,*,#17564,.T.);
#26815=ORIENTED_EDGE('',*,*,#17561,.T.);
#26816=ORIENTED_EDGE('',*,*,#17558,.T.);
#26817=ORIENTED_EDGE('',*,*,#17518,.T.);
#26818=ORIENTED_EDGE('',*,*,#17552,.T.);
#26819=ORIENTED_EDGE('',*,*,#17549,.T.);
#26820=ORIENTED_EDGE('',*,*,#17546,.T.);
#26821=ORIENTED_EDGE('',*,*,#17543,.T.);
#26822=ORIENTED_EDGE('',*,*,#17540,.T.);
#26823=ORIENTED_EDGE('',*,*,#17537,.T.);
#26824=ORIENTED_EDGE('',*,*,#17534,.T.);
#26825=ORIENTED_EDGE('',*,*,#17531,.T.);
#26826=ORIENTED_EDGE('',*,*,#17528,.T.);
#26827=ORIENTED_EDGE('',*,*,#17525,.T.);
#26828=ORIENTED_EDGE('',*,*,#17522,.T.);
#26829=ORIENTED_EDGE('',*,*,#17311,.T.);
#26830=ORIENTED_EDGE('',*,*,#17342,.T.);
#26831=ORIENTED_EDGE('',*,*,#17339,.T.);
#26832=ORIENTED_EDGE('',*,*,#17336,.T.);
#26833=ORIENTED_EDGE('',*,*,#17333,.T.);
#26834=ORIENTED_EDGE('',*,*,#17330,.T.);
#26835=ORIENTED_EDGE('',*,*,#17327,.T.);
#26836=ORIENTED_EDGE('',*,*,#17324,.T.);
#26837=ORIENTED_EDGE('',*,*,#17321,.T.);
#26838=ORIENTED_EDGE('',*,*,#17318,.T.);
#26839=ORIENTED_EDGE('',*,*,#17315,.T.);
#26840=ORIENTED_EDGE('',*,*,#17266,.T.);
#26841=ORIENTED_EDGE('',*,*,#17300,.T.);
#26842=ORIENTED_EDGE('',*,*,#17297,.T.);
#26843=ORIENTED_EDGE('',*,*,#17294,.T.);
#26844=ORIENTED_EDGE('',*,*,#17291,.T.);
#26845=ORIENTED_EDGE('',*,*,#17288,.T.);
#26846=ORIENTED_EDGE('',*,*,#17285,.T.);
#26847=ORIENTED_EDGE('',*,*,#17282,.T.);
#26848=ORIENTED_EDGE('',*,*,#17279,.T.);
#26849=ORIENTED_EDGE('',*,*,#17276,.T.);
#26850=ORIENTED_EDGE('',*,*,#17273,.T.);
#26851=ORIENTED_EDGE('',*,*,#17270,.T.);
#26852=ORIENTED_EDGE('',*,*,#19280,.F.);
#26853=ORIENTED_EDGE('',*,*,#19258,.F.);
#26854=ORIENTED_EDGE('',*,*,#19262,.F.);
#26855=ORIENTED_EDGE('',*,*,#19265,.F.);
#26856=ORIENTED_EDGE('',*,*,#19268,.F.);
#26857=ORIENTED_EDGE('',*,*,#19271,.F.);
#26858=ORIENTED_EDGE('',*,*,#19274,.F.);
#26859=ORIENTED_EDGE('',*,*,#19277,.F.);
#26860=ORIENTED_EDGE('',*,*,#19252,.T.);
#26861=ORIENTED_EDGE('',*,*,#19255,.T.);
#30683=ADVANCED_FACE('',(#3708),#331,.F.);
#30684=ADVANCED_FACE('',(#3709),#332,.F.);
#30685=ADVANCED_FACE('',(#3710),#333,.F.);
#30686=ADVANCED_FACE('',(#3711),#334,.F.);
#30687=ADVANCED_FACE('',(#3712),#335,.F.);
#30688=ADVANCED_FACE('',(#3713),#336,.F.);
#30689=ADVANCED_FACE('',(#3714),#337,.F.);
#30690=ADVANCED_FACE('',(#3715),#338,.F.);
#30691=ADVANCED_FACE('',(#3716),#339,.F.);
#30692=ADVANCED_FACE('',(#3717),#340,.F.);
#30693=ADVANCED_FACE('',(#3718),#341,.F.);
#30694=ADVANCED_FACE('',(#3719),#342,.F.);
#30695=ADVANCED_FACE('',(#3720),#343,.F.);
#30696=ADVANCED_FACE('',(#3721),#344,.F.);
#30697=ADVANCED_FACE('',(#3722),#345,.F.);
#30698=ADVANCED_FACE('',(#3723),#346,.F.);
#30699=ADVANCED_FACE('',(#3724),#347,.F.);
#30700=ADVANCED_FACE('',(#3725),#348,.F.);
#30701=ADVANCED_FACE('',(#3726),#349,.F.);
#30702=ADVANCED_FACE('',(#3727),#350,.F.);
#30703=ADVANCED_FACE('',(#3728,#2078),#2450,.T.);
#30704=ADVANCED_FACE('',(#3729),#2451,.F.);
#30705=ADVANCED_FACE('',(#3730),#2452,.F.);
#30706=ADVANCED_FACE('',(#3731),#2453,.F.);
#30707=ADVANCED_FACE('',(#3732),#2454,.F.);
#30708=ADVANCED_FACE('',(#3733),#2455,.F.);
#30709=ADVANCED_FACE('',(#3734),#2456,.F.);
#30710=ADVANCED_FACE('',(#3735),#2457,.F.);
#30711=ADVANCED_FACE('',(#3736),#2458,.F.);
#30712=ADVANCED_FACE('',(#3737),#2459,.F.);
#30713=ADVANCED_FACE('',(#3738),#2460,.F.);
#30714=ADVANCED_FACE('',(#3739),#2461,.F.);
#30715=ADVANCED_FACE('',(#3740),#2462,.F.);
#30716=ADVANCED_FACE('',(#3741),#2463,.F.);
#30717=ADVANCED_FACE('',(#3742),#2464,.F.);
#30718=ADVANCED_FACE('',(#3743,#2079),#2465,.F.);
#30719=ADVANCED_FACE('',(#3744),#2466,.T.);
#30720=ADVANCED_FACE('',(#3745),#2467,.T.);
#30721=ADVANCED_FACE('',(#3746),#351,.F.);
#30722=ADVANCED_FACE('',(#3747),#352,.F.);
#30723=ADVANCED_FACE('',(#3748),#353,.F.);
#30724=ADVANCED_FACE('',(#3749),#354,.F.);
#30725=ADVANCED_FACE('',(#3750),#355,.F.);
#30726=ADVANCED_FACE('',(#3751),#356,.F.);
#30727=ADVANCED_FACE('',(#3752),#357,.F.);
#30728=ADVANCED_FACE('',(#3753),#358,.F.);
#30729=ADVANCED_FACE('',(#3754),#359,.F.);
#30730=ADVANCED_FACE('',(#3755),#360,.F.);
#30731=ADVANCED_FACE('',(#3756),#361,.F.);
#30732=ADVANCED_FACE('',(#3757),#362,.F.);
#30733=ADVANCED_FACE('',(#3758),#363,.F.);
#30734=ADVANCED_FACE('',(#3759),#364,.F.);
#30735=ADVANCED_FACE('',(#3760),#365,.F.);
#30736=ADVANCED_FACE('',(#3761),#366,.F.);
#30737=ADVANCED_FACE('',(#3762),#367,.F.);
#30738=ADVANCED_FACE('',(#3763),#368,.F.);
#30739=ADVANCED_FACE('',(#3764),#369,.F.);
#30740=ADVANCED_FACE('',(#3765),#370,.F.);
#30741=ADVANCED_FACE('',(#3766,#2080),#2468,.T.);
#30742=ADVANCED_FACE('',(#3767),#371,.F.);
#30743=ADVANCED_FACE('',(#3768),#372,.F.);
#30744=ADVANCED_FACE('',(#3769),#373,.F.);
#30745=ADVANCED_FACE('',(#3770),#374,.F.);
#30746=ADVANCED_FACE('',(#3771),#375,.F.);
#30747=ADVANCED_FACE('',(#3772),#376,.F.);
#30748=ADVANCED_FACE('',(#3773),#377,.F.);
#30749=ADVANCED_FACE('',(#3774),#378,.F.);
#30750=ADVANCED_FACE('',(#3775),#379,.F.);
#30751=ADVANCED_FACE('',(#3776),#380,.F.);
#30752=ADVANCED_FACE('',(#3777),#381,.F.);
#30753=ADVANCED_FACE('',(#3778),#382,.F.);
#30754=ADVANCED_FACE('',(#3779),#2469,.F.);
#30755=ADVANCED_FACE('',(#3780),#383,.F.);
#30756=ADVANCED_FACE('',(#3781),#384,.F.);
#30757=ADVANCED_FACE('',(#3782),#385,.F.);
#30758=ADVANCED_FACE('',(#3783),#386,.F.);
#30759=ADVANCED_FACE('',(#3784),#387,.F.);
#30760=ADVANCED_FACE('',(#3785),#388,.F.);
#30761=ADVANCED_FACE('',(#3786),#389,.F.);
#30762=ADVANCED_FACE('',(#3787),#2470,.F.);
#30763=ADVANCED_FACE('',(#3788),#390,.F.);
#30764=ADVANCED_FACE('',(#3789),#391,.F.);
#30765=ADVANCED_FACE('',(#3790),#392,.F.);
#30766=ADVANCED_FACE('',(#3791),#393,.F.);
#30767=ADVANCED_FACE('',(#3792),#394,.F.);
#30768=ADVANCED_FACE('',(#3793),#395,.F.);
#30769=ADVANCED_FACE('',(#3794),#396,.F.);
#30770=ADVANCED_FACE('',(#3795),#2471,.F.);
#30771=ADVANCED_FACE('',(#3796),#397,.F.);
#30772=ADVANCED_FACE('',(#3797),#2472,.T.);
#30773=ADVANCED_FACE('',(#3798),#2473,.T.);
#30774=ADVANCED_FACE('',(#3799),#398,.F.);
#30775=ADVANCED_FACE('',(#3800),#399,.F.);
#30776=ADVANCED_FACE('',(#3801),#400,.F.);
#30777=ADVANCED_FACE('',(#3802),#401,.F.);
#30778=ADVANCED_FACE('',(#3803),#402,.F.);
#30779=ADVANCED_FACE('',(#3804),#403,.F.);
#30780=ADVANCED_FACE('',(#3805),#404,.F.);
#30781=ADVANCED_FACE('',(#3806),#405,.F.);
#30782=ADVANCED_FACE('',(#3807),#406,.F.);
#30783=ADVANCED_FACE('',(#3808),#407,.F.);
#30784=ADVANCED_FACE('',(#3809),#408,.F.);
#30785=ADVANCED_FACE('',(#3810),#409,.F.);
#30786=ADVANCED_FACE('',(#3811),#410,.F.);
#30787=ADVANCED_FACE('',(#3812),#411,.F.);
#30788=ADVANCED_FACE('',(#3813),#412,.F.);
#30789=ADVANCED_FACE('',(#3814),#413,.F.);
#30790=ADVANCED_FACE('',(#3815),#414,.F.);
#30791=ADVANCED_FACE('',(#3816),#415,.F.);
#30792=ADVANCED_FACE('',(#3817),#416,.F.);
#30793=ADVANCED_FACE('',(#3818),#417,.F.);
#30794=ADVANCED_FACE('',(#3819,#2081),#2474,.T.);
#30795=ADVANCED_FACE('',(#3820),#418,.F.);
#30796=ADVANCED_FACE('',(#3821),#419,.F.);
#30797=ADVANCED_FACE('',(#3822),#420,.F.);
#30798=ADVANCED_FACE('',(#3823),#421,.F.);
#30799=ADVANCED_FACE('',(#3824),#422,.F.);
#30800=ADVANCED_FACE('',(#3825),#423,.F.);
#30801=ADVANCED_FACE('',(#3826),#424,.F.);
#30802=ADVANCED_FACE('',(#3827),#425,.F.);
#30803=ADVANCED_FACE('',(#3828),#426,.F.);
#30804=ADVANCED_FACE('',(#3829),#2475,.F.);
#30805=ADVANCED_FACE('',(#3830),#427,.F.);
#30806=ADVANCED_FACE('',(#3831),#428,.F.);
#30807=ADVANCED_FACE('',(#3832),#429,.F.);
#30808=ADVANCED_FACE('',(#3833),#430,.F.);
#30809=ADVANCED_FACE('',(#3834),#431,.F.);
#30810=ADVANCED_FACE('',(#3835),#432,.F.);
#30811=ADVANCED_FACE('',(#3836),#433,.F.);
#30812=ADVANCED_FACE('',(#3837),#434,.F.);
#30813=ADVANCED_FACE('',(#3838),#435,.F.);
#30814=ADVANCED_FACE('',(#3839),#2476,.F.);
#30815=ADVANCED_FACE('',(#3840),#2477,.F.);
#30816=ADVANCED_FACE('',(#3841),#2478,.F.);
#30817=ADVANCED_FACE('',(#3842),#2479,.T.);
#30818=ADVANCED_FACE('',(#3843),#2480,.T.);
#30819=ADVANCED_FACE('',(#3844),#436,.F.);
#30820=ADVANCED_FACE('',(#3845),#437,.F.);
#30821=ADVANCED_FACE('',(#3846),#438,.F.);
#30822=ADVANCED_FACE('',(#3847),#439,.F.);
#30823=ADVANCED_FACE('',(#3848),#440,.F.);
#30824=ADVANCED_FACE('',(#3849),#441,.F.);
#30825=ADVANCED_FACE('',(#3850),#442,.F.);
#30826=ADVANCED_FACE('',(#3851),#443,.F.);
#30827=ADVANCED_FACE('',(#3852),#444,.F.);
#30828=ADVANCED_FACE('',(#3853),#445,.F.);
#30829=ADVANCED_FACE('',(#3854),#446,.F.);
#30830=ADVANCED_FACE('',(#3855),#447,.F.);
#30831=ADVANCED_FACE('',(#3856),#448,.F.);
#30832=ADVANCED_FACE('',(#3857),#449,.F.);
#30833=ADVANCED_FACE('',(#3858),#450,.F.);
#30834=ADVANCED_FACE('',(#3859),#451,.F.);
#30835=ADVANCED_FACE('',(#3860),#452,.F.);
#30836=ADVANCED_FACE('',(#3861),#453,.F.);
#30837=ADVANCED_FACE('',(#3862),#454,.F.);
#30838=ADVANCED_FACE('',(#3863),#455,.F.);
#30839=ADVANCED_FACE('',(#3864,#2082),#2481,.T.);
#30840=ADVANCED_FACE('',(#3865),#2482,.F.);
#30841=ADVANCED_FACE('',(#3866),#456,.F.);
#30842=ADVANCED_FACE('',(#3867),#457,.F.);
#30843=ADVANCED_FACE('',(#3868),#2483,.F.);
#30844=ADVANCED_FACE('',(#3869),#458,.F.);
#30845=ADVANCED_FACE('',(#3870),#459,.F.);
#30846=ADVANCED_FACE('',(#3871),#2484,.F.);
#30847=ADVANCED_FACE('',(#3872),#2485,.F.);
#30848=ADVANCED_FACE('',(#3873),#2486,.F.);
#30849=ADVANCED_FACE('',(#3874),#2487,.T.);
#30850=ADVANCED_FACE('',(#3875),#2488,.T.);
#30851=ADVANCED_FACE('',(#3876),#460,.F.);
#30852=ADVANCED_FACE('',(#3877),#461,.F.);
#30853=ADVANCED_FACE('',(#3878),#462,.F.);
#30854=ADVANCED_FACE('',(#3879),#463,.F.);
#30855=ADVANCED_FACE('',(#3880),#464,.F.);
#30856=ADVANCED_FACE('',(#3881),#465,.F.);
#30857=ADVANCED_FACE('',(#3882),#466,.F.);
#30858=ADVANCED_FACE('',(#3883),#467,.F.);
#30859=ADVANCED_FACE('',(#3884),#468,.F.);
#30860=ADVANCED_FACE('',(#3885),#469,.F.);
#30861=ADVANCED_FACE('',(#3886),#470,.F.);
#30862=ADVANCED_FACE('',(#3887),#471,.F.);
#30863=ADVANCED_FACE('',(#3888),#472,.F.);
#30864=ADVANCED_FACE('',(#3889),#473,.F.);
#30865=ADVANCED_FACE('',(#3890),#474,.F.);
#30866=ADVANCED_FACE('',(#3891),#475,.F.);
#30867=ADVANCED_FACE('',(#3892),#476,.F.);
#30868=ADVANCED_FACE('',(#3893),#477,.F.);
#30869=ADVANCED_FACE('',(#3894),#478,.F.);
#30870=ADVANCED_FACE('',(#3895),#479,.F.);
#30871=ADVANCED_FACE('',(#3896,#2083),#2489,.T.);
#30872=ADVANCED_FACE('',(#3897),#2490,.T.);
#30873=ADVANCED_FACE('',(#3898),#480,.F.);
#30874=ADVANCED_FACE('',(#3899),#481,.F.);
#30875=ADVANCED_FACE('',(#3900),#482,.F.);
#30876=ADVANCED_FACE('',(#3901),#483,.F.);
#30877=ADVANCED_FACE('',(#3902),#484,.F.);
#30878=ADVANCED_FACE('',(#3903),#485,.F.);
#30879=ADVANCED_FACE('',(#3904),#486,.F.);
#30880=ADVANCED_FACE('',(#3905),#487,.F.);
#30881=ADVANCED_FACE('',(#3906),#488,.F.);
#30882=ADVANCED_FACE('',(#3907),#489,.F.);
#30883=ADVANCED_FACE('',(#3908),#490,.F.);
#30884=ADVANCED_FACE('',(#3909),#491,.F.);
#30885=ADVANCED_FACE('',(#3910),#492,.F.);
#30886=ADVANCED_FACE('',(#3911),#493,.F.);
#30887=ADVANCED_FACE('',(#3912),#494,.F.);
#30888=ADVANCED_FACE('',(#3913),#495,.F.);
#30889=ADVANCED_FACE('',(#3914),#496,.F.);
#30890=ADVANCED_FACE('',(#3915),#497,.F.);
#30891=ADVANCED_FACE('',(#3916),#498,.F.);
#30892=ADVANCED_FACE('',(#3917),#499,.F.);
#30893=ADVANCED_FACE('',(#3918,#2084),#2491,.T.);
#30894=ADVANCED_FACE('',(#3919),#2492,.F.);
#30895=ADVANCED_FACE('',(#3920),#500,.F.);
#30896=ADVANCED_FACE('',(#3921),#501,.F.);
#30897=ADVANCED_FACE('',(#3922),#2493,.F.);
#30898=ADVANCED_FACE('',(#3923),#502,.F.);
#30899=ADVANCED_FACE('',(#3924),#503,.F.);
#30900=ADVANCED_FACE('',(#3925),#2494,.F.);
#30901=ADVANCED_FACE('',(#3926),#2495,.F.);
#30902=ADVANCED_FACE('',(#3927),#2496,.F.);
#30903=ADVANCED_FACE('',(#3928),#2497,.T.);
#30904=ADVANCED_FACE('',(#3929),#2498,.T.);
#30905=ADVANCED_FACE('',(#3930),#504,.F.);
#30906=ADVANCED_FACE('',(#3931),#505,.F.);
#30907=ADVANCED_FACE('',(#3932),#506,.F.);
#30908=ADVANCED_FACE('',(#3933),#507,.F.);
#30909=ADVANCED_FACE('',(#3934),#508,.F.);
#30910=ADVANCED_FACE('',(#3935),#509,.F.);
#30911=ADVANCED_FACE('',(#3936),#510,.F.);
#30912=ADVANCED_FACE('',(#3937),#511,.F.);
#30913=ADVANCED_FACE('',(#3938),#512,.F.);
#30914=ADVANCED_FACE('',(#3939),#513,.F.);
#30915=ADVANCED_FACE('',(#3940),#514,.F.);
#30916=ADVANCED_FACE('',(#3941),#515,.F.);
#30917=ADVANCED_FACE('',(#3942),#516,.F.);
#30918=ADVANCED_FACE('',(#3943),#517,.F.);
#30919=ADVANCED_FACE('',(#3944),#518,.F.);
#30920=ADVANCED_FACE('',(#3945),#519,.F.);
#30921=ADVANCED_FACE('',(#3946),#520,.F.);
#30922=ADVANCED_FACE('',(#3947),#521,.F.);
#30923=ADVANCED_FACE('',(#3948),#522,.F.);
#30924=ADVANCED_FACE('',(#3949),#523,.F.);
#30925=ADVANCED_FACE('',(#3950,#2085),#2499,.T.);
#30926=ADVANCED_FACE('',(#3951),#524,.F.);
#30927=ADVANCED_FACE('',(#3952),#525,.F.);
#30928=ADVANCED_FACE('',(#3953),#526,.F.);
#30929=ADVANCED_FACE('',(#3954),#527,.F.);
#30930=ADVANCED_FACE('',(#3955),#528,.F.);
#30931=ADVANCED_FACE('',(#3956),#529,.F.);
#30932=ADVANCED_FACE('',(#3957),#530,.F.);
#30933=ADVANCED_FACE('',(#3958),#531,.F.);
#30934=ADVANCED_FACE('',(#3959),#532,.F.);
#30935=ADVANCED_FACE('',(#3960),#2500,.F.);
#30936=ADVANCED_FACE('',(#3961),#533,.F.);
#30937=ADVANCED_FACE('',(#3962),#534,.F.);
#30938=ADVANCED_FACE('',(#3963),#535,.F.);
#30939=ADVANCED_FACE('',(#3964),#536,.F.);
#30940=ADVANCED_FACE('',(#3965),#537,.F.);
#30941=ADVANCED_FACE('',(#3966),#538,.F.);
#30942=ADVANCED_FACE('',(#3967),#539,.F.);
#30943=ADVANCED_FACE('',(#3968),#540,.F.);
#30944=ADVANCED_FACE('',(#3969),#541,.F.);
#30945=ADVANCED_FACE('',(#3970),#2501,.F.);
#30946=ADVANCED_FACE('',(#3971),#2502,.F.);
#30947=ADVANCED_FACE('',(#3972),#2503,.F.);
#30948=ADVANCED_FACE('',(#3973),#2504,.T.);
#30949=ADVANCED_FACE('',(#3974),#2505,.T.);
#30950=ADVANCED_FACE('',(#3975),#542,.F.);
#30951=ADVANCED_FACE('',(#3976),#543,.F.);
#30952=ADVANCED_FACE('',(#3977),#544,.F.);
#30953=ADVANCED_FACE('',(#3978),#545,.F.);
#30954=ADVANCED_FACE('',(#3979),#546,.F.);
#30955=ADVANCED_FACE('',(#3980),#547,.F.);
#30956=ADVANCED_FACE('',(#3981),#548,.F.);
#30957=ADVANCED_FACE('',(#3982),#549,.F.);
#30958=ADVANCED_FACE('',(#3983),#550,.F.);
#30959=ADVANCED_FACE('',(#3984),#551,.F.);
#30960=ADVANCED_FACE('',(#3985),#552,.F.);
#30961=ADVANCED_FACE('',(#3986),#553,.F.);
#30962=ADVANCED_FACE('',(#3987),#554,.F.);
#30963=ADVANCED_FACE('',(#3988),#555,.F.);
#30964=ADVANCED_FACE('',(#3989),#556,.F.);
#30965=ADVANCED_FACE('',(#3990),#557,.F.);
#30966=ADVANCED_FACE('',(#3991),#558,.F.);
#30967=ADVANCED_FACE('',(#3992),#559,.F.);
#30968=ADVANCED_FACE('',(#3993),#560,.F.);
#30969=ADVANCED_FACE('',(#3994),#561,.F.);
#30970=ADVANCED_FACE('',(#3995,#2086),#2506,.T.);
#30971=ADVANCED_FACE('',(#3996),#562,.F.);
#30972=ADVANCED_FACE('',(#3997),#563,.F.);
#30973=ADVANCED_FACE('',(#3998),#564,.F.);
#30974=ADVANCED_FACE('',(#3999),#565,.F.);
#30975=ADVANCED_FACE('',(#4000),#566,.F.);
#30976=ADVANCED_FACE('',(#4001),#567,.F.);
#30977=ADVANCED_FACE('',(#4002),#568,.F.);
#30978=ADVANCED_FACE('',(#4003),#569,.F.);
#30979=ADVANCED_FACE('',(#4004),#570,.F.);
#30980=ADVANCED_FACE('',(#4005),#571,.F.);
#30981=ADVANCED_FACE('',(#4006),#572,.F.);
#30982=ADVANCED_FACE('',(#4007),#573,.F.);
#30983=ADVANCED_FACE('',(#4008),#2507,.F.);
#30984=ADVANCED_FACE('',(#4009),#574,.F.);
#30985=ADVANCED_FACE('',(#4010),#575,.F.);
#30986=ADVANCED_FACE('',(#4011),#576,.F.);
#30987=ADVANCED_FACE('',(#4012),#577,.F.);
#30988=ADVANCED_FACE('',(#4013),#578,.F.);
#30989=ADVANCED_FACE('',(#4014),#579,.F.);
#30990=ADVANCED_FACE('',(#4015),#580,.F.);
#30991=ADVANCED_FACE('',(#4016),#2508,.F.);
#30992=ADVANCED_FACE('',(#4017),#581,.F.);
#30993=ADVANCED_FACE('',(#4018),#582,.F.);
#30994=ADVANCED_FACE('',(#4019),#583,.F.);
#30995=ADVANCED_FACE('',(#4020),#584,.F.);
#30996=ADVANCED_FACE('',(#4021),#585,.F.);
#30997=ADVANCED_FACE('',(#4022),#586,.F.);
#30998=ADVANCED_FACE('',(#4023),#587,.F.);
#30999=ADVANCED_FACE('',(#4024),#2509,.F.);
#31000=ADVANCED_FACE('',(#4025),#588,.F.);
#31001=ADVANCED_FACE('',(#4026),#2510,.T.);
#31002=ADVANCED_FACE('',(#4027),#2511,.T.);
#31003=ADVANCED_FACE('',(#4028),#589,.F.);
#31004=ADVANCED_FACE('',(#4029),#590,.F.);
#31005=ADVANCED_FACE('',(#4030),#591,.F.);
#31006=ADVANCED_FACE('',(#4031),#592,.F.);
#31007=ADVANCED_FACE('',(#4032),#593,.F.);
#31008=ADVANCED_FACE('',(#4033),#594,.F.);
#31009=ADVANCED_FACE('',(#4034),#595,.F.);
#31010=ADVANCED_FACE('',(#4035),#596,.F.);
#31011=ADVANCED_FACE('',(#4036),#597,.F.);
#31012=ADVANCED_FACE('',(#4037),#598,.F.);
#31013=ADVANCED_FACE('',(#4038),#599,.F.);
#31014=ADVANCED_FACE('',(#4039),#600,.F.);
#31015=ADVANCED_FACE('',(#4040),#601,.F.);
#31016=ADVANCED_FACE('',(#4041),#602,.F.);
#31017=ADVANCED_FACE('',(#4042),#603,.F.);
#31018=ADVANCED_FACE('',(#4043),#604,.F.);
#31019=ADVANCED_FACE('',(#4044),#605,.F.);
#31020=ADVANCED_FACE('',(#4045),#606,.F.);
#31021=ADVANCED_FACE('',(#4046),#607,.F.);
#31022=ADVANCED_FACE('',(#4047),#608,.F.);
#31023=ADVANCED_FACE('',(#4048,#2087),#2512,.T.);
#31024=ADVANCED_FACE('',(#4049),#2513,.F.);
#31025=ADVANCED_FACE('',(#4050),#2514,.F.);
#31026=ADVANCED_FACE('',(#4051),#2515,.F.);
#31027=ADVANCED_FACE('',(#4052),#2516,.F.);
#31028=ADVANCED_FACE('',(#4053),#2517,.F.);
#31029=ADVANCED_FACE('',(#4054),#2518,.F.);
#31030=ADVANCED_FACE('',(#4055),#2519,.F.);
#31031=ADVANCED_FACE('',(#4056),#2520,.F.);
#31032=ADVANCED_FACE('',(#4057),#2521,.F.);
#31033=ADVANCED_FACE('',(#4058),#2522,.F.);
#31034=ADVANCED_FACE('',(#4059),#2523,.F.);
#31035=ADVANCED_FACE('',(#4060),#2524,.F.);
#31036=ADVANCED_FACE('',(#4061),#2525,.F.);
#31037=ADVANCED_FACE('',(#4062),#2526,.F.);
#31038=ADVANCED_FACE('',(#4063,#2088),#2527,.F.);
#31039=ADVANCED_FACE('',(#4064),#2528,.T.);
#31040=ADVANCED_FACE('',(#4065),#2529,.T.);
#31041=ADVANCED_FACE('',(#4066),#2530,.F.);
#31042=ADVANCED_FACE('',(#4067),#2531,.F.);
#31043=ADVANCED_FACE('',(#4068),#2532,.F.);
#31044=ADVANCED_FACE('',(#4069),#2533,.F.);
#31045=ADVANCED_FACE('',(#4070),#2534,.F.);
#31046=ADVANCED_FACE('',(#4071),#2535,.F.);
#31047=ADVANCED_FACE('',(#4072),#2536,.F.);
#31048=ADVANCED_FACE('',(#4073),#2537,.F.);
#31049=ADVANCED_FACE('',(#4074),#2538,.F.);
#31050=ADVANCED_FACE('',(#4075),#2539,.F.);
#31051=ADVANCED_FACE('',(#4076),#2540,.F.);
#31052=ADVANCED_FACE('',(#4077),#2541,.F.);
#31053=ADVANCED_FACE('',(#4078),#2542,.F.);
#31054=ADVANCED_FACE('',(#4079),#2543,.F.);
#31055=ADVANCED_FACE('',(#4080),#2544,.F.);
#31056=ADVANCED_FACE('',(#4081),#2545,.F.);
#31057=ADVANCED_FACE('',(#4082),#2546,.F.);
#31058=ADVANCED_FACE('',(#4083),#2547,.F.);
#31059=ADVANCED_FACE('',(#4084),#2548,.F.);
#31060=ADVANCED_FACE('',(#4085),#2549,.F.);
#31061=ADVANCED_FACE('',(#4086),#2550,.F.);
#31062=ADVANCED_FACE('',(#4087),#2551,.F.);
#31063=ADVANCED_FACE('',(#4088),#2552,.F.);
#31064=ADVANCED_FACE('',(#4089),#2553,.F.);
#31065=ADVANCED_FACE('',(#4090),#2554,.F.);
#31066=ADVANCED_FACE('',(#4091),#2555,.F.);
#31067=ADVANCED_FACE('',(#4092),#2556,.F.);
#31068=ADVANCED_FACE('',(#4093),#2557,.F.);
#31069=ADVANCED_FACE('',(#4094),#2558,.F.);
#31070=ADVANCED_FACE('',(#4095),#2559,.F.);
#31071=ADVANCED_FACE('',(#4096),#2560,.F.);
#31072=ADVANCED_FACE('',(#4097),#2561,.F.);
#31073=ADVANCED_FACE('',(#4098),#2562,.F.);
#31074=ADVANCED_FACE('',(#4099),#2563,.F.);
#31075=ADVANCED_FACE('',(#4100),#2564,.F.);
#31076=ADVANCED_FACE('',(#4101),#2565,.F.);
#31077=ADVANCED_FACE('',(#4102),#2566,.F.);
#31078=ADVANCED_FACE('',(#4103),#2567,.F.);
#31079=ADVANCED_FACE('',(#4104),#2568,.F.);
#31080=ADVANCED_FACE('',(#4105),#2569,.F.);
#31081=ADVANCED_FACE('',(#4106),#2570,.F.);
#31082=ADVANCED_FACE('',(#4107),#2571,.F.);
#31083=ADVANCED_FACE('',(#4108),#2572,.F.);
#31084=ADVANCED_FACE('',(#4109),#2573,.F.);
#31085=ADVANCED_FACE('',(#4110),#2574,.F.);
#31086=ADVANCED_FACE('',(#4111),#2575,.F.);
#31087=ADVANCED_FACE('',(#4112),#2576,.F.);
#31088=ADVANCED_FACE('',(#4113),#2577,.F.);
#31089=ADVANCED_FACE('',(#4114),#2578,.F.);
#31090=ADVANCED_FACE('',(#4115),#2579,.F.);
#31091=ADVANCED_FACE('',(#4116),#2580,.F.);
#31092=ADVANCED_FACE('',(#4117),#2581,.F.);
#31093=ADVANCED_FACE('',(#4118),#2582,.F.);
#31094=ADVANCED_FACE('',(#4119),#2583,.F.);
#31095=ADVANCED_FACE('',(#4120),#2584,.F.);
#31096=ADVANCED_FACE('',(#4121),#2585,.F.);
#31097=ADVANCED_FACE('',(#4122),#2586,.F.);
#31098=ADVANCED_FACE('',(#4123),#2587,.F.);
#31099=ADVANCED_FACE('',(#4124),#2588,.F.);
#31100=ADVANCED_FACE('',(#4125),#2589,.F.);
#31101=ADVANCED_FACE('',(#4126),#2590,.F.);
#31102=ADVANCED_FACE('',(#4127),#2591,.F.);
#31103=ADVANCED_FACE('',(#4128),#2592,.F.);
#31104=ADVANCED_FACE('',(#4129),#2593,.F.);
#31105=ADVANCED_FACE('',(#4130),#2594,.F.);
#31106=ADVANCED_FACE('',(#4131),#2595,.F.);
#31107=ADVANCED_FACE('',(#4132),#2596,.F.);
#31108=ADVANCED_FACE('',(#4133),#2597,.F.);
#31109=ADVANCED_FACE('',(#4134),#2598,.F.);
#31110=ADVANCED_FACE('',(#4135),#2599,.F.);
#31111=ADVANCED_FACE('',(#4136),#2600,.F.);
#31112=ADVANCED_FACE('',(#4137),#2601,.F.);
#31113=ADVANCED_FACE('',(#4138),#2602,.F.);
#31114=ADVANCED_FACE('',(#4139),#2603,.F.);
#31115=ADVANCED_FACE('',(#4140),#2604,.F.);
#31116=ADVANCED_FACE('',(#4141),#2605,.F.);
#31117=ADVANCED_FACE('',(#4142),#2606,.F.);
#31118=ADVANCED_FACE('',(#4143),#2607,.F.);
#31119=ADVANCED_FACE('',(#4144),#2608,.F.);
#31120=ADVANCED_FACE('',(#4145),#2609,.F.);
#31121=ADVANCED_FACE('',(#4146),#2610,.F.);
#31122=ADVANCED_FACE('',(#4147),#2611,.F.);
#31123=ADVANCED_FACE('',(#4148),#2612,.F.);
#31124=ADVANCED_FACE('',(#4149),#2613,.F.);
#31125=ADVANCED_FACE('',(#4150),#2614,.F.);
#31126=ADVANCED_FACE('',(#4151),#2615,.F.);
#31127=ADVANCED_FACE('',(#4152),#2616,.F.);
#31128=ADVANCED_FACE('',(#4153),#2617,.F.);
#31129=ADVANCED_FACE('',(#4154),#2618,.F.);
#31130=ADVANCED_FACE('',(#4155),#2619,.F.);
#31131=ADVANCED_FACE('',(#4156),#2620,.F.);
#31132=ADVANCED_FACE('',(#4157),#2621,.F.);
#31133=ADVANCED_FACE('',(#4158),#2622,.F.);
#31134=ADVANCED_FACE('',(#4159),#2623,.F.);
#31135=ADVANCED_FACE('',(#4160),#2624,.F.);
#31136=ADVANCED_FACE('',(#4161),#2625,.F.);
#31137=ADVANCED_FACE('',(#4162),#2626,.F.);
#31138=ADVANCED_FACE('',(#4163),#2627,.F.);
#31139=ADVANCED_FACE('',(#4164),#2628,.F.);
#31140=ADVANCED_FACE('',(#4165),#2629,.F.);
#31141=ADVANCED_FACE('',(#4166),#2630,.F.);
#31142=ADVANCED_FACE('',(#4167),#2631,.F.);
#31143=ADVANCED_FACE('',(#4168),#2632,.F.);
#31144=ADVANCED_FACE('',(#4169),#2633,.F.);
#31145=ADVANCED_FACE('',(#4170),#2634,.F.);
#31146=ADVANCED_FACE('',(#4171),#2635,.F.);
#31147=ADVANCED_FACE('',(#4172),#2636,.F.);
#31148=ADVANCED_FACE('',(#4173),#2637,.F.);
#31149=ADVANCED_FACE('',(#4174),#2638,.F.);
#31150=ADVANCED_FACE('',(#4175),#2639,.F.);
#31151=ADVANCED_FACE('',(#4176),#2640,.F.);
#31152=ADVANCED_FACE('',(#4177),#2641,.F.);
#31153=ADVANCED_FACE('',(#4178),#2642,.F.);
#31154=ADVANCED_FACE('',(#4179),#2643,.F.);
#31155=ADVANCED_FACE('',(#4180),#2644,.F.);
#31156=ADVANCED_FACE('',(#4181),#2645,.F.);
#31157=ADVANCED_FACE('',(#4182),#2646,.F.);
#31158=ADVANCED_FACE('',(#4183),#2647,.F.);
#31159=ADVANCED_FACE('',(#4184),#2648,.F.);
#31160=ADVANCED_FACE('',(#4185),#2649,.F.);
#31161=ADVANCED_FACE('',(#4186),#2650,.F.);
#31162=ADVANCED_FACE('',(#4187),#2651,.F.);
#31163=ADVANCED_FACE('',(#4188),#2652,.F.);
#31164=ADVANCED_FACE('',(#4189),#2653,.F.);
#31165=ADVANCED_FACE('',(#4190),#2654,.F.);
#31166=ADVANCED_FACE('',(#4191),#2655,.F.);
#31167=ADVANCED_FACE('',(#4192),#2656,.F.);
#31168=ADVANCED_FACE('',(#4193),#2657,.F.);
#31169=ADVANCED_FACE('',(#4194),#2658,.F.);
#31170=ADVANCED_FACE('',(#4195),#2659,.F.);
#31171=ADVANCED_FACE('',(#4196),#2660,.F.);
#31172=ADVANCED_FACE('',(#4197),#2661,.F.);
#31173=ADVANCED_FACE('',(#4198),#2662,.F.);
#31174=ADVANCED_FACE('',(#4199),#2663,.F.);
#31175=ADVANCED_FACE('',(#4200),#2664,.F.);
#31176=ADVANCED_FACE('',(#4201),#2665,.F.);
#31177=ADVANCED_FACE('',(#4202),#2666,.F.);
#31178=ADVANCED_FACE('',(#4203),#2667,.F.);
#31179=ADVANCED_FACE('',(#4204),#2668,.F.);
#31180=ADVANCED_FACE('',(#4205),#2669,.F.);
#31181=ADVANCED_FACE('',(#4206),#2670,.F.);
#31182=ADVANCED_FACE('',(#4207),#2671,.F.);
#31183=ADVANCED_FACE('',(#4208),#2672,.F.);
#31184=ADVANCED_FACE('',(#4209),#2673,.F.);
#31185=ADVANCED_FACE('',(#4210),#2674,.F.);
#31186=ADVANCED_FACE('',(#4211),#2675,.F.);
#31187=ADVANCED_FACE('',(#4212),#2676,.F.);
#31188=ADVANCED_FACE('',(#4213),#2677,.F.);
#31189=ADVANCED_FACE('',(#4214),#2678,.F.);
#31190=ADVANCED_FACE('',(#4215),#2679,.F.);
#31191=ADVANCED_FACE('',(#4216),#2680,.F.);
#31192=ADVANCED_FACE('',(#4217),#2681,.F.);
#31193=ADVANCED_FACE('',(#4218),#2682,.F.);
#31194=ADVANCED_FACE('',(#4219),#2683,.F.);
#31195=ADVANCED_FACE('',(#4220),#2684,.F.);
#31196=ADVANCED_FACE('',(#4221),#2685,.F.);
#31197=ADVANCED_FACE('',(#4222),#2686,.F.);
#31198=ADVANCED_FACE('',(#4223),#2687,.F.);
#31199=ADVANCED_FACE('',(#4224),#2688,.F.);
#31200=ADVANCED_FACE('',(#4225),#2689,.F.);
#31201=ADVANCED_FACE('',(#4226),#2690,.F.);
#31202=ADVANCED_FACE('',(#4227),#2691,.F.);
#31203=ADVANCED_FACE('',(#4228),#2692,.F.);
#31204=ADVANCED_FACE('',(#4229),#2693,.F.);
#31205=ADVANCED_FACE('',(#4230),#2694,.F.);
#31206=ADVANCED_FACE('',(#4231),#2695,.F.);
#31207=ADVANCED_FACE('',(#4232),#2696,.F.);
#31208=ADVANCED_FACE('',(#4233),#2697,.F.);
#31209=ADVANCED_FACE('',(#4234),#2698,.F.);
#31210=ADVANCED_FACE('',(#4235),#2699,.F.);
#31211=ADVANCED_FACE('',(#4236),#2700,.F.);
#31212=ADVANCED_FACE('',(#4237),#2701,.F.);
#31213=ADVANCED_FACE('',(#4238),#2702,.F.);
#31214=ADVANCED_FACE('',(#4239),#2703,.F.);
#31215=ADVANCED_FACE('',(#4240),#2704,.F.);
#31216=ADVANCED_FACE('',(#4241),#2705,.F.);
#31217=ADVANCED_FACE('',(#4242),#2706,.F.);
#31218=ADVANCED_FACE('',(#4243),#2707,.F.);
#31219=ADVANCED_FACE('',(#4244),#2708,.F.);
#31220=ADVANCED_FACE('',(#4245),#2709,.F.);
#31221=ADVANCED_FACE('',(#4246),#2710,.F.);
#31222=ADVANCED_FACE('',(#4247),#2711,.F.);
#31223=ADVANCED_FACE('',(#4248),#2712,.F.);
#31224=ADVANCED_FACE('',(#4249),#2713,.F.);
#31225=ADVANCED_FACE('',(#4250),#2714,.F.);
#31226=ADVANCED_FACE('',(#4251),#2715,.F.);
#31227=ADVANCED_FACE('',(#4252),#2716,.F.);
#31228=ADVANCED_FACE('',(#4253),#2717,.F.);
#31229=ADVANCED_FACE('',(#4254),#2718,.F.);
#31230=ADVANCED_FACE('',(#4255),#2719,.F.);
#31231=ADVANCED_FACE('',(#4256),#2720,.F.);
#31232=ADVANCED_FACE('',(#4257),#2721,.F.);
#31233=ADVANCED_FACE('',(#4258),#2722,.F.);
#31234=ADVANCED_FACE('',(#4259),#2723,.F.);
#31235=ADVANCED_FACE('',(#4260),#2724,.F.);
#31236=ADVANCED_FACE('',(#4261),#2725,.F.);
#31237=ADVANCED_FACE('',(#4262),#2726,.F.);
#31238=ADVANCED_FACE('',(#4263),#2727,.F.);
#31239=ADVANCED_FACE('',(#4264),#2728,.F.);
#31240=ADVANCED_FACE('',(#4265),#2729,.F.);
#31241=ADVANCED_FACE('',(#4266),#2730,.F.);
#31242=ADVANCED_FACE('',(#4267),#2731,.F.);
#31243=ADVANCED_FACE('',(#4268),#2732,.F.);
#31244=ADVANCED_FACE('',(#4269),#2733,.F.);
#31245=ADVANCED_FACE('',(#4270),#2734,.F.);
#31246=ADVANCED_FACE('',(#4271),#2735,.F.);
#31247=ADVANCED_FACE('',(#4272),#2736,.F.);
#31248=ADVANCED_FACE('',(#4273),#2737,.F.);
#31249=ADVANCED_FACE('',(#4274),#2738,.F.);
#31250=ADVANCED_FACE('',(#4275),#2739,.F.);
#31251=ADVANCED_FACE('',(#4276),#2740,.F.);
#31252=ADVANCED_FACE('',(#4277),#2741,.F.);
#31253=ADVANCED_FACE('',(#4278),#2742,.F.);
#31254=ADVANCED_FACE('',(#4279),#2743,.F.);
#31255=ADVANCED_FACE('',(#4280),#2744,.F.);
#31256=ADVANCED_FACE('',(#4281),#2745,.F.);
#31257=ADVANCED_FACE('',(#4282),#2746,.F.);
#31258=ADVANCED_FACE('',(#4283),#2747,.F.);
#31259=ADVANCED_FACE('',(#4284),#2748,.F.);
#31260=ADVANCED_FACE('',(#4285),#2749,.F.);
#31261=ADVANCED_FACE('',(#4286),#2750,.F.);
#31262=ADVANCED_FACE('',(#4287),#2751,.F.);
#31263=ADVANCED_FACE('',(#4288),#2752,.F.);
#31264=ADVANCED_FACE('',(#4289),#2753,.F.);
#31265=ADVANCED_FACE('',(#4290),#2754,.F.);
#31266=ADVANCED_FACE('',(#4291),#2755,.F.);
#31267=ADVANCED_FACE('',(#4292),#2756,.F.);
#31268=ADVANCED_FACE('',(#4293),#2757,.F.);
#31269=ADVANCED_FACE('',(#4294),#2758,.F.);
#31270=ADVANCED_FACE('',(#4295),#2759,.F.);
#31271=ADVANCED_FACE('',(#4296),#2760,.F.);
#31272=ADVANCED_FACE('',(#4297),#2761,.F.);
#31273=ADVANCED_FACE('',(#4298),#2762,.F.);
#31274=ADVANCED_FACE('',(#4299),#2763,.F.);
#31275=ADVANCED_FACE('',(#4300),#2764,.F.);
#31276=ADVANCED_FACE('',(#4301),#2765,.F.);
#31277=ADVANCED_FACE('',(#4302),#2766,.F.);
#31278=ADVANCED_FACE('',(#4303),#2767,.F.);
#31279=ADVANCED_FACE('',(#4304),#2768,.F.);
#31280=ADVANCED_FACE('',(#4305),#2769,.F.);
#31281=ADVANCED_FACE('',(#4306),#2770,.F.);
#31282=ADVANCED_FACE('',(#4307),#2771,.F.);
#31283=ADVANCED_FACE('',(#4308),#2772,.F.);
#31284=ADVANCED_FACE('',(#4309),#2773,.F.);
#31285=ADVANCED_FACE('',(#4310),#2774,.F.);
#31286=ADVANCED_FACE('',(#4311),#2775,.F.);
#31287=ADVANCED_FACE('',(#4312),#2776,.F.);
#31288=ADVANCED_FACE('',(#4313),#2777,.F.);
#31289=ADVANCED_FACE('',(#4314),#2778,.F.);
#31290=ADVANCED_FACE('',(#4315),#2779,.F.);
#31291=ADVANCED_FACE('',(#4316),#2780,.F.);
#31292=ADVANCED_FACE('',(#4317),#2781,.F.);
#31293=ADVANCED_FACE('',(#4318),#2782,.F.);
#31294=ADVANCED_FACE('',(#4319),#2783,.F.);
#31295=ADVANCED_FACE('',(#4320),#2784,.F.);
#31296=ADVANCED_FACE('',(#4321),#2785,.F.);
#31297=ADVANCED_FACE('',(#4322),#2786,.F.);
#31298=ADVANCED_FACE('',(#4323),#2787,.F.);
#31299=ADVANCED_FACE('',(#4324),#2788,.F.);
#31300=ADVANCED_FACE('',(#4325),#2789,.F.);
#31301=ADVANCED_FACE('',(#4326),#2790,.F.);
#31302=ADVANCED_FACE('',(#4327),#2791,.F.);
#31303=ADVANCED_FACE('',(#4328),#2792,.F.);
#31304=ADVANCED_FACE('',(#4329),#2793,.F.);
#31305=ADVANCED_FACE('',(#4330),#2794,.F.);
#31306=ADVANCED_FACE('',(#4331),#2795,.F.);
#31307=ADVANCED_FACE('',(#4332),#2796,.F.);
#31308=ADVANCED_FACE('',(#4333),#2797,.F.);
#31309=ADVANCED_FACE('',(#4334),#2798,.F.);
#31310=ADVANCED_FACE('',(#4335),#2799,.F.);
#31311=ADVANCED_FACE('',(#4336),#2800,.F.);
#31312=ADVANCED_FACE('',(#4337),#2801,.F.);
#31313=ADVANCED_FACE('',(#4338),#2802,.F.);
#31314=ADVANCED_FACE('',(#4339),#2803,.F.);
#31315=ADVANCED_FACE('',(#4340),#2804,.F.);
#31316=ADVANCED_FACE('',(#4341),#2805,.F.);
#31317=ADVANCED_FACE('',(#4342),#2806,.F.);
#31318=ADVANCED_FACE('',(#4343),#2807,.F.);
#31319=ADVANCED_FACE('',(#4344),#2808,.F.);
#31320=ADVANCED_FACE('',(#4345),#2809,.F.);
#31321=ADVANCED_FACE('',(#4346),#2810,.F.);
#31322=ADVANCED_FACE('',(#4347),#2811,.F.);
#31323=ADVANCED_FACE('',(#4348),#2812,.F.);
#31324=ADVANCED_FACE('',(#4349),#2813,.F.);
#31325=ADVANCED_FACE('',(#4350),#2814,.F.);
#31326=ADVANCED_FACE('',(#4351),#2815,.F.);
#31327=ADVANCED_FACE('',(#4352),#2816,.F.);
#31328=ADVANCED_FACE('',(#4353),#2817,.F.);
#31329=ADVANCED_FACE('',(#4354),#2818,.F.);
#31330=ADVANCED_FACE('',(#4355),#2819,.F.);
#31331=ADVANCED_FACE('',(#4356),#2820,.F.);
#31332=ADVANCED_FACE('',(#4357),#2821,.F.);
#31333=ADVANCED_FACE('',(#4358),#2822,.F.);
#31334=ADVANCED_FACE('',(#4359),#2823,.F.);
#31335=ADVANCED_FACE('',(#4360),#2824,.F.);
#31336=ADVANCED_FACE('',(#4361),#2825,.F.);
#31337=ADVANCED_FACE('',(#4362),#2826,.F.);
#31338=ADVANCED_FACE('',(#4363),#2827,.F.);
#31339=ADVANCED_FACE('',(#4364),#2828,.F.);
#31340=ADVANCED_FACE('',(#4365),#2829,.F.);
#31341=ADVANCED_FACE('',(#4366),#2830,.F.);
#31342=ADVANCED_FACE('',(#4367),#2831,.F.);
#31343=ADVANCED_FACE('',(#4368),#2832,.F.);
#31344=ADVANCED_FACE('',(#4369),#2833,.F.);
#31345=ADVANCED_FACE('',(#4370),#2834,.F.);
#31346=ADVANCED_FACE('',(#4371),#2835,.F.);
#31347=ADVANCED_FACE('',(#4372),#2836,.F.);
#31348=ADVANCED_FACE('',(#4373),#2837,.F.);
#31349=ADVANCED_FACE('',(#4374),#2838,.F.);
#31350=ADVANCED_FACE('',(#4375),#2839,.F.);
#31351=ADVANCED_FACE('',(#4376),#2840,.F.);
#31352=ADVANCED_FACE('',(#4377),#2841,.F.);
#31353=ADVANCED_FACE('',(#4378),#2842,.F.);
#31354=ADVANCED_FACE('',(#4379),#2843,.F.);
#31355=ADVANCED_FACE('',(#4380),#2844,.F.);
#31356=ADVANCED_FACE('',(#4381),#2845,.F.);
#31357=ADVANCED_FACE('',(#4382),#2846,.F.);
#31358=ADVANCED_FACE('',(#4383),#2847,.F.);
#31359=ADVANCED_FACE('',(#4384),#2848,.F.);
#31360=ADVANCED_FACE('',(#4385),#2849,.F.);
#31361=ADVANCED_FACE('',(#4386),#2850,.F.);
#31362=ADVANCED_FACE('',(#4387),#2851,.F.);
#31363=ADVANCED_FACE('',(#4388),#2852,.F.);
#31364=ADVANCED_FACE('',(#4389),#2853,.F.);
#31365=ADVANCED_FACE('',(#4390),#2854,.F.);
#31366=ADVANCED_FACE('',(#4391),#2855,.F.);
#31367=ADVANCED_FACE('',(#4392),#2856,.F.);
#31368=ADVANCED_FACE('',(#4393),#2857,.F.);
#31369=ADVANCED_FACE('',(#4394),#2858,.F.);
#31370=ADVANCED_FACE('',(#4395),#2859,.F.);
#31371=ADVANCED_FACE('',(#4396),#2860,.F.);
#31372=ADVANCED_FACE('',(#4397),#2861,.F.);
#31373=ADVANCED_FACE('',(#4398),#2862,.F.);
#31374=ADVANCED_FACE('',(#4399),#2863,.F.);
#31375=ADVANCED_FACE('',(#4400),#2864,.F.);
#31376=ADVANCED_FACE('',(#4401),#2865,.F.);
#31377=ADVANCED_FACE('',(#4402),#2866,.F.);
#31378=ADVANCED_FACE('',(#4403),#2867,.F.);
#31379=ADVANCED_FACE('',(#4404),#2868,.F.);
#31380=ADVANCED_FACE('',(#4405),#2869,.F.);
#31381=ADVANCED_FACE('',(#4406),#2870,.F.);
#31382=ADVANCED_FACE('',(#4407),#2871,.F.);
#31383=ADVANCED_FACE('',(#4408),#2872,.F.);
#31384=ADVANCED_FACE('',(#4409),#2873,.F.);
#31385=ADVANCED_FACE('',(#4410),#2874,.F.);
#31386=ADVANCED_FACE('',(#4411),#2875,.F.);
#31387=ADVANCED_FACE('',(#4412),#2876,.F.);
#31388=ADVANCED_FACE('',(#4413),#2877,.F.);
#31389=ADVANCED_FACE('',(#4414),#2878,.F.);
#31390=ADVANCED_FACE('',(#4415),#2879,.F.);
#31391=ADVANCED_FACE('',(#4416),#2880,.F.);
#31392=ADVANCED_FACE('',(#4417),#2881,.F.);
#31393=ADVANCED_FACE('',(#4418),#2882,.F.);
#31394=ADVANCED_FACE('',(#4419),#2883,.F.);
#31395=ADVANCED_FACE('',(#4420),#2884,.F.);
#31396=ADVANCED_FACE('',(#4421),#2885,.F.);
#31397=ADVANCED_FACE('',(#4422),#2886,.F.);
#31398=ADVANCED_FACE('',(#4423),#2887,.F.);
#31399=ADVANCED_FACE('',(#4424),#2888,.F.);
#31400=ADVANCED_FACE('',(#4425),#2889,.F.);
#31401=ADVANCED_FACE('',(#4426),#2890,.F.);
#31402=ADVANCED_FACE('',(#4427),#2891,.F.);
#31403=ADVANCED_FACE('',(#4428),#2892,.F.);
#31404=ADVANCED_FACE('',(#4429),#2893,.F.);
#31405=ADVANCED_FACE('',(#4430),#2894,.F.);
#31406=ADVANCED_FACE('',(#4431),#2895,.F.);
#31407=ADVANCED_FACE('',(#4432),#2896,.F.);
#31408=ADVANCED_FACE('',(#4433),#2897,.F.);
#31409=ADVANCED_FACE('',(#4434),#2898,.F.);
#31410=ADVANCED_FACE('',(#4435),#2899,.F.);
#31411=ADVANCED_FACE('',(#4436),#2900,.F.);
#31412=ADVANCED_FACE('',(#4437),#2901,.F.);
#31413=ADVANCED_FACE('',(#4438),#2902,.F.);
#31414=ADVANCED_FACE('',(#4439),#2903,.F.);
#31415=ADVANCED_FACE('',(#4440),#2904,.F.);
#31416=ADVANCED_FACE('',(#4441),#2905,.F.);
#31417=ADVANCED_FACE('',(#4442),#2906,.F.);
#31418=ADVANCED_FACE('',(#4443),#2907,.F.);
#31419=ADVANCED_FACE('',(#4444),#2908,.F.);
#31420=ADVANCED_FACE('',(#4445),#2909,.F.);
#31421=ADVANCED_FACE('',(#4446),#2910,.F.);
#31422=ADVANCED_FACE('',(#4447),#2911,.F.);
#31423=ADVANCED_FACE('',(#4448),#2912,.F.);
#31424=ADVANCED_FACE('',(#4449),#2913,.F.);
#31425=ADVANCED_FACE('',(#4450),#2914,.F.);
#31426=ADVANCED_FACE('',(#4451),#2915,.F.);
#31427=ADVANCED_FACE('',(#4452),#2916,.F.);
#31428=ADVANCED_FACE('',(#4453),#2917,.F.);
#31429=ADVANCED_FACE('',(#4454),#2918,.F.);
#31430=ADVANCED_FACE('',(#4455),#2919,.F.);
#31431=ADVANCED_FACE('',(#4456),#2920,.F.);
#31432=ADVANCED_FACE('',(#4457),#2921,.F.);
#31433=ADVANCED_FACE('',(#4458),#2922,.F.);
#31434=ADVANCED_FACE('',(#4459),#2923,.F.);
#31435=ADVANCED_FACE('',(#4460),#2924,.F.);
#31436=ADVANCED_FACE('',(#4461),#2925,.F.);
#31437=ADVANCED_FACE('',(#4462),#2926,.F.);
#31438=ADVANCED_FACE('',(#4463),#2927,.F.);
#31439=ADVANCED_FACE('',(#4464),#2928,.F.);
#31440=ADVANCED_FACE('',(#4465),#2929,.F.);
#31441=ADVANCED_FACE('',(#4466),#2930,.F.);
#31442=ADVANCED_FACE('',(#4467),#2931,.F.);
#31443=ADVANCED_FACE('',(#4468),#2932,.F.);
#31444=ADVANCED_FACE('',(#4469),#2933,.F.);
#31445=ADVANCED_FACE('',(#4470),#2934,.F.);
#31446=ADVANCED_FACE('',(#4471),#2935,.F.);
#31447=ADVANCED_FACE('',(#4472),#2936,.F.);
#31448=ADVANCED_FACE('',(#4473),#2937,.F.);
#31449=ADVANCED_FACE('',(#4474),#2938,.F.);
#31450=ADVANCED_FACE('',(#4475),#2939,.F.);
#31451=ADVANCED_FACE('',(#4476),#2940,.F.);
#31452=ADVANCED_FACE('',(#4477),#2941,.F.);
#31453=ADVANCED_FACE('',(#4478),#2942,.F.);
#31454=ADVANCED_FACE('',(#4479),#2943,.F.);
#31455=ADVANCED_FACE('',(#4480),#2944,.F.);
#31456=ADVANCED_FACE('',(#4481),#2945,.F.);
#31457=ADVANCED_FACE('',(#4482),#2946,.F.);
#31458=ADVANCED_FACE('',(#4483),#2947,.F.);
#31459=ADVANCED_FACE('',(#4484),#2948,.F.);
#31460=ADVANCED_FACE('',(#4485),#2949,.F.);
#31461=ADVANCED_FACE('',(#4486),#2950,.F.);
#31462=ADVANCED_FACE('',(#4487),#2951,.F.);
#31463=ADVANCED_FACE('',(#4488),#2952,.F.);
#31464=ADVANCED_FACE('',(#4489),#2953,.F.);
#31465=ADVANCED_FACE('',(#4490),#2954,.F.);
#31466=ADVANCED_FACE('',(#4491),#1840,.F.);
#31467=ADVANCED_FACE('',(#4492),#1841,.F.);
#31468=ADVANCED_FACE('',(#4493),#2955,.T.);
#31469=ADVANCED_FACE('',(#4494),#1842,.T.);
#31470=ADVANCED_FACE('',(#4495),#2956,.T.);
#31471=ADVANCED_FACE('',(#4496),#1843,.T.);
#31472=ADVANCED_FACE('',(#4497),#2957,.T.);
#31473=ADVANCED_FACE('',(#4498),#1844,.T.);
#31474=ADVANCED_FACE('',(#4499),#2958,.T.);
#31475=ADVANCED_FACE('',(#4500),#1845,.T.);
#31476=ADVANCED_FACE('',(#4501,#2089,#2090,#2091,#2092,#2093,#2094,#2095,
#2096,#2097,#2098,#2099,#2100,#2101,#2102,#2103,#2104,#2105,#2106,#2107,
#2108,#2109,#2110,#2111,#2112,#2113,#2114,#2115,#2116,#2117,#2118,#2119,
#2120,#2121,#2122,#2123,#2124,#2125,#2126,#2127,#2128,#2129,#2130,#2131,
#2132,#2133,#2134,#2135,#2136,#2137,#2138,#2139,#2140,#2141,#2142,#2143,
#2144,#2145,#2146,#2147,#2148,#2149,#2150,#2151,#2152,#2153,#2154,#2155,
#2156,#2157,#2158,#2159,#2160,#2161,#2162,#2163,#2164,#2165,#2166,#2167,
#2168,#2169,#2170,#2171,#2172,#2173,#2174,#2175,#2176,#2177,#2178,#2179,
#2180,#2181,#2182,#2183,#2184,#2185,#2186,#2187,#2188,#2189,#2190,#2191,
#2192),#2959,.T.);
#31477=ADVANCED_FACE('',(#4502,#2193,#2194),#2960,.F.);
#32080=CLOSED_SHELL('',(#30683,#30684,#30685,#30686,#30687,#30688,#30689,
#30690,#30691,#30692,#30693,#30694,#30695,#30696,#30697,#30698,#30699,#30700,
#30701,#30702,#30703,#30704,#30705,#30706,#30707,#30708,#30709,#30710,#30711,
#30712,#30713,#30714,#30715,#30716,#30717,#30718,#30719,#30720,#30721,#30722,
#30723,#30724,#30725,#30726,#30727,#30728,#30729,#30730,#30731,#30732,#30733,
#30734,#30735,#30736,#30737,#30738,#30739,#30740,#30741,#30742,#30743,#30744,
#30745,#30746,#30747,#30748,#30749,#30750,#30751,#30752,#30753,#30754,#30755,
#30756,#30757,#30758,#30759,#30760,#30761,#30762,#30763,#30764,#30765,#30766,
#30767,#30768,#30769,#30770,#30771,#30772,#30773,#30774,#30775,#30776,#30777,
#30778,#30779,#30780,#30781,#30782,#30783,#30784,#30785,#30786,#30787,#30788,
#30789,#30790,#30791,#30792,#30793,#30794,#30795,#30796,#30797,#30798,#30799,
#30800,#30801,#30802,#30803,#30804,#30805,#30806,#30807,#30808,#30809,#30810,
#30811,#30812,#30813,#30814,#30815,#30816,#30817,#30818,#30819,#30820,#30821,
#30822,#30823,#30824,#30825,#30826,#30827,#30828,#30829,#30830,#30831,#30832,
#30833,#30834,#30835,#30836,#30837,#30838,#30839,#30840,#30841,#30842,#30843,
#30844,#30845,#30846,#30847,#30848,#30849,#30850,#30851,#30852,#30853,#30854,
#30855,#30856,#30857,#30858,#30859,#30860,#30861,#30862,#30863,#30864,#30865,
#30866,#30867,#30868,#30869,#30870,#30871,#30872,#30873,#30874,#30875,#30876,
#30877,#30878,#30879,#30880,#30881,#30882,#30883,#30884,#30885,#30886,#30887,
#30888,#30889,#30890,#30891,#30892,#30893,#30894,#30895,#30896,#30897,#30898,
#30899,#30900,#30901,#30902,#30903,#30904,#30905,#30906,#30907,#30908,#30909,
#30910,#30911,#30912,#30913,#30914,#30915,#30916,#30917,#30918,#30919,#30920,
#30921,#30922,#30923,#30924,#30925,#30926,#30927,#30928,#30929,#30930,#30931,
#30932,#30933,#30934,#30935,#30936,#30937,#30938,#30939,#30940,#30941,#30942,
#30943,#30944,#30945,#30946,#30947,#30948,#30949,#30950,#30951,#30952,#30953,
#30954,#30955,#30956,#30957,#30958,#30959,#30960,#30961,#30962,#30963,#30964,
#30965,#30966,#30967,#30968,#30969,#30970,#30971,#30972,#30973,#30974,#30975,
#30976,#30977,#30978,#30979,#30980,#30981,#30982,#30983,#30984,#30985,#30986,
#30987,#30988,#30989,#30990,#30991,#30992,#30993,#30994,#30995,#30996,#30997,
#30998,#30999,#31000,#31001,#31002,#31003,#31004,#31005,#31006,#31007,#31008,
#31009,#31010,#31011,#31012,#31013,#31014,#31015,#31016,#31017,#31018,#31019,
#31020,#31021,#31022,#31023,#31024,#31025,#31026,#31027,#31028,#31029,#31030,
#31031,#31032,#31033,#31034,#31035,#31036,#31037,#31038,#31039,#31040,#31041,
#31042,#31043,#31044,#31045,#31046,#31047,#31048,#31049,#31050,#31051,#31052,
#31053,#31054,#31055,#31056,#31057,#31058,#31059,#31060,#31061,#31062,#31063,
#31064,#31065,#31066,#31067,#31068,#31069,#31070,#31071,#31072,#31073,#31074,
#31075,#31076,#31077,#31078,#31079,#31080,#31081,#31082,#31083,#31084,#31085,
#31086,#31087,#31088,#31089,#31090,#31091,#31092,#31093,#31094,#31095,#31096,
#31097,#31098,#31099,#31100,#31101,#31102,#31103,#31104,#31105,#31106,#31107,
#31108,#31109,#31110,#31111,#31112,#31113,#31114,#31115,#31116,#31117,#31118,
#31119,#31120,#31121,#31122,#31123,#31124,#31125,#31126,#31127,#31128,#31129,
#31130,#31131,#31132,#31133,#31134,#31135,#31136,#31137,#31138,#31139,#31140,
#31141,#31142,#31143,#31144,#31145,#31146,#31147,#31148,#31149,#31150,#31151,
#31152,#31153,#31154,#31155,#31156,#31157,#31158,#31159,#31160,#31161,#31162,
#31163,#31164,#31165,#31166,#31167,#31168,#31169,#31170,#31171,#31172,#31173,
#31174,#31175,#31176,#31177,#31178,#31179,#31180,#31181,#31182,#31183,#31184,
#31185,#31186,#31187,#31188,#31189,#31190,#31191,#31192,#31193,#31194,#31195,
#31196,#31197,#31198,#31199,#31200,#31201,#31202,#31203,#31204,#31205,#31206,
#31207,#31208,#31209,#31210,#31211,#31212,#31213,#31214,#31215,#31216,#31217,
#31218,#31219,#31220,#31221,#31222,#31223,#31224,#31225,#31226,#31227,#31228,
#31229,#31230,#31231,#31232,#31233,#31234,#31235,#31236,#31237,#31238,#31239,
#31240,#31241,#31242,#31243,#31244,#31245,#31246,#31247,#31248,#31249,#31250,
#31251,#31252,#31253,#31254,#31255,#31256,#31257,#31258,#31259,#31260,#31261,
#31262,#31263,#31264,#31265,#31266,#31267,#31268,#31269,#31270,#31271,#31272,
#31273,#31274,#31275,#31276,#31277,#31278,#31279,#31280,#31281,#31282,#31283,
#31284,#31285,#31286,#31287,#31288,#31289,#31290,#31291,#31292,#31293,#31294,
#31295,#31296,#31297,#31298,#31299,#31300,#31301,#31302,#31303,#31304,#31305,
#31306,#31307,#31308,#31309,#31310,#31311,#31312,#31313,#31314,#31315,#31316,
#31317,#31318,#31319,#31320,#31321,#31322,#31323,#31324,#31325,#31326,#31327,
#31328,#31329,#31330,#31331,#31332,#31333,#31334,#31335,#31336,#31337,#31338,
#31339,#31340,#31341,#31342,#31343,#31344,#31345,#31346,#31347,#31348,#31349,
#31350,#31351,#31352,#31353,#31354,#31355,#31356,#31357,#31358,#31359,#31360,
#31361,#31362,#31363,#31364,#31365,#31366,#31367,#31368,#31369,#31370,#31371,
#31372,#31373,#31374,#31375,#31376,#31377,#31378,#31379,#31380,#31381,#31382,
#31383,#31384,#31385,#31386,#31387,#31388,#31389,#31390,#31391,#31392,#31393,
#31394,#31395,#31396,#31397,#31398,#31399,#31400,#31401,#31402,#31403,#31404,
#31405,#31406,#31407,#31408,#31409,#31410,#31411,#31412,#31413,#31414,#31415,
#31416,#31417,#31418,#31419,#31420,#31421,#31422,#31423,#31424,#31425,#31426,
#31427,#31428,#31429,#31430,#31431,#31432,#31433,#31434,#31435,#31436,#31437,
#31438,#31439,#31440,#31441,#31442,#31443,#31444,#31445,#31446,#31447,#31448,
#31449,#31450,#31451,#31452,#31453,#31454,#31455,#31456,#31457,#31458,#31459,
#31460,#31461,#31462,#31463,#31464,#31465,#31466,#31467,#31468,#31469,#31470,
#31471,#31472,#31473,#31474,#31475,#31476,#31477));
#32757=AXIS2_PLACEMENT_3D('',#69950,#35790,#35791);
#32758=AXIS2_PLACEMENT_3D('',#70251,#35812,#35813);
#32759=AXIS2_PLACEMENT_3D('',#70252,#35814,#35815);
#32760=AXIS2_PLACEMENT_3D('',#70261,#35820,#35821);
#32761=AXIS2_PLACEMENT_3D('',#70267,#35825,#35826);
#32762=AXIS2_PLACEMENT_3D('',#70270,#35829,#35830);
#32763=AXIS2_PLACEMENT_3D('',#70279,#35835,#35836);
#32764=AXIS2_PLACEMENT_3D('',#70285,#35840,#35841);
#32765=AXIS2_PLACEMENT_3D('',#70291,#35845,#35846);
#32766=AXIS2_PLACEMENT_3D('',#70297,#35850,#35851);
#32767=AXIS2_PLACEMENT_3D('',#70303,#35855,#35856);
#32768=AXIS2_PLACEMENT_3D('',#70309,#35860,#35861);
#32769=AXIS2_PLACEMENT_3D('',#70315,#35865,#35866);
#32770=AXIS2_PLACEMENT_3D('',#70321,#35870,#35871);
#32771=AXIS2_PLACEMENT_3D('',#70327,#35875,#35876);
#32772=AXIS2_PLACEMENT_3D('',#70333,#35880,#35881);
#32773=AXIS2_PLACEMENT_3D('',#70336,#35884,#35885);
#32774=AXIS2_PLACEMENT_3D('',#70337,#35886,#35887);
#32775=AXIS2_PLACEMENT_3D('',#70338,#35888,#35889);
#32776=AXIS2_PLACEMENT_3D('',#70639,#35910,#35911);
#32777=AXIS2_PLACEMENT_3D('',#70823,#35925,#35926);
#32778=AXIS2_PLACEMENT_3D('',#70934,#35937,#35938);
#32779=AXIS2_PLACEMENT_3D('',#71045,#35949,#35950);
#32780=AXIS2_PLACEMENT_3D('',#71063,#35954,#35955);
#32781=AXIS2_PLACEMENT_3D('',#71064,#35956,#35957);
#32782=AXIS2_PLACEMENT_3D('',#71365,#35978,#35979);
#32783=AXIS2_PLACEMENT_3D('',#71504,#35990,#35991);
#32784=AXIS2_PLACEMENT_3D('',#71645,#36004,#36005);
#32785=AXIS2_PLACEMENT_3D('',#71651,#36009,#36010);
#32786=AXIS2_PLACEMENT_3D('',#71657,#36014,#36015);
#32787=AXIS2_PLACEMENT_3D('',#71660,#36018,#36019);
#32788=AXIS2_PLACEMENT_3D('',#71661,#36020,#36021);
#32789=AXIS2_PLACEMENT_3D('',#71962,#36042,#36043);
#32790=AXIS2_PLACEMENT_3D('',#71963,#36044,#36045);
#32791=AXIS2_PLACEMENT_3D('',#72002,#36052,#36053);
#32792=AXIS2_PLACEMENT_3D('',#72038,#36059,#36060);
#32793=AXIS2_PLACEMENT_3D('',#72044,#36064,#36065);
#32794=AXIS2_PLACEMENT_3D('',#72050,#36069,#36070);
#32795=AXIS2_PLACEMENT_3D('',#72053,#36073,#36074);
#32796=AXIS2_PLACEMENT_3D('',#72054,#36075,#36076);
#32797=AXIS2_PLACEMENT_3D('',#72355,#36097,#36098);
#32798=AXIS2_PLACEMENT_3D('',#72356,#36099,#36100);
#32799=AXIS2_PLACEMENT_3D('',#72657,#36121,#36122);
#32800=AXIS2_PLACEMENT_3D('',#72658,#36123,#36124);
#32801=AXIS2_PLACEMENT_3D('',#72697,#36131,#36132);
#32802=AXIS2_PLACEMENT_3D('',#72733,#36138,#36139);
#32803=AXIS2_PLACEMENT_3D('',#72739,#36143,#36144);
#32804=AXIS2_PLACEMENT_3D('',#72745,#36148,#36149);
#32805=AXIS2_PLACEMENT_3D('',#72748,#36152,#36153);
#32806=AXIS2_PLACEMENT_3D('',#72749,#36154,#36155);
#32807=AXIS2_PLACEMENT_3D('',#73050,#36176,#36177);
#32808=AXIS2_PLACEMENT_3D('',#73189,#36188,#36189);
#32809=AXIS2_PLACEMENT_3D('',#73330,#36202,#36203);
#32810=AXIS2_PLACEMENT_3D('',#73336,#36207,#36208);
#32811=AXIS2_PLACEMENT_3D('',#73342,#36212,#36213);
#32812=AXIS2_PLACEMENT_3D('',#73345,#36216,#36217);
#32813=AXIS2_PLACEMENT_3D('',#73346,#36218,#36219);
#32814=AXIS2_PLACEMENT_3D('',#73647,#36240,#36241);
#32815=AXIS2_PLACEMENT_3D('',#73831,#36255,#36256);
#32816=AXIS2_PLACEMENT_3D('',#73942,#36267,#36268);
#32817=AXIS2_PLACEMENT_3D('',#74053,#36279,#36280);
#32818=AXIS2_PLACEMENT_3D('',#74071,#36284,#36285);
#32819=AXIS2_PLACEMENT_3D('',#74072,#36286,#36287);
#32820=AXIS2_PLACEMENT_3D('',#74373,#36308,#36309);
#32821=AXIS2_PLACEMENT_3D('',#74374,#36310,#36311);
#32822=AXIS2_PLACEMENT_3D('',#74383,#36316,#36317);
#32823=AXIS2_PLACEMENT_3D('',#74389,#36321,#36322);
#32824=AXIS2_PLACEMENT_3D('',#74392,#36325,#36326);
#32825=AXIS2_PLACEMENT_3D('',#74401,#36331,#36332);
#32826=AXIS2_PLACEMENT_3D('',#74407,#36336,#36337);
#32827=AXIS2_PLACEMENT_3D('',#74413,#36341,#36342);
#32828=AXIS2_PLACEMENT_3D('',#74419,#36346,#36347);
#32829=AXIS2_PLACEMENT_3D('',#74425,#36351,#36352);
#32830=AXIS2_PLACEMENT_3D('',#74431,#36356,#36357);
#32831=AXIS2_PLACEMENT_3D('',#74437,#36361,#36362);
#32832=AXIS2_PLACEMENT_3D('',#74443,#36366,#36367);
#32833=AXIS2_PLACEMENT_3D('',#74449,#36371,#36372);
#32834=AXIS2_PLACEMENT_3D('',#74455,#36376,#36377);
#32835=AXIS2_PLACEMENT_3D('',#74458,#36380,#36381);
#32836=AXIS2_PLACEMENT_3D('',#74459,#36382,#36383);
#32837=AXIS2_PLACEMENT_3D('',#74460,#36384,#36385);
#32838=AXIS2_PLACEMENT_3D('',#74461,#36386,#36387);
#32839=AXIS2_PLACEMENT_3D('',#74470,#36392,#36393);
#32840=AXIS2_PLACEMENT_3D('',#74476,#36397,#36398);
#32841=AXIS2_PLACEMENT_3D('',#74482,#36402,#36403);
#32842=AXIS2_PLACEMENT_3D('',#74485,#36406,#36407);
#32843=AXIS2_PLACEMENT_3D('',#74486,#36408,#36409);
#32844=AXIS2_PLACEMENT_3D('',#74495,#36414,#36415);
#32845=AXIS2_PLACEMENT_3D('',#74501,#36419,#36420);
#32846=AXIS2_PLACEMENT_3D('',#74507,#36424,#36425);
#32847=AXIS2_PLACEMENT_3D('',#74510,#36428,#36429);
#32848=AXIS2_PLACEMENT_3D('',#74511,#36430,#36431);
#32849=AXIS2_PLACEMENT_3D('',#74520,#36436,#36437);
#32850=AXIS2_PLACEMENT_3D('',#74526,#36441,#36442);
#32851=AXIS2_PLACEMENT_3D('',#74532,#36446,#36447);
#32852=AXIS2_PLACEMENT_3D('',#74535,#36450,#36451);
#32853=AXIS2_PLACEMENT_3D('',#74536,#36452,#36453);
#32854=AXIS2_PLACEMENT_3D('',#74545,#36458,#36459);
#32855=AXIS2_PLACEMENT_3D('',#74551,#36463,#36464);
#32856=AXIS2_PLACEMENT_3D('',#74557,#36468,#36469);
#32857=AXIS2_PLACEMENT_3D('',#74560,#36472,#36473);
#32858=AXIS2_PLACEMENT_3D('',#74561,#36474,#36475);
#32859=AXIS2_PLACEMENT_3D('',#74570,#36480,#36481);
#32860=AXIS2_PLACEMENT_3D('',#74576,#36485,#36486);
#32861=AXIS2_PLACEMENT_3D('',#74582,#36490,#36491);
#32862=AXIS2_PLACEMENT_3D('',#74585,#36494,#36495);
#32863=AXIS2_PLACEMENT_3D('',#74586,#36496,#36497);
#32864=AXIS2_PLACEMENT_3D('',#74595,#36502,#36503);
#32865=AXIS2_PLACEMENT_3D('',#74601,#36507,#36508);
#32866=AXIS2_PLACEMENT_3D('',#74607,#36512,#36513);
#32867=AXIS2_PLACEMENT_3D('',#74610,#36516,#36517);
#32868=AXIS2_PLACEMENT_3D('',#74611,#36518,#36519);
#32869=AXIS2_PLACEMENT_3D('',#74620,#36524,#36525);
#32870=AXIS2_PLACEMENT_3D('',#74626,#36529,#36530);
#32871=AXIS2_PLACEMENT_3D('',#74632,#36534,#36535);
#32872=AXIS2_PLACEMENT_3D('',#74635,#36538,#36539);
#32873=AXIS2_PLACEMENT_3D('',#74636,#36540,#36541);
#32874=AXIS2_PLACEMENT_3D('',#74645,#36546,#36547);
#32875=AXIS2_PLACEMENT_3D('',#74651,#36551,#36552);
#32876=AXIS2_PLACEMENT_3D('',#74657,#36556,#36557);
#32877=AXIS2_PLACEMENT_3D('',#74660,#36560,#36561);
#32878=AXIS2_PLACEMENT_3D('',#74661,#36562,#36563);
#32879=AXIS2_PLACEMENT_3D('',#74670,#36568,#36569);
#32880=AXIS2_PLACEMENT_3D('',#74676,#36573,#36574);
#32881=AXIS2_PLACEMENT_3D('',#74682,#36578,#36579);
#32882=AXIS2_PLACEMENT_3D('',#74685,#36582,#36583);
#32883=AXIS2_PLACEMENT_3D('',#74686,#36584,#36585);
#32884=AXIS2_PLACEMENT_3D('',#74695,#36590,#36591);
#32885=AXIS2_PLACEMENT_3D('',#74701,#36595,#36596);
#32886=AXIS2_PLACEMENT_3D('',#74707,#36600,#36601);
#32887=AXIS2_PLACEMENT_3D('',#74710,#36604,#36605);
#32888=AXIS2_PLACEMENT_3D('',#74711,#36606,#36607);
#32889=AXIS2_PLACEMENT_3D('',#74720,#36612,#36613);
#32890=AXIS2_PLACEMENT_3D('',#74726,#36617,#36618);
#32891=AXIS2_PLACEMENT_3D('',#74732,#36622,#36623);
#32892=AXIS2_PLACEMENT_3D('',#74735,#36626,#36627);
#32893=AXIS2_PLACEMENT_3D('',#74736,#36628,#36629);
#32894=AXIS2_PLACEMENT_3D('',#74745,#36634,#36635);
#32895=AXIS2_PLACEMENT_3D('',#74751,#36639,#36640);
#32896=AXIS2_PLACEMENT_3D('',#74757,#36644,#36645);
#32897=AXIS2_PLACEMENT_3D('',#74760,#36648,#36649);
#32898=AXIS2_PLACEMENT_3D('',#74761,#36650,#36651);
#32899=AXIS2_PLACEMENT_3D('',#74770,#36656,#36657);
#32900=AXIS2_PLACEMENT_3D('',#74776,#36661,#36662);
#32901=AXIS2_PLACEMENT_3D('',#74782,#36666,#36667);
#32902=AXIS2_PLACEMENT_3D('',#74785,#36670,#36671);
#32903=AXIS2_PLACEMENT_3D('',#74786,#36672,#36673);
#32904=AXIS2_PLACEMENT_3D('',#74795,#36678,#36679);
#32905=AXIS2_PLACEMENT_3D('',#74801,#36683,#36684);
#32906=AXIS2_PLACEMENT_3D('',#74807,#36688,#36689);
#32907=AXIS2_PLACEMENT_3D('',#74810,#36692,#36693);
#32908=AXIS2_PLACEMENT_3D('',#74811,#36694,#36695);
#32909=AXIS2_PLACEMENT_3D('',#74820,#36700,#36701);
#32910=AXIS2_PLACEMENT_3D('',#74826,#36705,#36706);
#32911=AXIS2_PLACEMENT_3D('',#74832,#36710,#36711);
#32912=AXIS2_PLACEMENT_3D('',#74835,#36714,#36715);
#32913=AXIS2_PLACEMENT_3D('',#74836,#36716,#36717);
#32914=AXIS2_PLACEMENT_3D('',#74845,#36722,#36723);
#32915=AXIS2_PLACEMENT_3D('',#74851,#36727,#36728);
#32916=AXIS2_PLACEMENT_3D('',#74857,#36732,#36733);
#32917=AXIS2_PLACEMENT_3D('',#74860,#36736,#36737);
#32918=AXIS2_PLACEMENT_3D('',#74861,#36738,#36739);
#32919=AXIS2_PLACEMENT_3D('',#74870,#36744,#36745);
#32920=AXIS2_PLACEMENT_3D('',#74876,#36749,#36750);
#32921=AXIS2_PLACEMENT_3D('',#74882,#36754,#36755);
#32922=AXIS2_PLACEMENT_3D('',#74885,#36758,#36759);
#32923=AXIS2_PLACEMENT_3D('',#74886,#36760,#36761);
#32924=AXIS2_PLACEMENT_3D('',#74895,#36766,#36767);
#32925=AXIS2_PLACEMENT_3D('',#74901,#36771,#36772);
#32926=AXIS2_PLACEMENT_3D('',#74907,#36776,#36777);
#32927=AXIS2_PLACEMENT_3D('',#74910,#36780,#36781);
#32928=AXIS2_PLACEMENT_3D('',#74911,#36782,#36783);
#32929=AXIS2_PLACEMENT_3D('',#74920,#36788,#36789);
#32930=AXIS2_PLACEMENT_3D('',#74926,#36793,#36794);
#32931=AXIS2_PLACEMENT_3D('',#74932,#36798,#36799);
#32932=AXIS2_PLACEMENT_3D('',#74935,#36802,#36803);
#32933=AXIS2_PLACEMENT_3D('',#74936,#36804,#36805);
#32934=AXIS2_PLACEMENT_3D('',#74945,#36810,#36811);
#32935=AXIS2_PLACEMENT_3D('',#74951,#36815,#36816);
#32936=AXIS2_PLACEMENT_3D('',#74957,#36820,#36821);
#32937=AXIS2_PLACEMENT_3D('',#74960,#36824,#36825);
#32938=AXIS2_PLACEMENT_3D('',#74961,#36826,#36827);
#32939=AXIS2_PLACEMENT_3D('',#74970,#36832,#36833);
#32940=AXIS2_PLACEMENT_3D('',#74976,#36837,#36838);
#32941=AXIS2_PLACEMENT_3D('',#74982,#36842,#36843);
#32942=AXIS2_PLACEMENT_3D('',#74985,#36846,#36847);
#32943=AXIS2_PLACEMENT_3D('',#74986,#36848,#36849);
#32944=AXIS2_PLACEMENT_3D('',#74995,#36854,#36855);
#32945=AXIS2_PLACEMENT_3D('',#75001,#36859,#36860);
#32946=AXIS2_PLACEMENT_3D('',#75007,#36864,#36865);
#32947=AXIS2_PLACEMENT_3D('',#75010,#36868,#36869);
#32948=AXIS2_PLACEMENT_3D('',#75011,#36870,#36871);
#32949=AXIS2_PLACEMENT_3D('',#75020,#36876,#36877);
#32950=AXIS2_PLACEMENT_3D('',#75026,#36881,#36882);
#32951=AXIS2_PLACEMENT_3D('',#75032,#36886,#36887);
#32952=AXIS2_PLACEMENT_3D('',#75035,#36890,#36891);
#32953=AXIS2_PLACEMENT_3D('',#75036,#36892,#36893);
#32954=AXIS2_PLACEMENT_3D('',#75045,#36898,#36899);
#32955=AXIS2_PLACEMENT_3D('',#75051,#36903,#36904);
#32956=AXIS2_PLACEMENT_3D('',#75057,#36908,#36909);
#32957=AXIS2_PLACEMENT_3D('',#75060,#36912,#36913);
#32958=AXIS2_PLACEMENT_3D('',#75061,#36914,#36915);
#32959=AXIS2_PLACEMENT_3D('',#75070,#36920,#36921);
#32960=AXIS2_PLACEMENT_3D('',#75076,#36925,#36926);
#32961=AXIS2_PLACEMENT_3D('',#75082,#36930,#36931);
#32962=AXIS2_PLACEMENT_3D('',#75085,#36934,#36935);
#32963=AXIS2_PLACEMENT_3D('',#75086,#36936,#36937);
#32964=AXIS2_PLACEMENT_3D('',#75095,#36942,#36943);
#32965=AXIS2_PLACEMENT_3D('',#75101,#36947,#36948);
#32966=AXIS2_PLACEMENT_3D('',#75107,#36952,#36953);
#32967=AXIS2_PLACEMENT_3D('',#75110,#36956,#36957);
#32968=AXIS2_PLACEMENT_3D('',#75111,#36958,#36959);
#32969=AXIS2_PLACEMENT_3D('',#75120,#36964,#36965);
#32970=AXIS2_PLACEMENT_3D('',#75126,#36969,#36970);
#32971=AXIS2_PLACEMENT_3D('',#75132,#36974,#36975);
#32972=AXIS2_PLACEMENT_3D('',#75135,#36978,#36979);
#32973=AXIS2_PLACEMENT_3D('',#75136,#36980,#36981);
#32974=AXIS2_PLACEMENT_3D('',#75145,#36986,#36987);
#32975=AXIS2_PLACEMENT_3D('',#75151,#36991,#36992);
#32976=AXIS2_PLACEMENT_3D('',#75157,#36996,#36997);
#32977=AXIS2_PLACEMENT_3D('',#75160,#37000,#37001);
#32978=AXIS2_PLACEMENT_3D('',#75161,#37002,#37003);
#32979=AXIS2_PLACEMENT_3D('',#75170,#37008,#37009);
#32980=AXIS2_PLACEMENT_3D('',#75176,#37013,#37014);
#32981=AXIS2_PLACEMENT_3D('',#75182,#37018,#37019);
#32982=AXIS2_PLACEMENT_3D('',#75185,#37022,#37023);
#32983=AXIS2_PLACEMENT_3D('',#75186,#37024,#37025);
#32984=AXIS2_PLACEMENT_3D('',#75195,#37030,#37031);
#32985=AXIS2_PLACEMENT_3D('',#75201,#37035,#37036);
#32986=AXIS2_PLACEMENT_3D('',#75207,#37040,#37041);
#32987=AXIS2_PLACEMENT_3D('',#75210,#37044,#37045);
#32988=AXIS2_PLACEMENT_3D('',#75211,#37046,#37047);
#32989=AXIS2_PLACEMENT_3D('',#75220,#37052,#37053);
#32990=AXIS2_PLACEMENT_3D('',#75226,#37057,#37058);
#32991=AXIS2_PLACEMENT_3D('',#75232,#37062,#37063);
#32992=AXIS2_PLACEMENT_3D('',#75235,#37066,#37067);
#32993=AXIS2_PLACEMENT_3D('',#75236,#37068,#37069);
#32994=AXIS2_PLACEMENT_3D('',#75245,#37074,#37075);
#32995=AXIS2_PLACEMENT_3D('',#75251,#37079,#37080);
#32996=AXIS2_PLACEMENT_3D('',#75257,#37084,#37085);
#32997=AXIS2_PLACEMENT_3D('',#75260,#37088,#37089);
#32998=AXIS2_PLACEMENT_3D('',#75261,#37090,#37091);
#32999=AXIS2_PLACEMENT_3D('',#75270,#37096,#37097);
#33000=AXIS2_PLACEMENT_3D('',#75276,#37101,#37102);
#33001=AXIS2_PLACEMENT_3D('',#75282,#37106,#37107);
#33002=AXIS2_PLACEMENT_3D('',#75285,#37110,#37111);
#33003=AXIS2_PLACEMENT_3D('',#75286,#37112,#37113);
#33004=AXIS2_PLACEMENT_3D('',#75295,#37118,#37119);
#33005=AXIS2_PLACEMENT_3D('',#75301,#37123,#37124);
#33006=AXIS2_PLACEMENT_3D('',#75307,#37128,#37129);
#33007=AXIS2_PLACEMENT_3D('',#75310,#37132,#37133);
#33008=AXIS2_PLACEMENT_3D('',#75311,#37134,#37135);
#33009=AXIS2_PLACEMENT_3D('',#75320,#37140,#37141);
#33010=AXIS2_PLACEMENT_3D('',#75326,#37145,#37146);
#33011=AXIS2_PLACEMENT_3D('',#75332,#37150,#37151);
#33012=AXIS2_PLACEMENT_3D('',#75335,#37154,#37155);
#33013=AXIS2_PLACEMENT_3D('',#75336,#37156,#37157);
#33014=AXIS2_PLACEMENT_3D('',#75345,#37162,#37163);
#33015=AXIS2_PLACEMENT_3D('',#75351,#37167,#37168);
#33016=AXIS2_PLACEMENT_3D('',#75357,#37172,#37173);
#33017=AXIS2_PLACEMENT_3D('',#75360,#37176,#37177);
#33018=AXIS2_PLACEMENT_3D('',#75361,#37178,#37179);
#33019=AXIS2_PLACEMENT_3D('',#75370,#37184,#37185);
#33020=AXIS2_PLACEMENT_3D('',#75376,#37189,#37190);
#33021=AXIS2_PLACEMENT_3D('',#75382,#37194,#37195);
#33022=AXIS2_PLACEMENT_3D('',#75385,#37198,#37199);
#33023=AXIS2_PLACEMENT_3D('',#75386,#37200,#37201);
#33024=AXIS2_PLACEMENT_3D('',#75395,#37206,#37207);
#33025=AXIS2_PLACEMENT_3D('',#75401,#37211,#37212);
#33026=AXIS2_PLACEMENT_3D('',#75407,#37216,#37217);
#33027=AXIS2_PLACEMENT_3D('',#75410,#37220,#37221);
#33028=AXIS2_PLACEMENT_3D('',#75411,#37222,#37223);
#33029=AXIS2_PLACEMENT_3D('',#75420,#37228,#37229);
#33030=AXIS2_PLACEMENT_3D('',#75426,#37233,#37234);
#33031=AXIS2_PLACEMENT_3D('',#75432,#37238,#37239);
#33032=AXIS2_PLACEMENT_3D('',#75435,#37242,#37243);
#33033=AXIS2_PLACEMENT_3D('',#75436,#37244,#37245);
#33034=AXIS2_PLACEMENT_3D('',#75445,#37250,#37251);
#33035=AXIS2_PLACEMENT_3D('',#75451,#37255,#37256);
#33036=AXIS2_PLACEMENT_3D('',#75457,#37260,#37261);
#33037=AXIS2_PLACEMENT_3D('',#75460,#37264,#37265);
#33038=AXIS2_PLACEMENT_3D('',#75461,#37266,#37267);
#33039=AXIS2_PLACEMENT_3D('',#75470,#37272,#37273);
#33040=AXIS2_PLACEMENT_3D('',#75476,#37277,#37278);
#33041=AXIS2_PLACEMENT_3D('',#75482,#37282,#37283);
#33042=AXIS2_PLACEMENT_3D('',#75485,#37286,#37287);
#33043=AXIS2_PLACEMENT_3D('',#75486,#37288,#37289);
#33044=AXIS2_PLACEMENT_3D('',#75495,#37294,#37295);
#33045=AXIS2_PLACEMENT_3D('',#75501,#37299,#37300);
#33046=AXIS2_PLACEMENT_3D('',#75507,#37304,#37305);
#33047=AXIS2_PLACEMENT_3D('',#75510,#37308,#37309);
#33048=AXIS2_PLACEMENT_3D('',#75511,#37310,#37311);
#33049=AXIS2_PLACEMENT_3D('',#75520,#37316,#37317);
#33050=AXIS2_PLACEMENT_3D('',#75526,#37321,#37322);
#33051=AXIS2_PLACEMENT_3D('',#75532,#37326,#37327);
#33052=AXIS2_PLACEMENT_3D('',#75535,#37330,#37331);
#33053=AXIS2_PLACEMENT_3D('',#75536,#37332,#37333);
#33054=AXIS2_PLACEMENT_3D('',#75545,#37338,#37339);
#33055=AXIS2_PLACEMENT_3D('',#75551,#37343,#37344);
#33056=AXIS2_PLACEMENT_3D('',#75557,#37348,#37349);
#33057=AXIS2_PLACEMENT_3D('',#75560,#37352,#37353);
#33058=AXIS2_PLACEMENT_3D('',#75561,#37354,#37355);
#33059=AXIS2_PLACEMENT_3D('',#75570,#37360,#37361);
#33060=AXIS2_PLACEMENT_3D('',#75576,#37365,#37366);
#33061=AXIS2_PLACEMENT_3D('',#75582,#37370,#37371);
#33062=AXIS2_PLACEMENT_3D('',#75585,#37374,#37375);
#33063=AXIS2_PLACEMENT_3D('',#75586,#37376,#37377);
#33064=AXIS2_PLACEMENT_3D('',#75595,#37382,#37383);
#33065=AXIS2_PLACEMENT_3D('',#75601,#37387,#37388);
#33066=AXIS2_PLACEMENT_3D('',#75607,#37392,#37393);
#33067=AXIS2_PLACEMENT_3D('',#75610,#37396,#37397);
#33068=AXIS2_PLACEMENT_3D('',#75611,#37398,#37399);
#33069=AXIS2_PLACEMENT_3D('',#75620,#37404,#37405);
#33070=AXIS2_PLACEMENT_3D('',#75626,#37409,#37410);
#33071=AXIS2_PLACEMENT_3D('',#75632,#37414,#37415);
#33072=AXIS2_PLACEMENT_3D('',#75635,#37418,#37419);
#33073=AXIS2_PLACEMENT_3D('',#75636,#37420,#37421);
#33074=AXIS2_PLACEMENT_3D('',#75645,#37426,#37427);
#33075=AXIS2_PLACEMENT_3D('',#75651,#37431,#37432);
#33076=AXIS2_PLACEMENT_3D('',#75657,#37436,#37437);
#33077=AXIS2_PLACEMENT_3D('',#75660,#37440,#37441);
#33078=AXIS2_PLACEMENT_3D('',#75661,#37442,#37443);
#33079=AXIS2_PLACEMENT_3D('',#75670,#37448,#37449);
#33080=AXIS2_PLACEMENT_3D('',#75676,#37453,#37454);
#33081=AXIS2_PLACEMENT_3D('',#75682,#37458,#37459);
#33082=AXIS2_PLACEMENT_3D('',#75685,#37462,#37463);
#33083=AXIS2_PLACEMENT_3D('',#75686,#37464,#37465);
#33084=AXIS2_PLACEMENT_3D('',#75695,#37470,#37471);
#33085=AXIS2_PLACEMENT_3D('',#75701,#37475,#37476);
#33086=AXIS2_PLACEMENT_3D('',#75707,#37480,#37481);
#33087=AXIS2_PLACEMENT_3D('',#75710,#37484,#37485);
#33088=AXIS2_PLACEMENT_3D('',#75711,#37486,#37487);
#33089=AXIS2_PLACEMENT_3D('',#75720,#37492,#37493);
#33090=AXIS2_PLACEMENT_3D('',#75726,#37497,#37498);
#33091=AXIS2_PLACEMENT_3D('',#75732,#37502,#37503);
#33092=AXIS2_PLACEMENT_3D('',#75735,#37506,#37507);
#33093=AXIS2_PLACEMENT_3D('',#75736,#37508,#37509);
#33094=AXIS2_PLACEMENT_3D('',#75745,#37514,#37515);
#33095=AXIS2_PLACEMENT_3D('',#75751,#37519,#37520);
#33096=AXIS2_PLACEMENT_3D('',#75757,#37524,#37525);
#33097=AXIS2_PLACEMENT_3D('',#75760,#37528,#37529);
#33098=AXIS2_PLACEMENT_3D('',#75761,#37530,#37531);
#33099=AXIS2_PLACEMENT_3D('',#75770,#37536,#37537);
#33100=AXIS2_PLACEMENT_3D('',#75776,#37541,#37542);
#33101=AXIS2_PLACEMENT_3D('',#75782,#37546,#37547);
#33102=AXIS2_PLACEMENT_3D('',#75785,#37550,#37551);
#33103=AXIS2_PLACEMENT_3D('',#75786,#37552,#37553);
#33104=AXIS2_PLACEMENT_3D('',#75795,#37558,#37559);
#33105=AXIS2_PLACEMENT_3D('',#75801,#37563,#37564);
#33106=AXIS2_PLACEMENT_3D('',#75807,#37568,#37569);
#33107=AXIS2_PLACEMENT_3D('',#75810,#37572,#37573);
#33108=AXIS2_PLACEMENT_3D('',#75811,#37574,#37575);
#33109=AXIS2_PLACEMENT_3D('',#75820,#37580,#37581);
#33110=AXIS2_PLACEMENT_3D('',#75826,#37585,#37586);
#33111=AXIS2_PLACEMENT_3D('',#75832,#37590,#37591);
#33112=AXIS2_PLACEMENT_3D('',#75835,#37594,#37595);
#33113=AXIS2_PLACEMENT_3D('',#75836,#37596,#37597);
#33114=AXIS2_PLACEMENT_3D('',#75845,#37602,#37603);
#33115=AXIS2_PLACEMENT_3D('',#75851,#37607,#37608);
#33116=AXIS2_PLACEMENT_3D('',#75857,#37612,#37613);
#33117=AXIS2_PLACEMENT_3D('',#75860,#37616,#37617);
#33118=AXIS2_PLACEMENT_3D('',#75861,#37618,#37619);
#33119=AXIS2_PLACEMENT_3D('',#75870,#37624,#37625);
#33120=AXIS2_PLACEMENT_3D('',#75876,#37629,#37630);
#33121=AXIS2_PLACEMENT_3D('',#75882,#37634,#37635);
#33122=AXIS2_PLACEMENT_3D('',#75885,#37638,#37639);
#33123=AXIS2_PLACEMENT_3D('',#75886,#37640,#37641);
#33124=AXIS2_PLACEMENT_3D('',#75895,#37646,#37647);
#33125=AXIS2_PLACEMENT_3D('',#75901,#37651,#37652);
#33126=AXIS2_PLACEMENT_3D('',#75907,#37656,#37657);
#33127=AXIS2_PLACEMENT_3D('',#75910,#37660,#37661);
#33128=AXIS2_PLACEMENT_3D('',#75911,#37662,#37663);
#33129=AXIS2_PLACEMENT_3D('',#75920,#37668,#37669);
#33130=AXIS2_PLACEMENT_3D('',#75926,#37673,#37674);
#33131=AXIS2_PLACEMENT_3D('',#75932,#37678,#37679);
#33132=AXIS2_PLACEMENT_3D('',#75935,#37682,#37683);
#33133=AXIS2_PLACEMENT_3D('',#75936,#37684,#37685);
#33134=AXIS2_PLACEMENT_3D('',#75945,#37690,#37691);
#33135=AXIS2_PLACEMENT_3D('',#75951,#37695,#37696);
#33136=AXIS2_PLACEMENT_3D('',#75957,#37700,#37701);
#33137=AXIS2_PLACEMENT_3D('',#75960,#37704,#37705);
#33138=AXIS2_PLACEMENT_3D('',#75961,#37706,#37707);
#33139=AXIS2_PLACEMENT_3D('',#75970,#37712,#37713);
#33140=AXIS2_PLACEMENT_3D('',#75976,#37717,#37718);
#33141=AXIS2_PLACEMENT_3D('',#75982,#37722,#37723);
#33142=AXIS2_PLACEMENT_3D('',#75985,#37726,#37727);
#33143=AXIS2_PLACEMENT_3D('',#75986,#37728,#37729);
#33144=AXIS2_PLACEMENT_3D('',#75995,#37734,#37735);
#33145=AXIS2_PLACEMENT_3D('',#76001,#37739,#37740);
#33146=AXIS2_PLACEMENT_3D('',#76007,#37744,#37745);
#33147=AXIS2_PLACEMENT_3D('',#76010,#37748,#37749);
#33148=AXIS2_PLACEMENT_3D('',#76011,#37750,#37751);
#33149=AXIS2_PLACEMENT_3D('',#76020,#37756,#37757);
#33150=AXIS2_PLACEMENT_3D('',#76026,#37761,#37762);
#33151=AXIS2_PLACEMENT_3D('',#76032,#37766,#37767);
#33152=AXIS2_PLACEMENT_3D('',#76035,#37770,#37771);
#33153=AXIS2_PLACEMENT_3D('',#76036,#37772,#37773);
#33154=AXIS2_PLACEMENT_3D('',#76045,#37778,#37779);
#33155=AXIS2_PLACEMENT_3D('',#76051,#37783,#37784);
#33156=AXIS2_PLACEMENT_3D('',#76057,#37788,#37789);
#33157=AXIS2_PLACEMENT_3D('',#76060,#37792,#37793);
#33158=AXIS2_PLACEMENT_3D('',#76061,#37794,#37795);
#33159=AXIS2_PLACEMENT_3D('',#76070,#37800,#37801);
#33160=AXIS2_PLACEMENT_3D('',#76076,#37805,#37806);
#33161=AXIS2_PLACEMENT_3D('',#76082,#37810,#37811);
#33162=AXIS2_PLACEMENT_3D('',#76085,#37814,#37815);
#33163=AXIS2_PLACEMENT_3D('',#76086,#37816,#37817);
#33164=AXIS2_PLACEMENT_3D('',#76095,#37822,#37823);
#33165=AXIS2_PLACEMENT_3D('',#76101,#37827,#37828);
#33166=AXIS2_PLACEMENT_3D('',#76107,#37832,#37833);
#33167=AXIS2_PLACEMENT_3D('',#76110,#37836,#37837);
#33168=AXIS2_PLACEMENT_3D('',#76111,#37838,#37839);
#33169=AXIS2_PLACEMENT_3D('',#76120,#37844,#37845);
#33170=AXIS2_PLACEMENT_3D('',#76126,#37849,#37850);
#33171=AXIS2_PLACEMENT_3D('',#76132,#37854,#37855);
#33172=AXIS2_PLACEMENT_3D('',#76135,#37858,#37859);
#33173=AXIS2_PLACEMENT_3D('',#76136,#37860,#37861);
#33174=AXIS2_PLACEMENT_3D('',#76145,#37866,#37867);
#33175=AXIS2_PLACEMENT_3D('',#76151,#37871,#37872);
#33176=AXIS2_PLACEMENT_3D('',#76157,#37876,#37877);
#33177=AXIS2_PLACEMENT_3D('',#76160,#37880,#37881);
#33178=AXIS2_PLACEMENT_3D('',#76161,#37882,#37883);
#33179=AXIS2_PLACEMENT_3D('',#76170,#37888,#37889);
#33180=AXIS2_PLACEMENT_3D('',#76176,#37893,#37894);
#33181=AXIS2_PLACEMENT_3D('',#76182,#37898,#37899);
#33182=AXIS2_PLACEMENT_3D('',#76185,#37902,#37903);
#33183=AXIS2_PLACEMENT_3D('',#76186,#37904,#37905);
#33184=AXIS2_PLACEMENT_3D('',#76195,#37910,#37911);
#33185=AXIS2_PLACEMENT_3D('',#76201,#37915,#37916);
#33186=AXIS2_PLACEMENT_3D('',#76207,#37920,#37921);
#33187=AXIS2_PLACEMENT_3D('',#76210,#37924,#37925);
#33188=AXIS2_PLACEMENT_3D('',#76211,#37926,#37927);
#33189=AXIS2_PLACEMENT_3D('',#76220,#37932,#37933);
#33190=AXIS2_PLACEMENT_3D('',#76226,#37937,#37938);
#33191=AXIS2_PLACEMENT_3D('',#76232,#37942,#37943);
#33192=AXIS2_PLACEMENT_3D('',#76235,#37946,#37947);
#33193=AXIS2_PLACEMENT_3D('',#76236,#37948,#37949);
#33194=AXIS2_PLACEMENT_3D('',#76245,#37954,#37955);
#33195=AXIS2_PLACEMENT_3D('',#76251,#37959,#37960);
#33196=AXIS2_PLACEMENT_3D('',#76257,#37964,#37965);
#33197=AXIS2_PLACEMENT_3D('',#76260,#37968,#37969);
#33198=AXIS2_PLACEMENT_3D('',#76261,#37970,#37971);
#33199=AXIS2_PLACEMENT_3D('',#76270,#37976,#37977);
#33200=AXIS2_PLACEMENT_3D('',#76276,#37981,#37982);
#33201=AXIS2_PLACEMENT_3D('',#76282,#37986,#37987);
#33202=AXIS2_PLACEMENT_3D('',#76285,#37990,#37991);
#33203=AXIS2_PLACEMENT_3D('',#76286,#37992,#37993);
#33204=AXIS2_PLACEMENT_3D('',#76295,#37998,#37999);
#33205=AXIS2_PLACEMENT_3D('',#76301,#38003,#38004);
#33206=AXIS2_PLACEMENT_3D('',#76307,#38008,#38009);
#33207=AXIS2_PLACEMENT_3D('',#76310,#38012,#38013);
#33208=AXIS2_PLACEMENT_3D('',#76311,#38014,#38015);
#33209=AXIS2_PLACEMENT_3D('',#76320,#38020,#38021);
#33210=AXIS2_PLACEMENT_3D('',#76326,#38025,#38026);
#33211=AXIS2_PLACEMENT_3D('',#76332,#38030,#38031);
#33212=AXIS2_PLACEMENT_3D('',#76335,#38034,#38035);
#33213=AXIS2_PLACEMENT_3D('',#76336,#38036,#38037);
#33214=AXIS2_PLACEMENT_3D('',#76345,#38042,#38043);
#33215=AXIS2_PLACEMENT_3D('',#76351,#38047,#38048);
#33216=AXIS2_PLACEMENT_3D('',#76357,#38052,#38053);
#33217=AXIS2_PLACEMENT_3D('',#76360,#38056,#38057);
#33218=AXIS2_PLACEMENT_3D('',#76361,#38058,#38059);
#33219=AXIS2_PLACEMENT_3D('',#76370,#38064,#38065);
#33220=AXIS2_PLACEMENT_3D('',#76376,#38069,#38070);
#33221=AXIS2_PLACEMENT_3D('',#76382,#38074,#38075);
#33222=AXIS2_PLACEMENT_3D('',#76385,#38078,#38079);
#33223=AXIS2_PLACEMENT_3D('',#76386,#38080,#38081);
#33224=AXIS2_PLACEMENT_3D('',#76395,#38086,#38087);
#33225=AXIS2_PLACEMENT_3D('',#76401,#38091,#38092);
#33226=AXIS2_PLACEMENT_3D('',#76407,#38096,#38097);
#33227=AXIS2_PLACEMENT_3D('',#76410,#38100,#38101);
#33228=AXIS2_PLACEMENT_3D('',#76411,#38102,#38103);
#33229=AXIS2_PLACEMENT_3D('',#76420,#38108,#38109);
#33230=AXIS2_PLACEMENT_3D('',#76426,#38113,#38114);
#33231=AXIS2_PLACEMENT_3D('',#76432,#38118,#38119);
#33232=AXIS2_PLACEMENT_3D('',#76435,#38122,#38123);
#33233=AXIS2_PLACEMENT_3D('',#76436,#38124,#38125);
#33234=AXIS2_PLACEMENT_3D('',#76445,#38130,#38131);
#33235=AXIS2_PLACEMENT_3D('',#76451,#38135,#38136);
#33236=AXIS2_PLACEMENT_3D('',#76457,#38140,#38141);
#33237=AXIS2_PLACEMENT_3D('',#76460,#38144,#38145);
#33238=AXIS2_PLACEMENT_3D('',#76461,#38146,#38147);
#33239=AXIS2_PLACEMENT_3D('',#76470,#38152,#38153);
#33240=AXIS2_PLACEMENT_3D('',#76476,#38157,#38158);
#33241=AXIS2_PLACEMENT_3D('',#76482,#38162,#38163);
#33242=AXIS2_PLACEMENT_3D('',#76485,#38166,#38167);
#33243=AXIS2_PLACEMENT_3D('',#76486,#38168,#38169);
#33244=AXIS2_PLACEMENT_3D('',#76495,#38174,#38175);
#33245=AXIS2_PLACEMENT_3D('',#76501,#38179,#38180);
#33246=AXIS2_PLACEMENT_3D('',#76507,#38184,#38185);
#33247=AXIS2_PLACEMENT_3D('',#76510,#38188,#38189);
#33248=AXIS2_PLACEMENT_3D('',#76511,#38190,#38191);
#33249=AXIS2_PLACEMENT_3D('',#76520,#38196,#38197);
#33250=AXIS2_PLACEMENT_3D('',#76526,#38201,#38202);
#33251=AXIS2_PLACEMENT_3D('',#76532,#38206,#38207);
#33252=AXIS2_PLACEMENT_3D('',#76535,#38210,#38211);
#33253=AXIS2_PLACEMENT_3D('',#76536,#38212,#38213);
#33254=AXIS2_PLACEMENT_3D('',#76545,#38218,#38219);
#33255=AXIS2_PLACEMENT_3D('',#76551,#38223,#38224);
#33256=AXIS2_PLACEMENT_3D('',#76557,#38228,#38229);
#33257=AXIS2_PLACEMENT_3D('',#76560,#38232,#38233);
#33258=AXIS2_PLACEMENT_3D('',#76561,#38234,#38235);
#33259=AXIS2_PLACEMENT_3D('',#76570,#38240,#38241);
#33260=AXIS2_PLACEMENT_3D('',#76576,#38245,#38246);
#33261=AXIS2_PLACEMENT_3D('',#76582,#38250,#38251);
#33262=AXIS2_PLACEMENT_3D('',#76585,#38254,#38255);
#33263=AXIS2_PLACEMENT_3D('',#76586,#38256,#38257);
#33264=AXIS2_PLACEMENT_3D('',#76588,#38258,#38259);
#33265=AXIS2_PLACEMENT_3D('',#76591,#38261,#38262);
#33266=AXIS2_PLACEMENT_3D('',#76592,#38263,#38264);
#33267=AXIS2_PLACEMENT_3D('',#76594,#38265,#38266);
#33268=AXIS2_PLACEMENT_3D('',#76597,#38268,#38269);
#33269=AXIS2_PLACEMENT_3D('',#76598,#38270,#38271);
#33270=AXIS2_PLACEMENT_3D('',#76607,#38276,#38277);
#33271=AXIS2_PLACEMENT_3D('',#76609,#38278,#38279);
#33272=AXIS2_PLACEMENT_3D('',#76611,#38280,#38281);
#33273=AXIS2_PLACEMENT_3D('',#76613,#38283,#38284);
#33274=AXIS2_PLACEMENT_3D('',#76619,#38288,#38289);
#33275=AXIS2_PLACEMENT_3D('',#76621,#38290,#38291);
#33276=AXIS2_PLACEMENT_3D('',#76623,#38292,#38293);
#33277=AXIS2_PLACEMENT_3D('',#76625,#38295,#38296);
#33278=AXIS2_PLACEMENT_3D('',#76631,#38300,#38301);
#33279=AXIS2_PLACEMENT_3D('',#76633,#38302,#38303);
#33280=AXIS2_PLACEMENT_3D('',#76635,#38304,#38305);
#33281=AXIS2_PLACEMENT_3D('',#76637,#38307,#38308);
#33282=AXIS2_PLACEMENT_3D('',#76643,#38312,#38313);
#33283=AXIS2_PLACEMENT_3D('',#76644,#38314,#38315);
#33284=AXIS2_PLACEMENT_3D('',#76645,#38316,#38317);
#33285=AXIS2_PLACEMENT_3D('',#76646,#38318,#38319);
#33286=AXIS2_PLACEMENT_3D('',#76647,#38320,#38321);
#35790=DIRECTION('axis',(0.,0.,1.));
#35791=DIRECTION('refdir',(1.,0.,0.));
#35792=DIRECTION('',(-1.,0.,0.));
#35793=DIRECTION('',(-1.,0.,0.));
#35794=DIRECTION('',(-1.,0.,0.));
#35795=DIRECTION('',(-1.,0.,0.));
#35796=DIRECTION('',(-1.,0.,0.));
#35797=DIRECTION('',(-1.,0.,0.));
#35798=DIRECTION('',(-1.,0.,0.));
#35799=DIRECTION('',(-1.,0.,0.));
#35800=DIRECTION('',(-1.,0.,0.));
#35801=DIRECTION('',(-1.,0.,0.));
#35802=DIRECTION('',(-1.,0.,0.));
#35803=DIRECTION('',(-1.,0.,0.));
#35804=DIRECTION('',(-1.,0.,0.));
#35805=DIRECTION('',(-1.,0.,0.));
#35806=DIRECTION('',(-1.,0.,0.));
#35807=DIRECTION('',(-1.,0.,0.));
#35808=DIRECTION('',(-1.,0.,0.));
#35809=DIRECTION('',(-1.,0.,0.));
#35810=DIRECTION('',(-1.,0.,0.));
#35811=DIRECTION('',(-1.,0.,0.));
#35812=DIRECTION('center_axis',(1.,0.,0.));
#35813=DIRECTION('ref_axis',(0.,0.,-1.));
#35814=DIRECTION('center_axis',(0.,-0.570372452855479,-0.821386185069864));
#35815=DIRECTION('ref_axis',(0.,-0.821386185069864,0.570372452855479));
#35816=DIRECTION('',(0.,-0.821386185069864,0.570372452855479));
#35817=DIRECTION('',(-1.,0.,0.));
#35818=DIRECTION('',(0.,-0.821386185069864,0.570372452855479));
#35819=DIRECTION('',(-1.,0.,0.));
#35820=DIRECTION('center_axis',(0.,0.,1.));
#35821=DIRECTION('ref_axis',(0.,1.,0.));
#35822=DIRECTION('',(0.,1.,0.));
#35823=DIRECTION('',(-1.,0.,0.));
#35824=DIRECTION('',(0.,1.,0.));
#35825=DIRECTION('center_axis',(0.,1.,0.));
#35826=DIRECTION('ref_axis',(0.,0.,-1.));
#35827=DIRECTION('',(0.,0.,-1.));
#35828=DIRECTION('',(0.,0.,-1.));
#35829=DIRECTION('center_axis',(0.,0.,-1.));
#35830=DIRECTION('ref_axis',(0.,-1.,0.));
#35831=DIRECTION('',(0.,-1.,0.));
#35832=DIRECTION('',(-1.,0.,0.));
#35833=DIRECTION('',(0.,-1.,0.));
#35834=DIRECTION('',(-1.,0.,0.));
#35835=DIRECTION('center_axis',(0.,-1.,0.));
#35836=DIRECTION('ref_axis',(0.,0.,1.));
#35837=DIRECTION('',(0.,0.,1.));
#35838=DIRECTION('',(-1.,0.,0.));
#35839=DIRECTION('',(0.,0.,1.));
#35840=DIRECTION('center_axis',(0.,0.,-1.));
#35841=DIRECTION('ref_axis',(0.,-1.,0.));
#35842=DIRECTION('',(0.,-1.,0.));
#35843=DIRECTION('',(-1.,0.,0.));
#35844=DIRECTION('',(0.,-1.,0.));
#35845=DIRECTION('center_axis',(0.,1.,0.));
#35846=DIRECTION('ref_axis',(0.,0.,-1.));
#35847=DIRECTION('',(0.,0.,-1.));
#35848=DIRECTION('',(-1.,0.,0.));
#35849=DIRECTION('',(0.,0.,-1.));
#35850=DIRECTION('center_axis',(0.,0.,-1.));
#35851=DIRECTION('ref_axis',(0.,-1.,0.));
#35852=DIRECTION('',(0.,-1.,0.));
#35853=DIRECTION('',(-1.,0.,0.));
#35854=DIRECTION('',(0.,-1.,0.));
#35855=DIRECTION('center_axis',(0.,1.,0.));
#35856=DIRECTION('ref_axis',(0.,0.,-1.));
#35857=DIRECTION('',(0.,0.,-1.));
#35858=DIRECTION('',(-1.,0.,0.));
#35859=DIRECTION('',(0.,0.,-1.));
#35860=DIRECTION('center_axis',(0.,0.575770455267793,0.817611388644213));
#35861=DIRECTION('ref_axis',(0.,0.817611388644213,-0.575770455267793));
#35862=DIRECTION('',(0.,0.817611388644214,-0.575770455267792));
#35863=DIRECTION('',(-1.,0.,0.));
#35864=DIRECTION('',(0.,0.817611388644214,-0.575770455267792));
#35865=DIRECTION('center_axis',(0.,0.,1.));
#35866=DIRECTION('ref_axis',(0.,1.,0.));
#35867=DIRECTION('',(0.,1.,0.));
#35868=DIRECTION('',(-1.,0.,0.));
#35869=DIRECTION('',(0.,1.,0.));
#35870=DIRECTION('center_axis',(0.,-1.,0.));
#35871=DIRECTION('ref_axis',(0.,0.,1.));
#35872=DIRECTION('',(0.,0.,1.));
#35873=DIRECTION('',(-1.,0.,0.));
#35874=DIRECTION('',(0.,0.,1.));
#35875=DIRECTION('center_axis',(0.,0.,1.));
#35876=DIRECTION('ref_axis',(0.,1.,0.));
#35877=DIRECTION('',(0.,1.,0.));
#35878=DIRECTION('',(-1.,0.,0.));
#35879=DIRECTION('',(0.,1.,0.));
#35880=DIRECTION('center_axis',(0.,-1.,0.));
#35881=DIRECTION('ref_axis',(0.,0.,1.));
#35882=DIRECTION('',(0.,0.,1.));
#35883=DIRECTION('',(0.,0.,1.));
#35884=DIRECTION('center_axis',(-1.,0.,0.));
#35885=DIRECTION('ref_axis',(0.,0.,1.));
#35886=DIRECTION('center_axis',(1.,0.,0.));
#35887=DIRECTION('ref_axis',(0.,0.,-1.));
#35888=DIRECTION('center_axis',(1.,0.,0.));
#35889=DIRECTION('ref_axis',(0.,0.,-1.));
#35890=DIRECTION('',(-1.,0.,0.));
#35891=DIRECTION('',(-1.,0.,0.));
#35892=DIRECTION('',(-1.,0.,0.));
#35893=DIRECTION('',(-1.,0.,0.));
#35894=DIRECTION('',(-1.,0.,0.));
#35895=DIRECTION('',(-1.,0.,0.));
#35896=DIRECTION('',(-1.,0.,0.));
#35897=DIRECTION('',(-1.,0.,0.));
#35898=DIRECTION('',(-1.,0.,0.));
#35899=DIRECTION('',(-1.,0.,0.));
#35900=DIRECTION('',(-1.,0.,0.));
#35901=DIRECTION('',(-1.,0.,0.));
#35902=DIRECTION('',(-1.,0.,0.));
#35903=DIRECTION('',(-1.,0.,0.));
#35904=DIRECTION('',(-1.,0.,0.));
#35905=DIRECTION('',(-1.,0.,0.));
#35906=DIRECTION('',(-1.,0.,0.));
#35907=DIRECTION('',(-1.,0.,0.));
#35908=DIRECTION('',(-1.,0.,0.));
#35909=DIRECTION('',(-1.,0.,0.));
#35910=DIRECTION('center_axis',(1.,0.,0.));
#35911=DIRECTION('ref_axis',(0.,0.,-1.));
#35912=DIRECTION('',(-1.,0.,0.));
#35913=DIRECTION('',(-1.,0.,0.));
#35914=DIRECTION('',(-1.,0.,0.));
#35915=DIRECTION('',(-1.,0.,0.));
#35916=DIRECTION('',(-1.,0.,0.));
#35917=DIRECTION('',(-1.,0.,0.));
#35918=DIRECTION('',(-1.,0.,0.));
#35919=DIRECTION('',(-1.,0.,0.));
#35920=DIRECTION('',(-1.,0.,0.));
#35921=DIRECTION('',(-1.,0.,0.));
#35922=DIRECTION('',(-1.,0.,0.));
#35923=DIRECTION('',(-1.,0.,0.));
#35924=DIRECTION('',(-1.,0.,0.));
#35925=DIRECTION('center_axis',(0.,-0.984562439147349,0.175033720808942));
#35926=DIRECTION('ref_axis',(0.,0.175033720808942,0.984562439147349));
#35927=DIRECTION('',(0.,0.175033720808942,0.984562439147349));
#35928=DIRECTION('',(-1.,0.,0.));
#35929=DIRECTION('',(0.,0.175033720808942,0.984562439147349));
#35930=DIRECTION('',(-1.,0.,0.));
#35931=DIRECTION('',(-1.,0.,0.));
#35932=DIRECTION('',(-1.,0.,0.));
#35933=DIRECTION('',(-1.,0.,0.));
#35934=DIRECTION('',(-1.,0.,0.));
#35935=DIRECTION('',(-1.,0.,0.));
#35936=DIRECTION('',(-1.,0.,0.));
#35937=DIRECTION('center_axis',(0.,0.125580335944265,0.992083453759877));
#35938=DIRECTION('ref_axis',(0.,0.992083453759877,-0.125580335944265));
#35939=DIRECTION('',(0.,0.992083453759877,-0.125580335944265));
#35940=DIRECTION('',(-1.,0.,0.));
#35941=DIRECTION('',(0.,0.992083453759877,-0.125580335944265));
#35942=DIRECTION('',(-1.,0.,0.));
#35943=DIRECTION('',(-1.,0.,0.));
#35944=DIRECTION('',(-1.,0.,0.));
#35945=DIRECTION('',(-1.,0.,0.));
#35946=DIRECTION('',(-1.,0.,0.));
#35947=DIRECTION('',(-1.,0.,0.));
#35948=DIRECTION('',(-1.,0.,0.));
#35949=DIRECTION('center_axis',(0.,0.991227812035547,0.132164384942471));
#35950=DIRECTION('ref_axis',(0.,0.132164384942471,-0.991227812035547));
#35951=DIRECTION('',(0.,0.132164384942471,-0.991227812035547));
#35952=DIRECTION('',(-1.,0.,0.));
#35953=DIRECTION('',(0.,0.132164384942471,-0.991227812035547));
#35954=DIRECTION('center_axis',(1.,0.,0.));
#35955=DIRECTION('ref_axis',(0.,0.,-1.));
#35956=DIRECTION('center_axis',(1.,0.,0.));
#35957=DIRECTION('ref_axis',(0.,0.,-1.));
#35958=DIRECTION('',(-1.,0.,0.));
#35959=DIRECTION('',(-1.,0.,0.));
#35960=DIRECTION('',(-1.,0.,0.));
#35961=DIRECTION('',(-1.,0.,0.));
#35962=DIRECTION('',(-1.,0.,0.));
#35963=DIRECTION('',(-1.,0.,0.));
#35964=DIRECTION('',(-1.,0.,0.));
#35965=DIRECTION('',(-1.,0.,0.));
#35966=DIRECTION('',(-1.,0.,0.));
#35967=DIRECTION('',(-1.,0.,0.));
#35968=DIRECTION('',(-1.,0.,0.));
#35969=DIRECTION('',(-1.,0.,0.));
#35970=DIRECTION('',(-1.,0.,0.));
#35971=DIRECTION('',(-1.,0.,0.));
#35972=DIRECTION('',(-1.,0.,0.));
#35973=DIRECTION('',(-1.,0.,0.));
#35974=DIRECTION('',(-1.,0.,0.));
#35975=DIRECTION('',(-1.,0.,0.));
#35976=DIRECTION('',(-1.,0.,0.));
#35977=DIRECTION('',(-1.,0.,0.));
#35978=DIRECTION('center_axis',(1.,0.,0.));
#35979=DIRECTION('ref_axis',(0.,0.,-1.));
#35980=DIRECTION('',(-1.,0.,0.));
#35981=DIRECTION('',(-1.,0.,0.));
#35982=DIRECTION('',(-1.,0.,0.));
#35983=DIRECTION('',(-1.,0.,0.));
#35984=DIRECTION('',(-1.,0.,0.));
#35985=DIRECTION('',(-1.,0.,0.));
#35986=DIRECTION('',(-1.,0.,0.));
#35987=DIRECTION('',(-1.,0.,0.));
#35988=DIRECTION('',(-1.,0.,0.));
#35989=DIRECTION('',(-1.,0.,0.));
#35990=DIRECTION('center_axis',(0.,-0.994767480968245,0.10216486092631));
#35991=DIRECTION('ref_axis',(0.,0.10216486092631,0.994767480968245));
#35992=DIRECTION('',(0.,0.10216486092631,0.994767480968245));
#35993=DIRECTION('',(-1.,0.,0.));
#35994=DIRECTION('',(0.,0.10216486092631,0.994767480968245));
#35995=DIRECTION('',(-1.,0.,0.));
#35996=DIRECTION('',(-1.,0.,0.));
#35997=DIRECTION('',(-1.,0.,0.));
#35998=DIRECTION('',(-1.,0.,0.));
#35999=DIRECTION('',(-1.,0.,0.));
#36000=DIRECTION('',(-1.,0.,0.));
#36001=DIRECTION('',(-1.,0.,0.));
#36002=DIRECTION('',(-1.,0.,0.));
#36003=DIRECTION('',(-1.,0.,0.));
#36004=DIRECTION('center_axis',(0.,-1.,0.));
#36005=DIRECTION('ref_axis',(0.,0.,1.));
#36006=DIRECTION('',(0.,0.,1.));
#36007=DIRECTION('',(-1.,0.,0.));
#36008=DIRECTION('',(0.,0.,1.));
#36009=DIRECTION('center_axis',(0.,0.,-1.));
#36010=DIRECTION('ref_axis',(0.,-1.,0.));
#36011=DIRECTION('',(0.,-1.,0.));
#36012=DIRECTION('',(-1.,0.,0.));
#36013=DIRECTION('',(0.,-1.,0.));
#36014=DIRECTION('center_axis',(0.,1.,0.));
#36015=DIRECTION('ref_axis',(0.,0.,-1.));
#36016=DIRECTION('',(0.,0.,-1.));
#36017=DIRECTION('',(0.,0.,-1.));
#36018=DIRECTION('center_axis',(1.,0.,0.));
#36019=DIRECTION('ref_axis',(0.,0.,-1.));
#36020=DIRECTION('center_axis',(1.,0.,0.));
#36021=DIRECTION('ref_axis',(0.,0.,-1.));
#36022=DIRECTION('',(-1.,0.,0.));
#36023=DIRECTION('',(-1.,0.,0.));
#36024=DIRECTION('',(-1.,0.,0.));
#36025=DIRECTION('',(-1.,0.,0.));
#36026=DIRECTION('',(-1.,0.,0.));
#36027=DIRECTION('',(-1.,0.,0.));
#36028=DIRECTION('',(-1.,0.,0.));
#36029=DIRECTION('',(-1.,0.,0.));
#36030=DIRECTION('',(-1.,0.,0.));
#36031=DIRECTION('',(-1.,0.,0.));
#36032=DIRECTION('',(-1.,0.,0.));
#36033=DIRECTION('',(-1.,0.,0.));
#36034=DIRECTION('',(-1.,0.,0.));
#36035=DIRECTION('',(-1.,0.,0.));
#36036=DIRECTION('',(-1.,0.,0.));
#36037=DIRECTION('',(-1.,0.,0.));
#36038=DIRECTION('',(-1.,0.,0.));
#36039=DIRECTION('',(-1.,0.,0.));
#36040=DIRECTION('',(-1.,0.,0.));
#36041=DIRECTION('',(-1.,0.,0.));
#36042=DIRECTION('center_axis',(1.,0.,0.));
#36043=DIRECTION('ref_axis',(0.,0.,-1.));
#36044=DIRECTION('center_axis',(0.,1.,0.));
#36045=DIRECTION('ref_axis',(0.,0.,-1.));
#36046=DIRECTION('',(0.,0.,-1.));
#36047=DIRECTION('',(-1.,0.,0.));
#36048=DIRECTION('',(0.,0.,-1.));
#36049=DIRECTION('',(-1.,0.,0.));
#36050=DIRECTION('',(-1.,0.,0.));
#36051=DIRECTION('',(-1.,0.,0.));
#36052=DIRECTION('center_axis',(0.,0.,1.));
#36053=DIRECTION('ref_axis',(0.,1.,0.));
#36054=DIRECTION('',(0.,1.,0.));
#36055=DIRECTION('',(-1.,0.,0.));
#36056=DIRECTION('',(0.,1.,0.));
#36057=DIRECTION('',(-1.,0.,0.));
#36058=DIRECTION('',(-1.,0.,0.));
#36059=DIRECTION('center_axis',(0.,0.,1.));
#36060=DIRECTION('ref_axis',(0.,1.,0.));
#36061=DIRECTION('',(0.,1.,0.));
#36062=DIRECTION('',(-1.,0.,0.));
#36063=DIRECTION('',(0.,1.,0.));
#36064=DIRECTION('center_axis',(0.,-1.,0.));
#36065=DIRECTION('ref_axis',(0.,0.,1.));
#36066=DIRECTION('',(0.,0.,1.));
#36067=DIRECTION('',(-1.,0.,0.));
#36068=DIRECTION('',(0.,0.,1.));
#36069=DIRECTION('center_axis',(0.,0.,-1.));
#36070=DIRECTION('ref_axis',(0.,-1.,0.));
#36071=DIRECTION('',(0.,-1.,0.));
#36072=DIRECTION('',(0.,-1.,0.));
#36073=DIRECTION('center_axis',(1.,0.,0.));
#36074=DIRECTION('ref_axis',(0.,0.,-1.));
#36075=DIRECTION('center_axis',(1.,0.,0.));
#36076=DIRECTION('ref_axis',(0.,0.,-1.));
#36077=DIRECTION('',(-1.,0.,0.));
#36078=DIRECTION('',(-1.,0.,0.));
#36079=DIRECTION('',(-1.,0.,0.));
#36080=DIRECTION('',(-1.,0.,0.));
#36081=DIRECTION('',(-1.,0.,0.));
#36082=DIRECTION('',(-1.,0.,0.));
#36083=DIRECTION('',(-1.,0.,0.));
#36084=DIRECTION('',(-1.,0.,0.));
#36085=DIRECTION('',(-1.,0.,0.));
#36086=DIRECTION('',(-1.,0.,0.));
#36087=DIRECTION('',(-1.,0.,0.));
#36088=DIRECTION('',(-1.,0.,0.));
#36089=DIRECTION('',(-1.,0.,0.));
#36090=DIRECTION('',(-1.,0.,0.));
#36091=DIRECTION('',(-1.,0.,0.));
#36092=DIRECTION('',(-1.,0.,0.));
#36093=DIRECTION('',(-1.,0.,0.));
#36094=DIRECTION('',(-1.,0.,0.));
#36095=DIRECTION('',(-1.,0.,0.));
#36096=DIRECTION('',(-1.,0.,0.));
#36097=DIRECTION('center_axis',(1.,0.,0.));
#36098=DIRECTION('ref_axis',(0.,0.,-1.));
#36099=DIRECTION('center_axis',(1.,0.,0.));
#36100=DIRECTION('ref_axis',(0.,0.,-1.));
#36101=DIRECTION('',(-1.,0.,0.));
#36102=DIRECTION('',(-1.,0.,0.));
#36103=DIRECTION('',(-1.,0.,0.));
#36104=DIRECTION('',(-1.,0.,0.));
#36105=DIRECTION('',(-1.,0.,0.));
#36106=DIRECTION('',(-1.,0.,0.));
#36107=DIRECTION('',(-1.,0.,0.));
#36108=DIRECTION('',(-1.,0.,0.));
#36109=DIRECTION('',(-1.,0.,0.));
#36110=DIRECTION('',(-1.,0.,0.));
#36111=DIRECTION('',(-1.,0.,0.));
#36112=DIRECTION('',(-1.,0.,0.));
#36113=DIRECTION('',(-1.,0.,0.));
#36114=DIRECTION('',(-1.,0.,0.));
#36115=DIRECTION('',(-1.,0.,0.));
#36116=DIRECTION('',(-1.,0.,0.));
#36117=DIRECTION('',(-1.,0.,0.));
#36118=DIRECTION('',(-1.,0.,0.));
#36119=DIRECTION('',(-1.,0.,0.));
#36120=DIRECTION('',(-1.,0.,0.));
#36121=DIRECTION('center_axis',(1.,0.,0.));
#36122=DIRECTION('ref_axis',(0.,0.,-1.));
#36123=DIRECTION('center_axis',(0.,1.,0.));
#36124=DIRECTION('ref_axis',(0.,0.,-1.));
#36125=DIRECTION('',(0.,0.,-1.));
#36126=DIRECTION('',(-1.,0.,0.));
#36127=DIRECTION('',(0.,0.,-1.));
#36128=DIRECTION('',(-1.,0.,0.));
#36129=DIRECTION('',(-1.,0.,0.));
#36130=DIRECTION('',(-1.,0.,0.));
#36131=DIRECTION('center_axis',(0.,0.,1.));
#36132=DIRECTION('ref_axis',(0.,1.,0.));
#36133=DIRECTION('',(0.,1.,0.));
#36134=DIRECTION('',(-1.,0.,0.));
#36135=DIRECTION('',(0.,1.,0.));
#36136=DIRECTION('',(-1.,0.,0.));
#36137=DIRECTION('',(-1.,0.,0.));
#36138=DIRECTION('center_axis',(0.,0.,1.));
#36139=DIRECTION('ref_axis',(0.,1.,0.));
#36140=DIRECTION('',(0.,1.,0.));
#36141=DIRECTION('',(-1.,0.,0.));
#36142=DIRECTION('',(0.,1.,0.));
#36143=DIRECTION('center_axis',(0.,-1.,0.));
#36144=DIRECTION('ref_axis',(0.,0.,1.));
#36145=DIRECTION('',(0.,0.,1.));
#36146=DIRECTION('',(-1.,0.,0.));
#36147=DIRECTION('',(0.,0.,1.));
#36148=DIRECTION('center_axis',(0.,0.,-1.));
#36149=DIRECTION('ref_axis',(0.,-1.,0.));
#36150=DIRECTION('',(0.,-1.,0.));
#36151=DIRECTION('',(0.,-1.,0.));
#36152=DIRECTION('center_axis',(1.,0.,0.));
#36153=DIRECTION('ref_axis',(0.,0.,-1.));
#36154=DIRECTION('center_axis',(1.,0.,0.));
#36155=DIRECTION('ref_axis',(0.,0.,-1.));
#36156=DIRECTION('',(-1.,0.,0.));
#36157=DIRECTION('',(-1.,0.,0.));
#36158=DIRECTION('',(-1.,0.,0.));
#36159=DIRECTION('',(-1.,0.,0.));
#36160=DIRECTION('',(-1.,0.,0.));
#36161=DIRECTION('',(-1.,0.,0.));
#36162=DIRECTION('',(-1.,0.,0.));
#36163=DIRECTION('',(-1.,0.,0.));
#36164=DIRECTION('',(-1.,0.,0.));
#36165=DIRECTION('',(-1.,0.,0.));
#36166=DIRECTION('',(-1.,0.,0.));
#36167=DIRECTION('',(-1.,0.,0.));
#36168=DIRECTION('',(-1.,0.,0.));
#36169=DIRECTION('',(-1.,0.,0.));
#36170=DIRECTION('',(-1.,0.,0.));
#36171=DIRECTION('',(-1.,0.,0.));
#36172=DIRECTION('',(-1.,0.,0.));
#36173=DIRECTION('',(-1.,0.,0.));
#36174=DIRECTION('',(-1.,0.,0.));
#36175=DIRECTION('',(-1.,0.,0.));
#36176=DIRECTION('center_axis',(1.,0.,0.));
#36177=DIRECTION('ref_axis',(0.,0.,-1.));
#36178=DIRECTION('',(-1.,0.,0.));
#36179=DIRECTION('',(-1.,0.,0.));
#36180=DIRECTION('',(-1.,0.,0.));
#36181=DIRECTION('',(-1.,0.,0.));
#36182=DIRECTION('',(-1.,0.,0.));
#36183=DIRECTION('',(-1.,0.,0.));
#36184=DIRECTION('',(-1.,0.,0.));
#36185=DIRECTION('',(-1.,0.,0.));
#36186=DIRECTION('',(-1.,0.,0.));
#36187=DIRECTION('',(-1.,0.,0.));
#36188=DIRECTION('center_axis',(0.,-0.994767480968245,0.10216486092631));
#36189=DIRECTION('ref_axis',(0.,0.10216486092631,0.994767480968245));
#36190=DIRECTION('',(0.,0.10216486092631,0.994767480968245));
#36191=DIRECTION('',(-1.,0.,0.));
#36192=DIRECTION('',(0.,0.10216486092631,0.994767480968245));
#36193=DIRECTION('',(-1.,0.,0.));
#36194=DIRECTION('',(-1.,0.,0.));
#36195=DIRECTION('',(-1.,0.,0.));
#36196=DIRECTION('',(-1.,0.,0.));
#36197=DIRECTION('',(-1.,0.,0.));
#36198=DIRECTION('',(-1.,0.,0.));
#36199=DIRECTION('',(-1.,0.,0.));
#36200=DIRECTION('',(-1.,0.,0.));
#36201=DIRECTION('',(-1.,0.,0.));
#36202=DIRECTION('center_axis',(0.,-1.,0.));
#36203=DIRECTION('ref_axis',(0.,0.,1.));
#36204=DIRECTION('',(0.,0.,1.));
#36205=DIRECTION('',(-1.,0.,0.));
#36206=DIRECTION('',(0.,0.,1.));
#36207=DIRECTION('center_axis',(0.,0.,-1.));
#36208=DIRECTION('ref_axis',(0.,-1.,0.));
#36209=DIRECTION('',(0.,-1.,0.));
#36210=DIRECTION('',(-1.,0.,0.));
#36211=DIRECTION('',(0.,-1.,0.));
#36212=DIRECTION('center_axis',(0.,1.,0.));
#36213=DIRECTION('ref_axis',(0.,0.,-1.));
#36214=DIRECTION('',(0.,0.,-1.));
#36215=DIRECTION('',(0.,0.,-1.));
#36216=DIRECTION('center_axis',(1.,0.,0.));
#36217=DIRECTION('ref_axis',(0.,0.,-1.));
#36218=DIRECTION('center_axis',(1.,0.,0.));
#36219=DIRECTION('ref_axis',(0.,0.,-1.));
#36220=DIRECTION('',(-1.,0.,0.));
#36221=DIRECTION('',(-1.,0.,0.));
#36222=DIRECTION('',(-1.,0.,0.));
#36223=DIRECTION('',(-1.,0.,0.));
#36224=DIRECTION('',(-1.,0.,0.));
#36225=DIRECTION('',(-1.,0.,0.));
#36226=DIRECTION('',(-1.,0.,0.));
#36227=DIRECTION('',(-1.,0.,0.));
#36228=DIRECTION('',(-1.,0.,0.));
#36229=DIRECTION('',(-1.,0.,0.));
#36230=DIRECTION('',(-1.,0.,0.));
#36231=DIRECTION('',(-1.,0.,0.));
#36232=DIRECTION('',(-1.,0.,0.));
#36233=DIRECTION('',(-1.,0.,0.));
#36234=DIRECTION('',(-1.,0.,0.));
#36235=DIRECTION('',(-1.,0.,0.));
#36236=DIRECTION('',(-1.,0.,0.));
#36237=DIRECTION('',(-1.,0.,0.));
#36238=DIRECTION('',(-1.,0.,0.));
#36239=DIRECTION('',(-1.,0.,0.));
#36240=DIRECTION('center_axis',(1.,0.,0.));
#36241=DIRECTION('ref_axis',(0.,0.,-1.));
#36242=DIRECTION('',(-1.,0.,0.));
#36243=DIRECTION('',(-1.,0.,0.));
#36244=DIRECTION('',(-1.,0.,0.));
#36245=DIRECTION('',(-1.,0.,0.));
#36246=DIRECTION('',(-1.,0.,0.));
#36247=DIRECTION('',(-1.,0.,0.));
#36248=DIRECTION('',(-1.,0.,0.));
#36249=DIRECTION('',(-1.,0.,0.));
#36250=DIRECTION('',(-1.,0.,0.));
#36251=DIRECTION('',(-1.,0.,0.));
#36252=DIRECTION('',(-1.,0.,0.));
#36253=DIRECTION('',(-1.,0.,0.));
#36254=DIRECTION('',(-1.,0.,0.));
#36255=DIRECTION('center_axis',(0.,-0.984562439147349,0.175033720808942));
#36256=DIRECTION('ref_axis',(0.,0.175033720808942,0.984562439147349));
#36257=DIRECTION('',(0.,0.175033720808942,0.984562439147349));
#36258=DIRECTION('',(-1.,0.,0.));
#36259=DIRECTION('',(0.,0.175033720808942,0.984562439147349));
#36260=DIRECTION('',(-1.,0.,0.));
#36261=DIRECTION('',(-1.,0.,0.));
#36262=DIRECTION('',(-1.,0.,0.));
#36263=DIRECTION('',(-1.,0.,0.));
#36264=DIRECTION('',(-1.,0.,0.));
#36265=DIRECTION('',(-1.,0.,0.));
#36266=DIRECTION('',(-1.,0.,0.));
#36267=DIRECTION('center_axis',(0.,0.125580335944265,0.992083453759877));
#36268=DIRECTION('ref_axis',(0.,0.992083453759877,-0.125580335944265));
#36269=DIRECTION('',(0.,0.992083453759877,-0.125580335944265));
#36270=DIRECTION('',(-1.,0.,0.));
#36271=DIRECTION('',(0.,0.992083453759877,-0.125580335944265));
#36272=DIRECTION('',(-1.,0.,0.));
#36273=DIRECTION('',(-1.,0.,0.));
#36274=DIRECTION('',(-1.,0.,0.));
#36275=DIRECTION('',(-1.,0.,0.));
#36276=DIRECTION('',(-1.,0.,0.));
#36277=DIRECTION('',(-1.,0.,0.));
#36278=DIRECTION('',(-1.,0.,0.));
#36279=DIRECTION('center_axis',(0.,0.991227812035547,0.132164384942471));
#36280=DIRECTION('ref_axis',(0.,0.132164384942471,-0.991227812035547));
#36281=DIRECTION('',(0.,0.132164384942471,-0.991227812035547));
#36282=DIRECTION('',(-1.,0.,0.));
#36283=DIRECTION('',(0.,0.132164384942471,-0.991227812035547));
#36284=DIRECTION('center_axis',(1.,0.,0.));
#36285=DIRECTION('ref_axis',(0.,0.,-1.));
#36286=DIRECTION('center_axis',(1.,0.,0.));
#36287=DIRECTION('ref_axis',(0.,0.,-1.));
#36288=DIRECTION('',(-1.,0.,0.));
#36289=DIRECTION('',(-1.,0.,0.));
#36290=DIRECTION('',(-1.,0.,0.));
#36291=DIRECTION('',(-1.,0.,0.));
#36292=DIRECTION('',(-1.,0.,0.));
#36293=DIRECTION('',(-1.,0.,0.));
#36294=DIRECTION('',(-1.,0.,0.));
#36295=DIRECTION('',(-1.,0.,0.));
#36296=DIRECTION('',(-1.,0.,0.));
#36297=DIRECTION('',(-1.,0.,0.));
#36298=DIRECTION('',(-1.,0.,0.));
#36299=DIRECTION('',(-1.,0.,0.));
#36300=DIRECTION('',(-1.,0.,0.));
#36301=DIRECTION('',(-1.,0.,0.));
#36302=DIRECTION('',(-1.,0.,0.));
#36303=DIRECTION('',(-1.,0.,0.));
#36304=DIRECTION('',(-1.,0.,0.));
#36305=DIRECTION('',(-1.,0.,0.));
#36306=DIRECTION('',(-1.,0.,0.));
#36307=DIRECTION('',(-1.,0.,0.));
#36308=DIRECTION('center_axis',(1.,0.,0.));
#36309=DIRECTION('ref_axis',(0.,0.,-1.));
#36310=DIRECTION('center_axis',(0.,-0.570372452855479,-0.821386185069864));
#36311=DIRECTION('ref_axis',(0.,-0.821386185069864,0.570372452855479));
#36312=DIRECTION('',(0.,-0.821386185069864,0.570372452855479));
#36313=DIRECTION('',(-1.,0.,0.));
#36314=DIRECTION('',(0.,-0.821386185069864,0.570372452855479));
#36315=DIRECTION('',(-1.,0.,0.));
#36316=DIRECTION('center_axis',(0.,0.,1.));
#36317=DIRECTION('ref_axis',(0.,1.,0.));
#36318=DIRECTION('',(0.,1.,0.));
#36319=DIRECTION('',(-1.,0.,0.));
#36320=DIRECTION('',(0.,1.,0.));
#36321=DIRECTION('center_axis',(0.,1.,0.));
#36322=DIRECTION('ref_axis',(0.,0.,-1.));
#36323=DIRECTION('',(0.,0.,-1.));
#36324=DIRECTION('',(0.,0.,-1.));
#36325=DIRECTION('center_axis',(0.,0.,-1.));
#36326=DIRECTION('ref_axis',(0.,-1.,0.));
#36327=DIRECTION('',(0.,-1.,0.));
#36328=DIRECTION('',(-1.,0.,0.));
#36329=DIRECTION('',(0.,-1.,0.));
#36330=DIRECTION('',(-1.,0.,0.));
#36331=DIRECTION('center_axis',(0.,-1.,0.));
#36332=DIRECTION('ref_axis',(0.,0.,1.));
#36333=DIRECTION('',(0.,0.,1.));
#36334=DIRECTION('',(-1.,0.,0.));
#36335=DIRECTION('',(0.,0.,1.));
#36336=DIRECTION('center_axis',(0.,0.,-1.));
#36337=DIRECTION('ref_axis',(0.,-1.,0.));
#36338=DIRECTION('',(0.,-1.,0.));
#36339=DIRECTION('',(-1.,0.,0.));
#36340=DIRECTION('',(0.,-1.,0.));
#36341=DIRECTION('center_axis',(0.,1.,0.));
#36342=DIRECTION('ref_axis',(0.,0.,-1.));
#36343=DIRECTION('',(0.,0.,-1.));
#36344=DIRECTION('',(-1.,0.,0.));
#36345=DIRECTION('',(0.,0.,-1.));
#36346=DIRECTION('center_axis',(0.,0.,-1.));
#36347=DIRECTION('ref_axis',(0.,-1.,0.));
#36348=DIRECTION('',(0.,-1.,0.));
#36349=DIRECTION('',(-1.,0.,0.));
#36350=DIRECTION('',(0.,-1.,0.));
#36351=DIRECTION('center_axis',(0.,1.,0.));
#36352=DIRECTION('ref_axis',(0.,0.,-1.));
#36353=DIRECTION('',(0.,0.,-1.));
#36354=DIRECTION('',(-1.,0.,0.));
#36355=DIRECTION('',(0.,0.,-1.));
#36356=DIRECTION('center_axis',(0.,0.575770455267793,0.817611388644213));
#36357=DIRECTION('ref_axis',(0.,0.817611388644213,-0.575770455267793));
#36358=DIRECTION('',(0.,0.817611388644214,-0.575770455267792));
#36359=DIRECTION('',(-1.,0.,0.));
#36360=DIRECTION('',(0.,0.817611388644214,-0.575770455267792));
#36361=DIRECTION('center_axis',(0.,0.,1.));
#36362=DIRECTION('ref_axis',(0.,1.,0.));
#36363=DIRECTION('',(0.,1.,0.));
#36364=DIRECTION('',(-1.,0.,0.));
#36365=DIRECTION('',(0.,1.,0.));
#36366=DIRECTION('center_axis',(0.,-1.,0.));
#36367=DIRECTION('ref_axis',(0.,0.,1.));
#36368=DIRECTION('',(0.,0.,1.));
#36369=DIRECTION('',(-1.,0.,0.));
#36370=DIRECTION('',(0.,0.,1.));
#36371=DIRECTION('center_axis',(0.,0.,1.));
#36372=DIRECTION('ref_axis',(0.,1.,0.));
#36373=DIRECTION('',(0.,1.,0.));
#36374=DIRECTION('',(-1.,0.,0.));
#36375=DIRECTION('',(0.,1.,0.));
#36376=DIRECTION('center_axis',(0.,-1.,0.));
#36377=DIRECTION('ref_axis',(0.,0.,1.));
#36378=DIRECTION('',(0.,0.,1.));
#36379=DIRECTION('',(0.,0.,1.));
#36380=DIRECTION('center_axis',(-1.,0.,0.));
#36381=DIRECTION('ref_axis',(0.,0.,1.));
#36382=DIRECTION('center_axis',(1.,0.,0.));
#36383=DIRECTION('ref_axis',(0.,0.,-1.));
#36384=DIRECTION('center_axis',(1.,0.,0.));
#36385=DIRECTION('ref_axis',(0.,0.,-1.));
#36386=DIRECTION('center_axis',(0.,0.,-1.));
#36387=DIRECTION('ref_axis',(0.,-1.,0.));
#36388=DIRECTION('',(0.,-1.,0.));
#36389=DIRECTION('',(-1.,0.,0.));
#36390=DIRECTION('',(0.,-1.,0.));
#36391=DIRECTION('',(-1.,0.,0.));
#36392=DIRECTION('center_axis',(0.,1.,0.));
#36393=DIRECTION('ref_axis',(0.,0.,-1.));
#36394=DIRECTION('',(0.,0.,-1.));
#36395=DIRECTION('',(-1.,0.,0.));
#36396=DIRECTION('',(0.,0.,-1.));
#36397=DIRECTION('center_axis',(0.,0.,1.));
#36398=DIRECTION('ref_axis',(0.,1.,0.));
#36399=DIRECTION('',(0.,1.,0.));
#36400=DIRECTION('',(-1.,0.,0.));
#36401=DIRECTION('',(0.,1.,0.));
#36402=DIRECTION('center_axis',(0.,-1.,0.));
#36403=DIRECTION('ref_axis',(0.,0.,1.));
#36404=DIRECTION('',(0.,0.,1.));
#36405=DIRECTION('',(0.,0.,1.));
#36406=DIRECTION('center_axis',(-1.,0.,0.));
#36407=DIRECTION('ref_axis',(0.,0.,1.));
#36408=DIRECTION('center_axis',(0.,0.,-1.));
#36409=DIRECTION('ref_axis',(0.,-1.,0.));
#36410=DIRECTION('',(0.,-1.,0.));
#36411=DIRECTION('',(-1.,0.,0.));
#36412=DIRECTION('',(0.,-1.,0.));
#36413=DIRECTION('',(-1.,0.,0.));
#36414=DIRECTION('center_axis',(0.,1.,0.));
#36415=DIRECTION('ref_axis',(0.,0.,-1.));
#36416=DIRECTION('',(0.,0.,-1.));
#36417=DIRECTION('',(-1.,0.,0.));
#36418=DIRECTION('',(0.,0.,-1.));
#36419=DIRECTION('center_axis',(0.,0.,1.));
#36420=DIRECTION('ref_axis',(0.,1.,0.));
#36421=DIRECTION('',(0.,1.,0.));
#36422=DIRECTION('',(-1.,0.,0.));
#36423=DIRECTION('',(0.,1.,0.));
#36424=DIRECTION('center_axis',(0.,-1.,0.));
#36425=DIRECTION('ref_axis',(0.,0.,1.));
#36426=DIRECTION('',(0.,0.,1.));
#36427=DIRECTION('',(0.,0.,1.));
#36428=DIRECTION('center_axis',(-1.,0.,0.));
#36429=DIRECTION('ref_axis',(0.,0.,1.));
#36430=DIRECTION('center_axis',(0.,0.,-1.));
#36431=DIRECTION('ref_axis',(0.,-1.,0.));
#36432=DIRECTION('',(0.,-1.,0.));
#36433=DIRECTION('',(-1.,0.,0.));
#36434=DIRECTION('',(0.,-1.,0.));
#36435=DIRECTION('',(-1.,0.,0.));
#36436=DIRECTION('center_axis',(0.,1.,0.));
#36437=DIRECTION('ref_axis',(0.,0.,-1.));
#36438=DIRECTION('',(0.,0.,-1.));
#36439=DIRECTION('',(-1.,0.,0.));
#36440=DIRECTION('',(0.,0.,-1.));
#36441=DIRECTION('center_axis',(0.,0.,1.));
#36442=DIRECTION('ref_axis',(0.,1.,0.));
#36443=DIRECTION('',(0.,1.,0.));
#36444=DIRECTION('',(-1.,0.,0.));
#36445=DIRECTION('',(0.,1.,0.));
#36446=DIRECTION('center_axis',(0.,-1.,0.));
#36447=DIRECTION('ref_axis',(0.,0.,1.));
#36448=DIRECTION('',(0.,0.,1.));
#36449=DIRECTION('',(0.,0.,1.));
#36450=DIRECTION('center_axis',(-1.,0.,0.));
#36451=DIRECTION('ref_axis',(0.,0.,1.));
#36452=DIRECTION('center_axis',(0.,0.,-1.));
#36453=DIRECTION('ref_axis',(0.,-1.,0.));
#36454=DIRECTION('',(0.,-1.,0.));
#36455=DIRECTION('',(-1.,0.,0.));
#36456=DIRECTION('',(0.,-1.,0.));
#36457=DIRECTION('',(-1.,0.,0.));
#36458=DIRECTION('center_axis',(0.,1.,0.));
#36459=DIRECTION('ref_axis',(0.,0.,-1.));
#36460=DIRECTION('',(0.,0.,-1.));
#36461=DIRECTION('',(-1.,0.,0.));
#36462=DIRECTION('',(0.,0.,-1.));
#36463=DIRECTION('center_axis',(0.,0.,1.));
#36464=DIRECTION('ref_axis',(0.,1.,0.));
#36465=DIRECTION('',(0.,1.,0.));
#36466=DIRECTION('',(-1.,0.,0.));
#36467=DIRECTION('',(0.,1.,0.));
#36468=DIRECTION('center_axis',(0.,-1.,0.));
#36469=DIRECTION('ref_axis',(0.,0.,1.));
#36470=DIRECTION('',(0.,0.,1.));
#36471=DIRECTION('',(0.,0.,1.));
#36472=DIRECTION('center_axis',(-1.,0.,0.));
#36473=DIRECTION('ref_axis',(0.,0.,1.));
#36474=DIRECTION('center_axis',(0.,0.,-1.));
#36475=DIRECTION('ref_axis',(0.,-1.,0.));
#36476=DIRECTION('',(0.,-1.,0.));
#36477=DIRECTION('',(-1.,0.,0.));
#36478=DIRECTION('',(0.,-1.,0.));
#36479=DIRECTION('',(-1.,0.,0.));
#36480=DIRECTION('center_axis',(0.,1.,0.));
#36481=DIRECTION('ref_axis',(0.,0.,-1.));
#36482=DIRECTION('',(0.,0.,-1.));
#36483=DIRECTION('',(-1.,0.,0.));
#36484=DIRECTION('',(0.,0.,-1.));
#36485=DIRECTION('center_axis',(0.,0.,1.));
#36486=DIRECTION('ref_axis',(0.,1.,0.));
#36487=DIRECTION('',(0.,1.,0.));
#36488=DIRECTION('',(-1.,0.,0.));
#36489=DIRECTION('',(0.,1.,0.));
#36490=DIRECTION('center_axis',(0.,-1.,0.));
#36491=DIRECTION('ref_axis',(0.,0.,1.));
#36492=DIRECTION('',(0.,0.,1.));
#36493=DIRECTION('',(0.,0.,1.));
#36494=DIRECTION('center_axis',(-1.,0.,0.));
#36495=DIRECTION('ref_axis',(0.,0.,1.));
#36496=DIRECTION('center_axis',(0.,0.,-1.));
#36497=DIRECTION('ref_axis',(0.,-1.,0.));
#36498=DIRECTION('',(0.,-1.,0.));
#36499=DIRECTION('',(-1.,0.,0.));
#36500=DIRECTION('',(0.,-1.,0.));
#36501=DIRECTION('',(-1.,0.,0.));
#36502=DIRECTION('center_axis',(0.,1.,0.));
#36503=DIRECTION('ref_axis',(0.,0.,-1.));
#36504=DIRECTION('',(0.,0.,-1.));
#36505=DIRECTION('',(-1.,0.,0.));
#36506=DIRECTION('',(0.,0.,-1.));
#36507=DIRECTION('center_axis',(0.,0.,1.));
#36508=DIRECTION('ref_axis',(0.,1.,0.));
#36509=DIRECTION('',(0.,1.,0.));
#36510=DIRECTION('',(-1.,0.,0.));
#36511=DIRECTION('',(0.,1.,0.));
#36512=DIRECTION('center_axis',(0.,-1.,0.));
#36513=DIRECTION('ref_axis',(0.,0.,1.));
#36514=DIRECTION('',(0.,0.,1.));
#36515=DIRECTION('',(0.,0.,1.));
#36516=DIRECTION('center_axis',(-1.,0.,0.));
#36517=DIRECTION('ref_axis',(0.,0.,1.));
#36518=DIRECTION('center_axis',(0.,0.,-1.));
#36519=DIRECTION('ref_axis',(0.,-1.,0.));
#36520=DIRECTION('',(0.,-1.,0.));
#36521=DIRECTION('',(-1.,0.,0.));
#36522=DIRECTION('',(0.,-1.,0.));
#36523=DIRECTION('',(-1.,0.,0.));
#36524=DIRECTION('center_axis',(0.,1.,0.));
#36525=DIRECTION('ref_axis',(0.,0.,-1.));
#36526=DIRECTION('',(0.,0.,-1.));
#36527=DIRECTION('',(-1.,0.,0.));
#36528=DIRECTION('',(0.,0.,-1.));
#36529=DIRECTION('center_axis',(0.,0.,1.));
#36530=DIRECTION('ref_axis',(0.,1.,0.));
#36531=DIRECTION('',(0.,1.,0.));
#36532=DIRECTION('',(-1.,0.,0.));
#36533=DIRECTION('',(0.,1.,0.));
#36534=DIRECTION('center_axis',(0.,-1.,0.));
#36535=DIRECTION('ref_axis',(0.,0.,1.));
#36536=DIRECTION('',(0.,0.,1.));
#36537=DIRECTION('',(0.,0.,1.));
#36538=DIRECTION('center_axis',(-1.,0.,0.));
#36539=DIRECTION('ref_axis',(0.,0.,1.));
#36540=DIRECTION('center_axis',(0.,0.,-1.));
#36541=DIRECTION('ref_axis',(0.,-1.,0.));
#36542=DIRECTION('',(0.,-1.,0.));
#36543=DIRECTION('',(-1.,0.,0.));
#36544=DIRECTION('',(0.,-1.,0.));
#36545=DIRECTION('',(-1.,0.,0.));
#36546=DIRECTION('center_axis',(0.,1.,0.));
#36547=DIRECTION('ref_axis',(0.,0.,-1.));
#36548=DIRECTION('',(0.,0.,-1.));
#36549=DIRECTION('',(-1.,0.,0.));
#36550=DIRECTION('',(0.,0.,-1.));
#36551=DIRECTION('center_axis',(0.,0.,1.));
#36552=DIRECTION('ref_axis',(0.,1.,0.));
#36553=DIRECTION('',(0.,1.,0.));
#36554=DIRECTION('',(-1.,0.,0.));
#36555=DIRECTION('',(0.,1.,0.));
#36556=DIRECTION('center_axis',(0.,-1.,0.));
#36557=DIRECTION('ref_axis',(0.,0.,1.));
#36558=DIRECTION('',(0.,0.,1.));
#36559=DIRECTION('',(0.,0.,1.));
#36560=DIRECTION('center_axis',(-1.,0.,0.));
#36561=DIRECTION('ref_axis',(0.,0.,1.));
#36562=DIRECTION('center_axis',(0.,0.,-1.));
#36563=DIRECTION('ref_axis',(0.,-1.,0.));
#36564=DIRECTION('',(0.,-1.,0.));
#36565=DIRECTION('',(-1.,0.,0.));
#36566=DIRECTION('',(0.,-1.,0.));
#36567=DIRECTION('',(-1.,0.,0.));
#36568=DIRECTION('center_axis',(0.,1.,0.));
#36569=DIRECTION('ref_axis',(0.,0.,-1.));
#36570=DIRECTION('',(0.,0.,-1.));
#36571=DIRECTION('',(-1.,0.,0.));
#36572=DIRECTION('',(0.,0.,-1.));
#36573=DIRECTION('center_axis',(0.,0.,1.));
#36574=DIRECTION('ref_axis',(0.,1.,0.));
#36575=DIRECTION('',(0.,1.,0.));
#36576=DIRECTION('',(-1.,0.,0.));
#36577=DIRECTION('',(0.,1.,0.));
#36578=DIRECTION('center_axis',(0.,-1.,0.));
#36579=DIRECTION('ref_axis',(0.,0.,1.));
#36580=DIRECTION('',(0.,0.,1.));
#36581=DIRECTION('',(0.,0.,1.));
#36582=DIRECTION('center_axis',(-1.,0.,0.));
#36583=DIRECTION('ref_axis',(0.,0.,1.));
#36584=DIRECTION('center_axis',(0.,0.,-1.));
#36585=DIRECTION('ref_axis',(0.,-1.,0.));
#36586=DIRECTION('',(0.,-1.,0.));
#36587=DIRECTION('',(-1.,0.,0.));
#36588=DIRECTION('',(0.,-1.,0.));
#36589=DIRECTION('',(-1.,0.,0.));
#36590=DIRECTION('center_axis',(0.,1.,0.));
#36591=DIRECTION('ref_axis',(0.,0.,-1.));
#36592=DIRECTION('',(0.,0.,-1.));
#36593=DIRECTION('',(-1.,0.,0.));
#36594=DIRECTION('',(0.,0.,-1.));
#36595=DIRECTION('center_axis',(0.,0.,1.));
#36596=DIRECTION('ref_axis',(0.,1.,0.));
#36597=DIRECTION('',(0.,1.,0.));
#36598=DIRECTION('',(-1.,0.,0.));
#36599=DIRECTION('',(0.,1.,0.));
#36600=DIRECTION('center_axis',(0.,-1.,0.));
#36601=DIRECTION('ref_axis',(0.,0.,1.));
#36602=DIRECTION('',(0.,0.,1.));
#36603=DIRECTION('',(0.,0.,1.));
#36604=DIRECTION('center_axis',(-1.,0.,0.));
#36605=DIRECTION('ref_axis',(0.,0.,1.));
#36606=DIRECTION('center_axis',(0.,0.,-1.));
#36607=DIRECTION('ref_axis',(0.,-1.,0.));
#36608=DIRECTION('',(0.,-1.,0.));
#36609=DIRECTION('',(-1.,0.,0.));
#36610=DIRECTION('',(0.,-1.,0.));
#36611=DIRECTION('',(-1.,0.,0.));
#36612=DIRECTION('center_axis',(0.,1.,0.));
#36613=DIRECTION('ref_axis',(0.,0.,-1.));
#36614=DIRECTION('',(0.,0.,-1.));
#36615=DIRECTION('',(-1.,0.,0.));
#36616=DIRECTION('',(0.,0.,-1.));
#36617=DIRECTION('center_axis',(0.,0.,1.));
#36618=DIRECTION('ref_axis',(0.,1.,0.));
#36619=DIRECTION('',(0.,1.,0.));
#36620=DIRECTION('',(-1.,0.,0.));
#36621=DIRECTION('',(0.,1.,0.));
#36622=DIRECTION('center_axis',(0.,-1.,0.));
#36623=DIRECTION('ref_axis',(0.,0.,1.));
#36624=DIRECTION('',(0.,0.,1.));
#36625=DIRECTION('',(0.,0.,1.));
#36626=DIRECTION('center_axis',(-1.,0.,0.));
#36627=DIRECTION('ref_axis',(0.,0.,1.));
#36628=DIRECTION('center_axis',(0.,0.,-1.));
#36629=DIRECTION('ref_axis',(0.,-1.,0.));
#36630=DIRECTION('',(0.,-1.,0.));
#36631=DIRECTION('',(-1.,0.,0.));
#36632=DIRECTION('',(0.,-1.,0.));
#36633=DIRECTION('',(-1.,0.,0.));
#36634=DIRECTION('center_axis',(0.,1.,0.));
#36635=DIRECTION('ref_axis',(0.,0.,-1.));
#36636=DIRECTION('',(0.,0.,-1.));
#36637=DIRECTION('',(-1.,0.,0.));
#36638=DIRECTION('',(0.,0.,-1.));
#36639=DIRECTION('center_axis',(0.,0.,1.));
#36640=DIRECTION('ref_axis',(0.,1.,0.));
#36641=DIRECTION('',(0.,1.,0.));
#36642=DIRECTION('',(-1.,0.,0.));
#36643=DIRECTION('',(0.,1.,0.));
#36644=DIRECTION('center_axis',(0.,-1.,0.));
#36645=DIRECTION('ref_axis',(0.,0.,1.));
#36646=DIRECTION('',(0.,0.,1.));
#36647=DIRECTION('',(0.,0.,1.));
#36648=DIRECTION('center_axis',(-1.,0.,0.));
#36649=DIRECTION('ref_axis',(0.,0.,1.));
#36650=DIRECTION('center_axis',(0.,0.,-1.));
#36651=DIRECTION('ref_axis',(0.,-1.,0.));
#36652=DIRECTION('',(0.,-1.,0.));
#36653=DIRECTION('',(-1.,0.,0.));
#36654=DIRECTION('',(0.,-1.,0.));
#36655=DIRECTION('',(-1.,0.,0.));
#36656=DIRECTION('center_axis',(0.,1.,0.));
#36657=DIRECTION('ref_axis',(0.,0.,-1.));
#36658=DIRECTION('',(0.,0.,-1.));
#36659=DIRECTION('',(-1.,0.,0.));
#36660=DIRECTION('',(0.,0.,-1.));
#36661=DIRECTION('center_axis',(0.,0.,1.));
#36662=DIRECTION('ref_axis',(0.,1.,0.));
#36663=DIRECTION('',(0.,1.,0.));
#36664=DIRECTION('',(-1.,0.,0.));
#36665=DIRECTION('',(0.,1.,0.));
#36666=DIRECTION('center_axis',(0.,-1.,0.));
#36667=DIRECTION('ref_axis',(0.,0.,1.));
#36668=DIRECTION('',(0.,0.,1.));
#36669=DIRECTION('',(0.,0.,1.));
#36670=DIRECTION('center_axis',(-1.,0.,0.));
#36671=DIRECTION('ref_axis',(0.,0.,1.));
#36672=DIRECTION('center_axis',(0.,0.,-1.));
#36673=DIRECTION('ref_axis',(0.,-1.,0.));
#36674=DIRECTION('',(0.,-1.,0.));
#36675=DIRECTION('',(-1.,0.,0.));
#36676=DIRECTION('',(0.,-1.,0.));
#36677=DIRECTION('',(-1.,0.,0.));
#36678=DIRECTION('center_axis',(0.,1.,0.));
#36679=DIRECTION('ref_axis',(0.,0.,-1.));
#36680=DIRECTION('',(0.,0.,-1.));
#36681=DIRECTION('',(-1.,0.,0.));
#36682=DIRECTION('',(0.,0.,-1.));
#36683=DIRECTION('center_axis',(0.,0.,1.));
#36684=DIRECTION('ref_axis',(0.,1.,0.));
#36685=DIRECTION('',(0.,1.,0.));
#36686=DIRECTION('',(-1.,0.,0.));
#36687=DIRECTION('',(0.,1.,0.));
#36688=DIRECTION('center_axis',(0.,-1.,0.));
#36689=DIRECTION('ref_axis',(0.,0.,1.));
#36690=DIRECTION('',(0.,0.,1.));
#36691=DIRECTION('',(0.,0.,1.));
#36692=DIRECTION('center_axis',(-1.,0.,0.));
#36693=DIRECTION('ref_axis',(0.,0.,1.));
#36694=DIRECTION('center_axis',(0.,0.,-1.));
#36695=DIRECTION('ref_axis',(0.,-1.,0.));
#36696=DIRECTION('',(0.,-1.,0.));
#36697=DIRECTION('',(-1.,0.,0.));
#36698=DIRECTION('',(0.,-1.,0.));
#36699=DIRECTION('',(-1.,0.,0.));
#36700=DIRECTION('center_axis',(0.,1.,0.));
#36701=DIRECTION('ref_axis',(0.,0.,-1.));
#36702=DIRECTION('',(0.,0.,-1.));
#36703=DIRECTION('',(-1.,0.,0.));
#36704=DIRECTION('',(0.,0.,-1.));
#36705=DIRECTION('center_axis',(0.,0.,1.));
#36706=DIRECTION('ref_axis',(0.,1.,0.));
#36707=DIRECTION('',(0.,1.,0.));
#36708=DIRECTION('',(-1.,0.,0.));
#36709=DIRECTION('',(0.,1.,0.));
#36710=DIRECTION('center_axis',(0.,-1.,0.));
#36711=DIRECTION('ref_axis',(0.,0.,1.));
#36712=DIRECTION('',(0.,0.,1.));
#36713=DIRECTION('',(0.,0.,1.));
#36714=DIRECTION('center_axis',(-1.,0.,0.));
#36715=DIRECTION('ref_axis',(0.,0.,1.));
#36716=DIRECTION('center_axis',(0.,0.,-1.));
#36717=DIRECTION('ref_axis',(0.,-1.,0.));
#36718=DIRECTION('',(0.,-1.,0.));
#36719=DIRECTION('',(-1.,0.,0.));
#36720=DIRECTION('',(0.,-1.,0.));
#36721=DIRECTION('',(-1.,0.,0.));
#36722=DIRECTION('center_axis',(0.,1.,0.));
#36723=DIRECTION('ref_axis',(0.,0.,-1.));
#36724=DIRECTION('',(0.,0.,-1.));
#36725=DIRECTION('',(-1.,0.,0.));
#36726=DIRECTION('',(0.,0.,-1.));
#36727=DIRECTION('center_axis',(0.,0.,1.));
#36728=DIRECTION('ref_axis',(0.,1.,0.));
#36729=DIRECTION('',(0.,1.,0.));
#36730=DIRECTION('',(-1.,0.,0.));
#36731=DIRECTION('',(0.,1.,0.));
#36732=DIRECTION('center_axis',(0.,-1.,0.));
#36733=DIRECTION('ref_axis',(0.,0.,1.));
#36734=DIRECTION('',(0.,0.,1.));
#36735=DIRECTION('',(0.,0.,1.));
#36736=DIRECTION('center_axis',(-1.,0.,0.));
#36737=DIRECTION('ref_axis',(0.,0.,1.));
#36738=DIRECTION('center_axis',(0.,0.,-1.));
#36739=DIRECTION('ref_axis',(0.,-1.,0.));
#36740=DIRECTION('',(0.,-1.,0.));
#36741=DIRECTION('',(-1.,0.,0.));
#36742=DIRECTION('',(0.,-1.,0.));
#36743=DIRECTION('',(-1.,0.,0.));
#36744=DIRECTION('center_axis',(0.,1.,0.));
#36745=DIRECTION('ref_axis',(0.,0.,-1.));
#36746=DIRECTION('',(0.,0.,-1.));
#36747=DIRECTION('',(-1.,0.,0.));
#36748=DIRECTION('',(0.,0.,-1.));
#36749=DIRECTION('center_axis',(0.,0.,1.));
#36750=DIRECTION('ref_axis',(0.,1.,0.));
#36751=DIRECTION('',(0.,1.,0.));
#36752=DIRECTION('',(-1.,0.,0.));
#36753=DIRECTION('',(0.,1.,0.));
#36754=DIRECTION('center_axis',(0.,-1.,0.));
#36755=DIRECTION('ref_axis',(0.,0.,1.));
#36756=DIRECTION('',(0.,0.,1.));
#36757=DIRECTION('',(0.,0.,1.));
#36758=DIRECTION('center_axis',(-1.,0.,0.));
#36759=DIRECTION('ref_axis',(0.,0.,1.));
#36760=DIRECTION('center_axis',(0.,0.,-1.));
#36761=DIRECTION('ref_axis',(0.,-1.,0.));
#36762=DIRECTION('',(0.,-1.,0.));
#36763=DIRECTION('',(-1.,0.,0.));
#36764=DIRECTION('',(0.,-1.,0.));
#36765=DIRECTION('',(-1.,0.,0.));
#36766=DIRECTION('center_axis',(0.,1.,0.));
#36767=DIRECTION('ref_axis',(0.,0.,-1.));
#36768=DIRECTION('',(0.,0.,-1.));
#36769=DIRECTION('',(-1.,0.,0.));
#36770=DIRECTION('',(0.,0.,-1.));
#36771=DIRECTION('center_axis',(0.,0.,1.));
#36772=DIRECTION('ref_axis',(0.,1.,0.));
#36773=DIRECTION('',(0.,1.,0.));
#36774=DIRECTION('',(-1.,0.,0.));
#36775=DIRECTION('',(0.,1.,0.));
#36776=DIRECTION('center_axis',(0.,-1.,0.));
#36777=DIRECTION('ref_axis',(0.,0.,1.));
#36778=DIRECTION('',(0.,0.,1.));
#36779=DIRECTION('',(0.,0.,1.));
#36780=DIRECTION('center_axis',(-1.,0.,0.));
#36781=DIRECTION('ref_axis',(0.,0.,1.));
#36782=DIRECTION('center_axis',(0.,0.,-1.));
#36783=DIRECTION('ref_axis',(0.,-1.,0.));
#36784=DIRECTION('',(0.,-1.,0.));
#36785=DIRECTION('',(-1.,0.,0.));
#36786=DIRECTION('',(0.,-1.,0.));
#36787=DIRECTION('',(-1.,0.,0.));
#36788=DIRECTION('center_axis',(0.,1.,0.));
#36789=DIRECTION('ref_axis',(0.,0.,-1.));
#36790=DIRECTION('',(0.,0.,-1.));
#36791=DIRECTION('',(-1.,0.,0.));
#36792=DIRECTION('',(0.,0.,-1.));
#36793=DIRECTION('center_axis',(0.,0.,1.));
#36794=DIRECTION('ref_axis',(0.,1.,0.));
#36795=DIRECTION('',(0.,1.,0.));
#36796=DIRECTION('',(-1.,0.,0.));
#36797=DIRECTION('',(0.,1.,0.));
#36798=DIRECTION('center_axis',(0.,-1.,0.));
#36799=DIRECTION('ref_axis',(0.,0.,1.));
#36800=DIRECTION('',(0.,0.,1.));
#36801=DIRECTION('',(0.,0.,1.));
#36802=DIRECTION('center_axis',(-1.,0.,0.));
#36803=DIRECTION('ref_axis',(0.,0.,1.));
#36804=DIRECTION('center_axis',(0.,0.,-1.));
#36805=DIRECTION('ref_axis',(0.,-1.,0.));
#36806=DIRECTION('',(0.,-1.,0.));
#36807=DIRECTION('',(-1.,0.,0.));
#36808=DIRECTION('',(0.,-1.,0.));
#36809=DIRECTION('',(-1.,0.,0.));
#36810=DIRECTION('center_axis',(0.,1.,0.));
#36811=DIRECTION('ref_axis',(0.,0.,-1.));
#36812=DIRECTION('',(0.,0.,-1.));
#36813=DIRECTION('',(-1.,0.,0.));
#36814=DIRECTION('',(0.,0.,-1.));
#36815=DIRECTION('center_axis',(0.,0.,1.));
#36816=DIRECTION('ref_axis',(0.,1.,0.));
#36817=DIRECTION('',(0.,1.,0.));
#36818=DIRECTION('',(-1.,0.,0.));
#36819=DIRECTION('',(0.,1.,0.));
#36820=DIRECTION('center_axis',(0.,-1.,0.));
#36821=DIRECTION('ref_axis',(0.,0.,1.));
#36822=DIRECTION('',(0.,0.,1.));
#36823=DIRECTION('',(0.,0.,1.));
#36824=DIRECTION('center_axis',(-1.,0.,0.));
#36825=DIRECTION('ref_axis',(0.,0.,1.));
#36826=DIRECTION('center_axis',(0.,0.,-1.));
#36827=DIRECTION('ref_axis',(0.,-1.,0.));
#36828=DIRECTION('',(0.,-1.,0.));
#36829=DIRECTION('',(-1.,0.,0.));
#36830=DIRECTION('',(0.,-1.,0.));
#36831=DIRECTION('',(-1.,0.,0.));
#36832=DIRECTION('center_axis',(0.,1.,0.));
#36833=DIRECTION('ref_axis',(0.,0.,-1.));
#36834=DIRECTION('',(0.,0.,-1.));
#36835=DIRECTION('',(-1.,0.,0.));
#36836=DIRECTION('',(0.,0.,-1.));
#36837=DIRECTION('center_axis',(0.,0.,1.));
#36838=DIRECTION('ref_axis',(0.,1.,0.));
#36839=DIRECTION('',(0.,1.,0.));
#36840=DIRECTION('',(-1.,0.,0.));
#36841=DIRECTION('',(0.,1.,0.));
#36842=DIRECTION('center_axis',(0.,-1.,0.));
#36843=DIRECTION('ref_axis',(0.,0.,1.));
#36844=DIRECTION('',(0.,0.,1.));
#36845=DIRECTION('',(0.,0.,1.));
#36846=DIRECTION('center_axis',(-1.,0.,0.));
#36847=DIRECTION('ref_axis',(0.,0.,1.));
#36848=DIRECTION('center_axis',(0.,0.,-1.));
#36849=DIRECTION('ref_axis',(0.,-1.,0.));
#36850=DIRECTION('',(0.,-1.,0.));
#36851=DIRECTION('',(-1.,0.,0.));
#36852=DIRECTION('',(0.,-1.,0.));
#36853=DIRECTION('',(-1.,0.,0.));
#36854=DIRECTION('center_axis',(0.,1.,0.));
#36855=DIRECTION('ref_axis',(0.,0.,-1.));
#36856=DIRECTION('',(0.,0.,-1.));
#36857=DIRECTION('',(-1.,0.,0.));
#36858=DIRECTION('',(0.,0.,-1.));
#36859=DIRECTION('center_axis',(0.,0.,1.));
#36860=DIRECTION('ref_axis',(0.,1.,0.));
#36861=DIRECTION('',(0.,1.,0.));
#36862=DIRECTION('',(-1.,0.,0.));
#36863=DIRECTION('',(0.,1.,0.));
#36864=DIRECTION('center_axis',(0.,-1.,0.));
#36865=DIRECTION('ref_axis',(0.,0.,1.));
#36866=DIRECTION('',(0.,0.,1.));
#36867=DIRECTION('',(0.,0.,1.));
#36868=DIRECTION('center_axis',(-1.,0.,0.));
#36869=DIRECTION('ref_axis',(0.,0.,1.));
#36870=DIRECTION('center_axis',(0.,0.,-1.));
#36871=DIRECTION('ref_axis',(0.,-1.,0.));
#36872=DIRECTION('',(0.,-1.,0.));
#36873=DIRECTION('',(-1.,0.,0.));
#36874=DIRECTION('',(0.,-1.,0.));
#36875=DIRECTION('',(-1.,0.,0.));
#36876=DIRECTION('center_axis',(0.,1.,0.));
#36877=DIRECTION('ref_axis',(0.,0.,-1.));
#36878=DIRECTION('',(0.,0.,-1.));
#36879=DIRECTION('',(-1.,0.,0.));
#36880=DIRECTION('',(0.,0.,-1.));
#36881=DIRECTION('center_axis',(0.,0.,1.));
#36882=DIRECTION('ref_axis',(0.,1.,0.));
#36883=DIRECTION('',(0.,1.,0.));
#36884=DIRECTION('',(-1.,0.,0.));
#36885=DIRECTION('',(0.,1.,0.));
#36886=DIRECTION('center_axis',(0.,-1.,0.));
#36887=DIRECTION('ref_axis',(0.,0.,1.));
#36888=DIRECTION('',(0.,0.,1.));
#36889=DIRECTION('',(0.,0.,1.));
#36890=DIRECTION('center_axis',(-1.,0.,0.));
#36891=DIRECTION('ref_axis',(0.,0.,1.));
#36892=DIRECTION('center_axis',(0.,0.,-1.));
#36893=DIRECTION('ref_axis',(0.,-1.,0.));
#36894=DIRECTION('',(0.,-1.,0.));
#36895=DIRECTION('',(-1.,0.,0.));
#36896=DIRECTION('',(0.,-1.,0.));
#36897=DIRECTION('',(-1.,0.,0.));
#36898=DIRECTION('center_axis',(0.,1.,0.));
#36899=DIRECTION('ref_axis',(0.,0.,-1.));
#36900=DIRECTION('',(0.,0.,-1.));
#36901=DIRECTION('',(-1.,0.,0.));
#36902=DIRECTION('',(0.,0.,-1.));
#36903=DIRECTION('center_axis',(0.,0.,1.));
#36904=DIRECTION('ref_axis',(0.,1.,0.));
#36905=DIRECTION('',(0.,1.,0.));
#36906=DIRECTION('',(-1.,0.,0.));
#36907=DIRECTION('',(0.,1.,0.));
#36908=DIRECTION('center_axis',(0.,-1.,0.));
#36909=DIRECTION('ref_axis',(0.,0.,1.));
#36910=DIRECTION('',(0.,0.,1.));
#36911=DIRECTION('',(0.,0.,1.));
#36912=DIRECTION('center_axis',(-1.,0.,0.));
#36913=DIRECTION('ref_axis',(0.,0.,1.));
#36914=DIRECTION('center_axis',(0.,0.,-1.));
#36915=DIRECTION('ref_axis',(0.,-1.,0.));
#36916=DIRECTION('',(0.,-1.,0.));
#36917=DIRECTION('',(-1.,0.,0.));
#36918=DIRECTION('',(0.,-1.,0.));
#36919=DIRECTION('',(-1.,0.,0.));
#36920=DIRECTION('center_axis',(0.,1.,0.));
#36921=DIRECTION('ref_axis',(0.,0.,-1.));
#36922=DIRECTION('',(0.,0.,-1.));
#36923=DIRECTION('',(-1.,0.,0.));
#36924=DIRECTION('',(0.,0.,-1.));
#36925=DIRECTION('center_axis',(0.,0.,1.));
#36926=DIRECTION('ref_axis',(0.,1.,0.));
#36927=DIRECTION('',(0.,1.,0.));
#36928=DIRECTION('',(-1.,0.,0.));
#36929=DIRECTION('',(0.,1.,0.));
#36930=DIRECTION('center_axis',(0.,-1.,0.));
#36931=DIRECTION('ref_axis',(0.,0.,1.));
#36932=DIRECTION('',(0.,0.,1.));
#36933=DIRECTION('',(0.,0.,1.));
#36934=DIRECTION('center_axis',(-1.,0.,0.));
#36935=DIRECTION('ref_axis',(0.,0.,1.));
#36936=DIRECTION('center_axis',(0.,0.,-1.));
#36937=DIRECTION('ref_axis',(0.,-1.,0.));
#36938=DIRECTION('',(0.,-1.,0.));
#36939=DIRECTION('',(-1.,0.,0.));
#36940=DIRECTION('',(0.,-1.,0.));
#36941=DIRECTION('',(-1.,0.,0.));
#36942=DIRECTION('center_axis',(0.,1.,0.));
#36943=DIRECTION('ref_axis',(0.,0.,-1.));
#36944=DIRECTION('',(0.,0.,-1.));
#36945=DIRECTION('',(-1.,0.,0.));
#36946=DIRECTION('',(0.,0.,-1.));
#36947=DIRECTION('center_axis',(0.,0.,1.));
#36948=DIRECTION('ref_axis',(0.,1.,0.));
#36949=DIRECTION('',(0.,1.,0.));
#36950=DIRECTION('',(-1.,0.,0.));
#36951=DIRECTION('',(0.,1.,0.));
#36952=DIRECTION('center_axis',(0.,-1.,0.));
#36953=DIRECTION('ref_axis',(0.,0.,1.));
#36954=DIRECTION('',(0.,0.,1.));
#36955=DIRECTION('',(0.,0.,1.));
#36956=DIRECTION('center_axis',(-1.,0.,0.));
#36957=DIRECTION('ref_axis',(0.,0.,1.));
#36958=DIRECTION('center_axis',(0.,0.,-1.));
#36959=DIRECTION('ref_axis',(0.,-1.,0.));
#36960=DIRECTION('',(0.,-1.,0.));
#36961=DIRECTION('',(-1.,0.,0.));
#36962=DIRECTION('',(0.,-1.,0.));
#36963=DIRECTION('',(-1.,0.,0.));
#36964=DIRECTION('center_axis',(0.,1.,0.));
#36965=DIRECTION('ref_axis',(0.,0.,-1.));
#36966=DIRECTION('',(0.,0.,-1.));
#36967=DIRECTION('',(-1.,0.,0.));
#36968=DIRECTION('',(0.,0.,-1.));
#36969=DIRECTION('center_axis',(0.,0.,1.));
#36970=DIRECTION('ref_axis',(0.,1.,0.));
#36971=DIRECTION('',(0.,1.,0.));
#36972=DIRECTION('',(-1.,0.,0.));
#36973=DIRECTION('',(0.,1.,0.));
#36974=DIRECTION('center_axis',(0.,-1.,0.));
#36975=DIRECTION('ref_axis',(0.,0.,1.));
#36976=DIRECTION('',(0.,0.,1.));
#36977=DIRECTION('',(0.,0.,1.));
#36978=DIRECTION('center_axis',(-1.,0.,0.));
#36979=DIRECTION('ref_axis',(0.,0.,1.));
#36980=DIRECTION('center_axis',(0.,0.,-1.));
#36981=DIRECTION('ref_axis',(0.,-1.,0.));
#36982=DIRECTION('',(0.,-1.,0.));
#36983=DIRECTION('',(-1.,0.,0.));
#36984=DIRECTION('',(0.,-1.,0.));
#36985=DIRECTION('',(-1.,0.,0.));
#36986=DIRECTION('center_axis',(0.,1.,0.));
#36987=DIRECTION('ref_axis',(0.,0.,-1.));
#36988=DIRECTION('',(0.,0.,-1.));
#36989=DIRECTION('',(-1.,0.,0.));
#36990=DIRECTION('',(0.,0.,-1.));
#36991=DIRECTION('center_axis',(0.,0.,1.));
#36992=DIRECTION('ref_axis',(0.,1.,0.));
#36993=DIRECTION('',(0.,1.,0.));
#36994=DIRECTION('',(-1.,0.,0.));
#36995=DIRECTION('',(0.,1.,0.));
#36996=DIRECTION('center_axis',(0.,-1.,0.));
#36997=DIRECTION('ref_axis',(0.,0.,1.));
#36998=DIRECTION('',(0.,0.,1.));
#36999=DIRECTION('',(0.,0.,1.));
#37000=DIRECTION('center_axis',(-1.,0.,0.));
#37001=DIRECTION('ref_axis',(0.,0.,1.));
#37002=DIRECTION('center_axis',(0.,0.,-1.));
#37003=DIRECTION('ref_axis',(0.,-1.,0.));
#37004=DIRECTION('',(0.,-1.,0.));
#37005=DIRECTION('',(-1.,0.,0.));
#37006=DIRECTION('',(0.,-1.,0.));
#37007=DIRECTION('',(-1.,0.,0.));
#37008=DIRECTION('center_axis',(0.,1.,0.));
#37009=DIRECTION('ref_axis',(0.,0.,-1.));
#37010=DIRECTION('',(0.,0.,-1.));
#37011=DIRECTION('',(-1.,0.,0.));
#37012=DIRECTION('',(0.,0.,-1.));
#37013=DIRECTION('center_axis',(0.,0.,1.));
#37014=DIRECTION('ref_axis',(0.,1.,0.));
#37015=DIRECTION('',(0.,1.,0.));
#37016=DIRECTION('',(-1.,0.,0.));
#37017=DIRECTION('',(0.,1.,0.));
#37018=DIRECTION('center_axis',(0.,-1.,0.));
#37019=DIRECTION('ref_axis',(0.,0.,1.));
#37020=DIRECTION('',(0.,0.,1.));
#37021=DIRECTION('',(0.,0.,1.));
#37022=DIRECTION('center_axis',(-1.,0.,0.));
#37023=DIRECTION('ref_axis',(0.,0.,1.));
#37024=DIRECTION('center_axis',(0.,0.,-1.));
#37025=DIRECTION('ref_axis',(0.,-1.,0.));
#37026=DIRECTION('',(0.,-1.,0.));
#37027=DIRECTION('',(-1.,0.,0.));
#37028=DIRECTION('',(0.,-1.,0.));
#37029=DIRECTION('',(-1.,0.,0.));
#37030=DIRECTION('center_axis',(0.,1.,0.));
#37031=DIRECTION('ref_axis',(0.,0.,-1.));
#37032=DIRECTION('',(0.,0.,-1.));
#37033=DIRECTION('',(-1.,0.,0.));
#37034=DIRECTION('',(0.,0.,-1.));
#37035=DIRECTION('center_axis',(0.,0.,1.));
#37036=DIRECTION('ref_axis',(0.,1.,0.));
#37037=DIRECTION('',(0.,1.,0.));
#37038=DIRECTION('',(-1.,0.,0.));
#37039=DIRECTION('',(0.,1.,0.));
#37040=DIRECTION('center_axis',(0.,-1.,0.));
#37041=DIRECTION('ref_axis',(0.,0.,1.));
#37042=DIRECTION('',(0.,0.,1.));
#37043=DIRECTION('',(0.,0.,1.));
#37044=DIRECTION('center_axis',(-1.,0.,0.));
#37045=DIRECTION('ref_axis',(0.,0.,1.));
#37046=DIRECTION('center_axis',(0.,0.,-1.));
#37047=DIRECTION('ref_axis',(0.,-1.,0.));
#37048=DIRECTION('',(0.,-1.,0.));
#37049=DIRECTION('',(-1.,0.,0.));
#37050=DIRECTION('',(0.,-1.,0.));
#37051=DIRECTION('',(-1.,0.,0.));
#37052=DIRECTION('center_axis',(0.,1.,0.));
#37053=DIRECTION('ref_axis',(0.,0.,-1.));
#37054=DIRECTION('',(0.,0.,-1.));
#37055=DIRECTION('',(-1.,0.,0.));
#37056=DIRECTION('',(0.,0.,-1.));
#37057=DIRECTION('center_axis',(0.,0.,1.));
#37058=DIRECTION('ref_axis',(0.,1.,0.));
#37059=DIRECTION('',(0.,1.,0.));
#37060=DIRECTION('',(-1.,0.,0.));
#37061=DIRECTION('',(0.,1.,0.));
#37062=DIRECTION('center_axis',(0.,-1.,0.));
#37063=DIRECTION('ref_axis',(0.,0.,1.));
#37064=DIRECTION('',(0.,0.,1.));
#37065=DIRECTION('',(0.,0.,1.));
#37066=DIRECTION('center_axis',(-1.,0.,0.));
#37067=DIRECTION('ref_axis',(0.,0.,1.));
#37068=DIRECTION('center_axis',(0.,0.,-1.));
#37069=DIRECTION('ref_axis',(0.,-1.,0.));
#37070=DIRECTION('',(0.,-1.,0.));
#37071=DIRECTION('',(-1.,0.,0.));
#37072=DIRECTION('',(0.,-1.,0.));
#37073=DIRECTION('',(-1.,0.,0.));
#37074=DIRECTION('center_axis',(0.,1.,0.));
#37075=DIRECTION('ref_axis',(0.,0.,-1.));
#37076=DIRECTION('',(0.,0.,-1.));
#37077=DIRECTION('',(-1.,0.,0.));
#37078=DIRECTION('',(0.,0.,-1.));
#37079=DIRECTION('center_axis',(0.,0.,1.));
#37080=DIRECTION('ref_axis',(0.,1.,0.));
#37081=DIRECTION('',(0.,1.,0.));
#37082=DIRECTION('',(-1.,0.,0.));
#37083=DIRECTION('',(0.,1.,0.));
#37084=DIRECTION('center_axis',(0.,-1.,0.));
#37085=DIRECTION('ref_axis',(0.,0.,1.));
#37086=DIRECTION('',(0.,0.,1.));
#37087=DIRECTION('',(0.,0.,1.));
#37088=DIRECTION('center_axis',(-1.,0.,0.));
#37089=DIRECTION('ref_axis',(0.,0.,1.));
#37090=DIRECTION('center_axis',(0.,0.,-1.));
#37091=DIRECTION('ref_axis',(0.,-1.,0.));
#37092=DIRECTION('',(0.,-1.,0.));
#37093=DIRECTION('',(-1.,0.,0.));
#37094=DIRECTION('',(0.,-1.,0.));
#37095=DIRECTION('',(-1.,0.,0.));
#37096=DIRECTION('center_axis',(0.,1.,0.));
#37097=DIRECTION('ref_axis',(0.,0.,-1.));
#37098=DIRECTION('',(0.,0.,-1.));
#37099=DIRECTION('',(-1.,0.,0.));
#37100=DIRECTION('',(0.,0.,-1.));
#37101=DIRECTION('center_axis',(0.,0.,1.));
#37102=DIRECTION('ref_axis',(0.,1.,0.));
#37103=DIRECTION('',(0.,1.,0.));
#37104=DIRECTION('',(-1.,0.,0.));
#37105=DIRECTION('',(0.,1.,0.));
#37106=DIRECTION('center_axis',(0.,-1.,0.));
#37107=DIRECTION('ref_axis',(0.,0.,1.));
#37108=DIRECTION('',(0.,0.,1.));
#37109=DIRECTION('',(0.,0.,1.));
#37110=DIRECTION('center_axis',(-1.,0.,0.));
#37111=DIRECTION('ref_axis',(0.,0.,1.));
#37112=DIRECTION('center_axis',(0.,0.,-1.));
#37113=DIRECTION('ref_axis',(0.,-1.,0.));
#37114=DIRECTION('',(0.,-1.,0.));
#37115=DIRECTION('',(-1.,0.,0.));
#37116=DIRECTION('',(0.,-1.,0.));
#37117=DIRECTION('',(-1.,0.,0.));
#37118=DIRECTION('center_axis',(0.,1.,0.));
#37119=DIRECTION('ref_axis',(0.,0.,-1.));
#37120=DIRECTION('',(0.,0.,-1.));
#37121=DIRECTION('',(-1.,0.,0.));
#37122=DIRECTION('',(0.,0.,-1.));
#37123=DIRECTION('center_axis',(0.,0.,1.));
#37124=DIRECTION('ref_axis',(0.,1.,0.));
#37125=DIRECTION('',(0.,1.,0.));
#37126=DIRECTION('',(-1.,0.,0.));
#37127=DIRECTION('',(0.,1.,0.));
#37128=DIRECTION('center_axis',(0.,-1.,0.));
#37129=DIRECTION('ref_axis',(0.,0.,1.));
#37130=DIRECTION('',(0.,0.,1.));
#37131=DIRECTION('',(0.,0.,1.));
#37132=DIRECTION('center_axis',(-1.,0.,0.));
#37133=DIRECTION('ref_axis',(0.,0.,1.));
#37134=DIRECTION('center_axis',(0.,0.,-1.));
#37135=DIRECTION('ref_axis',(0.,-1.,0.));
#37136=DIRECTION('',(0.,-1.,0.));
#37137=DIRECTION('',(-1.,0.,0.));
#37138=DIRECTION('',(0.,-1.,0.));
#37139=DIRECTION('',(-1.,0.,0.));
#37140=DIRECTION('center_axis',(0.,1.,0.));
#37141=DIRECTION('ref_axis',(0.,0.,-1.));
#37142=DIRECTION('',(0.,0.,-1.));
#37143=DIRECTION('',(-1.,0.,0.));
#37144=DIRECTION('',(0.,0.,-1.));
#37145=DIRECTION('center_axis',(0.,0.,1.));
#37146=DIRECTION('ref_axis',(0.,1.,0.));
#37147=DIRECTION('',(0.,1.,0.));
#37148=DIRECTION('',(-1.,0.,0.));
#37149=DIRECTION('',(0.,1.,0.));
#37150=DIRECTION('center_axis',(0.,-1.,0.));
#37151=DIRECTION('ref_axis',(0.,0.,1.));
#37152=DIRECTION('',(0.,0.,1.));
#37153=DIRECTION('',(0.,0.,1.));
#37154=DIRECTION('center_axis',(-1.,0.,0.));
#37155=DIRECTION('ref_axis',(0.,0.,1.));
#37156=DIRECTION('center_axis',(0.,0.,-1.));
#37157=DIRECTION('ref_axis',(0.,-1.,0.));
#37158=DIRECTION('',(0.,-1.,0.));
#37159=DIRECTION('',(-1.,0.,0.));
#37160=DIRECTION('',(0.,-1.,0.));
#37161=DIRECTION('',(-1.,0.,0.));
#37162=DIRECTION('center_axis',(0.,1.,0.));
#37163=DIRECTION('ref_axis',(0.,0.,-1.));
#37164=DIRECTION('',(0.,0.,-1.));
#37165=DIRECTION('',(-1.,0.,0.));
#37166=DIRECTION('',(0.,0.,-1.));
#37167=DIRECTION('center_axis',(0.,0.,1.));
#37168=DIRECTION('ref_axis',(0.,1.,0.));
#37169=DIRECTION('',(0.,1.,0.));
#37170=DIRECTION('',(-1.,0.,0.));
#37171=DIRECTION('',(0.,1.,0.));
#37172=DIRECTION('center_axis',(0.,-1.,0.));
#37173=DIRECTION('ref_axis',(0.,0.,1.));
#37174=DIRECTION('',(0.,0.,1.));
#37175=DIRECTION('',(0.,0.,1.));
#37176=DIRECTION('center_axis',(-1.,0.,0.));
#37177=DIRECTION('ref_axis',(0.,0.,1.));
#37178=DIRECTION('center_axis',(0.,0.,-1.));
#37179=DIRECTION('ref_axis',(0.,-1.,0.));
#37180=DIRECTION('',(0.,-1.,0.));
#37181=DIRECTION('',(-1.,0.,0.));
#37182=DIRECTION('',(0.,-1.,0.));
#37183=DIRECTION('',(-1.,0.,0.));
#37184=DIRECTION('center_axis',(0.,1.,0.));
#37185=DIRECTION('ref_axis',(0.,0.,-1.));
#37186=DIRECTION('',(0.,0.,-1.));
#37187=DIRECTION('',(-1.,0.,0.));
#37188=DIRECTION('',(0.,0.,-1.));
#37189=DIRECTION('center_axis',(0.,0.,1.));
#37190=DIRECTION('ref_axis',(0.,1.,0.));
#37191=DIRECTION('',(0.,1.,0.));
#37192=DIRECTION('',(-1.,0.,0.));
#37193=DIRECTION('',(0.,1.,0.));
#37194=DIRECTION('center_axis',(0.,-1.,0.));
#37195=DIRECTION('ref_axis',(0.,0.,1.));
#37196=DIRECTION('',(0.,0.,1.));
#37197=DIRECTION('',(0.,0.,1.));
#37198=DIRECTION('center_axis',(-1.,0.,0.));
#37199=DIRECTION('ref_axis',(0.,0.,1.));
#37200=DIRECTION('center_axis',(0.,0.,-1.));
#37201=DIRECTION('ref_axis',(0.,-1.,0.));
#37202=DIRECTION('',(0.,-1.,0.));
#37203=DIRECTION('',(-1.,0.,0.));
#37204=DIRECTION('',(0.,-1.,0.));
#37205=DIRECTION('',(-1.,0.,0.));
#37206=DIRECTION('center_axis',(0.,1.,0.));
#37207=DIRECTION('ref_axis',(0.,0.,-1.));
#37208=DIRECTION('',(0.,0.,-1.));
#37209=DIRECTION('',(-1.,0.,0.));
#37210=DIRECTION('',(0.,0.,-1.));
#37211=DIRECTION('center_axis',(0.,0.,1.));
#37212=DIRECTION('ref_axis',(0.,1.,0.));
#37213=DIRECTION('',(0.,1.,0.));
#37214=DIRECTION('',(-1.,0.,0.));
#37215=DIRECTION('',(0.,1.,0.));
#37216=DIRECTION('center_axis',(0.,-1.,0.));
#37217=DIRECTION('ref_axis',(0.,0.,1.));
#37218=DIRECTION('',(0.,0.,1.));
#37219=DIRECTION('',(0.,0.,1.));
#37220=DIRECTION('center_axis',(-1.,0.,0.));
#37221=DIRECTION('ref_axis',(0.,0.,1.));
#37222=DIRECTION('center_axis',(0.,0.,-1.));
#37223=DIRECTION('ref_axis',(0.,-1.,0.));
#37224=DIRECTION('',(0.,-1.,0.));
#37225=DIRECTION('',(-1.,0.,0.));
#37226=DIRECTION('',(0.,-1.,0.));
#37227=DIRECTION('',(-1.,0.,0.));
#37228=DIRECTION('center_axis',(0.,1.,0.));
#37229=DIRECTION('ref_axis',(0.,0.,-1.));
#37230=DIRECTION('',(0.,0.,-1.));
#37231=DIRECTION('',(-1.,0.,0.));
#37232=DIRECTION('',(0.,0.,-1.));
#37233=DIRECTION('center_axis',(0.,0.,1.));
#37234=DIRECTION('ref_axis',(0.,1.,0.));
#37235=DIRECTION('',(0.,1.,0.));
#37236=DIRECTION('',(-1.,0.,0.));
#37237=DIRECTION('',(0.,1.,0.));
#37238=DIRECTION('center_axis',(0.,-1.,0.));
#37239=DIRECTION('ref_axis',(0.,0.,1.));
#37240=DIRECTION('',(0.,0.,1.));
#37241=DIRECTION('',(0.,0.,1.));
#37242=DIRECTION('center_axis',(-1.,0.,0.));
#37243=DIRECTION('ref_axis',(0.,0.,1.));
#37244=DIRECTION('center_axis',(0.,0.,-1.));
#37245=DIRECTION('ref_axis',(0.,-1.,0.));
#37246=DIRECTION('',(0.,-1.,0.));
#37247=DIRECTION('',(-1.,0.,0.));
#37248=DIRECTION('',(0.,-1.,0.));
#37249=DIRECTION('',(-1.,0.,0.));
#37250=DIRECTION('center_axis',(0.,1.,0.));
#37251=DIRECTION('ref_axis',(0.,0.,-1.));
#37252=DIRECTION('',(0.,0.,-1.));
#37253=DIRECTION('',(-1.,0.,0.));
#37254=DIRECTION('',(0.,0.,-1.));
#37255=DIRECTION('center_axis',(0.,0.,1.));
#37256=DIRECTION('ref_axis',(0.,1.,0.));
#37257=DIRECTION('',(0.,1.,0.));
#37258=DIRECTION('',(-1.,0.,0.));
#37259=DIRECTION('',(0.,1.,0.));
#37260=DIRECTION('center_axis',(0.,-1.,0.));
#37261=DIRECTION('ref_axis',(0.,0.,1.));
#37262=DIRECTION('',(0.,0.,1.));
#37263=DIRECTION('',(0.,0.,1.));
#37264=DIRECTION('center_axis',(-1.,0.,0.));
#37265=DIRECTION('ref_axis',(0.,0.,1.));
#37266=DIRECTION('center_axis',(0.,0.,-1.));
#37267=DIRECTION('ref_axis',(0.,-1.,0.));
#37268=DIRECTION('',(0.,-1.,0.));
#37269=DIRECTION('',(-1.,0.,0.));
#37270=DIRECTION('',(0.,-1.,0.));
#37271=DIRECTION('',(-1.,0.,0.));
#37272=DIRECTION('center_axis',(0.,1.,0.));
#37273=DIRECTION('ref_axis',(0.,0.,-1.));
#37274=DIRECTION('',(0.,0.,-1.));
#37275=DIRECTION('',(-1.,0.,0.));
#37276=DIRECTION('',(0.,0.,-1.));
#37277=DIRECTION('center_axis',(0.,0.,1.));
#37278=DIRECTION('ref_axis',(0.,1.,0.));
#37279=DIRECTION('',(0.,1.,0.));
#37280=DIRECTION('',(-1.,0.,0.));
#37281=DIRECTION('',(0.,1.,0.));
#37282=DIRECTION('center_axis',(0.,-1.,0.));
#37283=DIRECTION('ref_axis',(0.,0.,1.));
#37284=DIRECTION('',(0.,0.,1.));
#37285=DIRECTION('',(0.,0.,1.));
#37286=DIRECTION('center_axis',(-1.,0.,0.));
#37287=DIRECTION('ref_axis',(0.,0.,1.));
#37288=DIRECTION('center_axis',(0.,0.,-1.));
#37289=DIRECTION('ref_axis',(0.,-1.,0.));
#37290=DIRECTION('',(0.,-1.,0.));
#37291=DIRECTION('',(-1.,0.,0.));
#37292=DIRECTION('',(0.,-1.,0.));
#37293=DIRECTION('',(-1.,0.,0.));
#37294=DIRECTION('center_axis',(0.,1.,0.));
#37295=DIRECTION('ref_axis',(0.,0.,-1.));
#37296=DIRECTION('',(0.,0.,-1.));
#37297=DIRECTION('',(-1.,0.,0.));
#37298=DIRECTION('',(0.,0.,-1.));
#37299=DIRECTION('center_axis',(0.,0.,1.));
#37300=DIRECTION('ref_axis',(0.,1.,0.));
#37301=DIRECTION('',(0.,1.,0.));
#37302=DIRECTION('',(-1.,0.,0.));
#37303=DIRECTION('',(0.,1.,0.));
#37304=DIRECTION('center_axis',(0.,-1.,0.));
#37305=DIRECTION('ref_axis',(0.,0.,1.));
#37306=DIRECTION('',(0.,0.,1.));
#37307=DIRECTION('',(0.,0.,1.));
#37308=DIRECTION('center_axis',(-1.,0.,0.));
#37309=DIRECTION('ref_axis',(0.,0.,1.));
#37310=DIRECTION('center_axis',(0.,0.,-1.));
#37311=DIRECTION('ref_axis',(0.,-1.,0.));
#37312=DIRECTION('',(0.,-1.,0.));
#37313=DIRECTION('',(-1.,0.,0.));
#37314=DIRECTION('',(0.,-1.,0.));
#37315=DIRECTION('',(-1.,0.,0.));
#37316=DIRECTION('center_axis',(0.,1.,0.));
#37317=DIRECTION('ref_axis',(0.,0.,-1.));
#37318=DIRECTION('',(0.,0.,-1.));
#37319=DIRECTION('',(-1.,0.,0.));
#37320=DIRECTION('',(0.,0.,-1.));
#37321=DIRECTION('center_axis',(0.,0.,1.));
#37322=DIRECTION('ref_axis',(0.,1.,0.));
#37323=DIRECTION('',(0.,1.,0.));
#37324=DIRECTION('',(-1.,0.,0.));
#37325=DIRECTION('',(0.,1.,0.));
#37326=DIRECTION('center_axis',(0.,-1.,0.));
#37327=DIRECTION('ref_axis',(0.,0.,1.));
#37328=DIRECTION('',(0.,0.,1.));
#37329=DIRECTION('',(0.,0.,1.));
#37330=DIRECTION('center_axis',(-1.,0.,0.));
#37331=DIRECTION('ref_axis',(0.,0.,1.));
#37332=DIRECTION('center_axis',(0.,0.,-1.));
#37333=DIRECTION('ref_axis',(0.,-1.,0.));
#37334=DIRECTION('',(0.,-1.,0.));
#37335=DIRECTION('',(-1.,0.,0.));
#37336=DIRECTION('',(0.,-1.,0.));
#37337=DIRECTION('',(-1.,0.,0.));
#37338=DIRECTION('center_axis',(0.,1.,0.));
#37339=DIRECTION('ref_axis',(0.,0.,-1.));
#37340=DIRECTION('',(0.,0.,-1.));
#37341=DIRECTION('',(-1.,0.,0.));
#37342=DIRECTION('',(0.,0.,-1.));
#37343=DIRECTION('center_axis',(0.,0.,1.));
#37344=DIRECTION('ref_axis',(0.,1.,0.));
#37345=DIRECTION('',(0.,1.,0.));
#37346=DIRECTION('',(-1.,0.,0.));
#37347=DIRECTION('',(0.,1.,0.));
#37348=DIRECTION('center_axis',(0.,-1.,0.));
#37349=DIRECTION('ref_axis',(0.,0.,1.));
#37350=DIRECTION('',(0.,0.,1.));
#37351=DIRECTION('',(0.,0.,1.));
#37352=DIRECTION('center_axis',(-1.,0.,0.));
#37353=DIRECTION('ref_axis',(0.,0.,1.));
#37354=DIRECTION('center_axis',(0.,0.,-1.));
#37355=DIRECTION('ref_axis',(0.,-1.,0.));
#37356=DIRECTION('',(0.,-1.,0.));
#37357=DIRECTION('',(-1.,0.,0.));
#37358=DIRECTION('',(0.,-1.,0.));
#37359=DIRECTION('',(-1.,0.,0.));
#37360=DIRECTION('center_axis',(0.,1.,0.));
#37361=DIRECTION('ref_axis',(0.,0.,-1.));
#37362=DIRECTION('',(0.,0.,-1.));
#37363=DIRECTION('',(-1.,0.,0.));
#37364=DIRECTION('',(0.,0.,-1.));
#37365=DIRECTION('center_axis',(0.,0.,1.));
#37366=DIRECTION('ref_axis',(0.,1.,0.));
#37367=DIRECTION('',(0.,1.,0.));
#37368=DIRECTION('',(-1.,0.,0.));
#37369=DIRECTION('',(0.,1.,0.));
#37370=DIRECTION('center_axis',(0.,-1.,0.));
#37371=DIRECTION('ref_axis',(0.,0.,1.));
#37372=DIRECTION('',(0.,0.,1.));
#37373=DIRECTION('',(0.,0.,1.));
#37374=DIRECTION('center_axis',(-1.,0.,0.));
#37375=DIRECTION('ref_axis',(0.,0.,1.));
#37376=DIRECTION('center_axis',(0.,0.,-1.));
#37377=DIRECTION('ref_axis',(0.,-1.,0.));
#37378=DIRECTION('',(0.,-1.,0.));
#37379=DIRECTION('',(-1.,0.,0.));
#37380=DIRECTION('',(0.,-1.,0.));
#37381=DIRECTION('',(-1.,0.,0.));
#37382=DIRECTION('center_axis',(0.,1.,0.));
#37383=DIRECTION('ref_axis',(0.,0.,-1.));
#37384=DIRECTION('',(0.,0.,-1.));
#37385=DIRECTION('',(-1.,0.,0.));
#37386=DIRECTION('',(0.,0.,-1.));
#37387=DIRECTION('center_axis',(0.,0.,1.));
#37388=DIRECTION('ref_axis',(0.,1.,0.));
#37389=DIRECTION('',(0.,1.,0.));
#37390=DIRECTION('',(-1.,0.,0.));
#37391=DIRECTION('',(0.,1.,0.));
#37392=DIRECTION('center_axis',(0.,-1.,0.));
#37393=DIRECTION('ref_axis',(0.,0.,1.));
#37394=DIRECTION('',(0.,0.,1.));
#37395=DIRECTION('',(0.,0.,1.));
#37396=DIRECTION('center_axis',(-1.,0.,0.));
#37397=DIRECTION('ref_axis',(0.,0.,1.));
#37398=DIRECTION('center_axis',(0.,0.,-1.));
#37399=DIRECTION('ref_axis',(0.,-1.,0.));
#37400=DIRECTION('',(0.,-1.,0.));
#37401=DIRECTION('',(-1.,0.,0.));
#37402=DIRECTION('',(0.,-1.,0.));
#37403=DIRECTION('',(-1.,0.,0.));
#37404=DIRECTION('center_axis',(0.,1.,0.));
#37405=DIRECTION('ref_axis',(0.,0.,-1.));
#37406=DIRECTION('',(0.,0.,-1.));
#37407=DIRECTION('',(-1.,0.,0.));
#37408=DIRECTION('',(0.,0.,-1.));
#37409=DIRECTION('center_axis',(0.,0.,1.));
#37410=DIRECTION('ref_axis',(0.,1.,0.));
#37411=DIRECTION('',(0.,1.,0.));
#37412=DIRECTION('',(-1.,0.,0.));
#37413=DIRECTION('',(0.,1.,0.));
#37414=DIRECTION('center_axis',(0.,-1.,0.));
#37415=DIRECTION('ref_axis',(0.,0.,1.));
#37416=DIRECTION('',(0.,0.,1.));
#37417=DIRECTION('',(0.,0.,1.));
#37418=DIRECTION('center_axis',(-1.,0.,0.));
#37419=DIRECTION('ref_axis',(0.,0.,1.));
#37420=DIRECTION('center_axis',(0.,0.,-1.));
#37421=DIRECTION('ref_axis',(0.,-1.,0.));
#37422=DIRECTION('',(0.,-1.,0.));
#37423=DIRECTION('',(-1.,0.,0.));
#37424=DIRECTION('',(0.,-1.,0.));
#37425=DIRECTION('',(-1.,0.,0.));
#37426=DIRECTION('center_axis',(0.,1.,0.));
#37427=DIRECTION('ref_axis',(0.,0.,-1.));
#37428=DIRECTION('',(0.,0.,-1.));
#37429=DIRECTION('',(-1.,0.,0.));
#37430=DIRECTION('',(0.,0.,-1.));
#37431=DIRECTION('center_axis',(0.,0.,1.));
#37432=DIRECTION('ref_axis',(0.,1.,0.));
#37433=DIRECTION('',(0.,1.,0.));
#37434=DIRECTION('',(-1.,0.,0.));
#37435=DIRECTION('',(0.,1.,0.));
#37436=DIRECTION('center_axis',(0.,-1.,0.));
#37437=DIRECTION('ref_axis',(0.,0.,1.));
#37438=DIRECTION('',(0.,0.,1.));
#37439=DIRECTION('',(0.,0.,1.));
#37440=DIRECTION('center_axis',(-1.,0.,0.));
#37441=DIRECTION('ref_axis',(0.,0.,1.));
#37442=DIRECTION('center_axis',(0.,0.,-1.));
#37443=DIRECTION('ref_axis',(0.,-1.,0.));
#37444=DIRECTION('',(0.,-1.,0.));
#37445=DIRECTION('',(-1.,0.,0.));
#37446=DIRECTION('',(0.,-1.,0.));
#37447=DIRECTION('',(-1.,0.,0.));
#37448=DIRECTION('center_axis',(0.,1.,0.));
#37449=DIRECTION('ref_axis',(0.,0.,-1.));
#37450=DIRECTION('',(0.,0.,-1.));
#37451=DIRECTION('',(-1.,0.,0.));
#37452=DIRECTION('',(0.,0.,-1.));
#37453=DIRECTION('center_axis',(0.,0.,1.));
#37454=DIRECTION('ref_axis',(0.,1.,0.));
#37455=DIRECTION('',(0.,1.,0.));
#37456=DIRECTION('',(-1.,0.,0.));
#37457=DIRECTION('',(0.,1.,0.));
#37458=DIRECTION('center_axis',(0.,-1.,0.));
#37459=DIRECTION('ref_axis',(0.,0.,1.));
#37460=DIRECTION('',(0.,0.,1.));
#37461=DIRECTION('',(0.,0.,1.));
#37462=DIRECTION('center_axis',(-1.,0.,0.));
#37463=DIRECTION('ref_axis',(0.,0.,1.));
#37464=DIRECTION('center_axis',(0.,0.,-1.));
#37465=DIRECTION('ref_axis',(0.,-1.,0.));
#37466=DIRECTION('',(0.,-1.,0.));
#37467=DIRECTION('',(-1.,0.,0.));
#37468=DIRECTION('',(0.,-1.,0.));
#37469=DIRECTION('',(-1.,0.,0.));
#37470=DIRECTION('center_axis',(0.,1.,0.));
#37471=DIRECTION('ref_axis',(0.,0.,-1.));
#37472=DIRECTION('',(0.,0.,-1.));
#37473=DIRECTION('',(-1.,0.,0.));
#37474=DIRECTION('',(0.,0.,-1.));
#37475=DIRECTION('center_axis',(0.,0.,1.));
#37476=DIRECTION('ref_axis',(0.,1.,0.));
#37477=DIRECTION('',(0.,1.,0.));
#37478=DIRECTION('',(-1.,0.,0.));
#37479=DIRECTION('',(0.,1.,0.));
#37480=DIRECTION('center_axis',(0.,-1.,0.));
#37481=DIRECTION('ref_axis',(0.,0.,1.));
#37482=DIRECTION('',(0.,0.,1.));
#37483=DIRECTION('',(0.,0.,1.));
#37484=DIRECTION('center_axis',(-1.,0.,0.));
#37485=DIRECTION('ref_axis',(0.,0.,1.));
#37486=DIRECTION('center_axis',(0.,0.,-1.));
#37487=DIRECTION('ref_axis',(0.,-1.,0.));
#37488=DIRECTION('',(0.,-1.,0.));
#37489=DIRECTION('',(-1.,0.,0.));
#37490=DIRECTION('',(0.,-1.,0.));
#37491=DIRECTION('',(-1.,0.,0.));
#37492=DIRECTION('center_axis',(0.,1.,0.));
#37493=DIRECTION('ref_axis',(0.,0.,-1.));
#37494=DIRECTION('',(0.,0.,-1.));
#37495=DIRECTION('',(-1.,0.,0.));
#37496=DIRECTION('',(0.,0.,-1.));
#37497=DIRECTION('center_axis',(0.,0.,1.));
#37498=DIRECTION('ref_axis',(0.,1.,0.));
#37499=DIRECTION('',(0.,1.,0.));
#37500=DIRECTION('',(-1.,0.,0.));
#37501=DIRECTION('',(0.,1.,0.));
#37502=DIRECTION('center_axis',(0.,-1.,0.));
#37503=DIRECTION('ref_axis',(0.,0.,1.));
#37504=DIRECTION('',(0.,0.,1.));
#37505=DIRECTION('',(0.,0.,1.));
#37506=DIRECTION('center_axis',(-1.,0.,0.));
#37507=DIRECTION('ref_axis',(0.,0.,1.));
#37508=DIRECTION('center_axis',(0.,0.,-1.));
#37509=DIRECTION('ref_axis',(0.,-1.,0.));
#37510=DIRECTION('',(0.,-1.,0.));
#37511=DIRECTION('',(-1.,0.,0.));
#37512=DIRECTION('',(0.,-1.,0.));
#37513=DIRECTION('',(-1.,0.,0.));
#37514=DIRECTION('center_axis',(0.,1.,0.));
#37515=DIRECTION('ref_axis',(0.,0.,-1.));
#37516=DIRECTION('',(0.,0.,-1.));
#37517=DIRECTION('',(-1.,0.,0.));
#37518=DIRECTION('',(0.,0.,-1.));
#37519=DIRECTION('center_axis',(0.,0.,1.));
#37520=DIRECTION('ref_axis',(0.,1.,0.));
#37521=DIRECTION('',(0.,1.,0.));
#37522=DIRECTION('',(-1.,0.,0.));
#37523=DIRECTION('',(0.,1.,0.));
#37524=DIRECTION('center_axis',(0.,-1.,0.));
#37525=DIRECTION('ref_axis',(0.,0.,1.));
#37526=DIRECTION('',(0.,0.,1.));
#37527=DIRECTION('',(0.,0.,1.));
#37528=DIRECTION('center_axis',(-1.,0.,0.));
#37529=DIRECTION('ref_axis',(0.,0.,1.));
#37530=DIRECTION('center_axis',(0.,0.,-1.));
#37531=DIRECTION('ref_axis',(0.,-1.,0.));
#37532=DIRECTION('',(0.,-1.,0.));
#37533=DIRECTION('',(-1.,0.,0.));
#37534=DIRECTION('',(0.,-1.,0.));
#37535=DIRECTION('',(-1.,0.,0.));
#37536=DIRECTION('center_axis',(0.,1.,0.));
#37537=DIRECTION('ref_axis',(0.,0.,-1.));
#37538=DIRECTION('',(0.,0.,-1.));
#37539=DIRECTION('',(-1.,0.,0.));
#37540=DIRECTION('',(0.,0.,-1.));
#37541=DIRECTION('center_axis',(0.,0.,1.));
#37542=DIRECTION('ref_axis',(0.,1.,0.));
#37543=DIRECTION('',(0.,1.,0.));
#37544=DIRECTION('',(-1.,0.,0.));
#37545=DIRECTION('',(0.,1.,0.));
#37546=DIRECTION('center_axis',(0.,-1.,0.));
#37547=DIRECTION('ref_axis',(0.,0.,1.));
#37548=DIRECTION('',(0.,0.,1.));
#37549=DIRECTION('',(0.,0.,1.));
#37550=DIRECTION('center_axis',(-1.,0.,0.));
#37551=DIRECTION('ref_axis',(0.,0.,1.));
#37552=DIRECTION('center_axis',(0.,0.,-1.));
#37553=DIRECTION('ref_axis',(0.,-1.,0.));
#37554=DIRECTION('',(0.,-1.,0.));
#37555=DIRECTION('',(-1.,0.,0.));
#37556=DIRECTION('',(0.,-1.,0.));
#37557=DIRECTION('',(-1.,0.,0.));
#37558=DIRECTION('center_axis',(0.,1.,0.));
#37559=DIRECTION('ref_axis',(0.,0.,-1.));
#37560=DIRECTION('',(0.,0.,-1.));
#37561=DIRECTION('',(-1.,0.,0.));
#37562=DIRECTION('',(0.,0.,-1.));
#37563=DIRECTION('center_axis',(0.,0.,1.));
#37564=DIRECTION('ref_axis',(0.,1.,0.));
#37565=DIRECTION('',(0.,1.,0.));
#37566=DIRECTION('',(-1.,0.,0.));
#37567=DIRECTION('',(0.,1.,0.));
#37568=DIRECTION('center_axis',(0.,-1.,0.));
#37569=DIRECTION('ref_axis',(0.,0.,1.));
#37570=DIRECTION('',(0.,0.,1.));
#37571=DIRECTION('',(0.,0.,1.));
#37572=DIRECTION('center_axis',(-1.,0.,0.));
#37573=DIRECTION('ref_axis',(0.,0.,1.));
#37574=DIRECTION('center_axis',(0.,0.,-1.));
#37575=DIRECTION('ref_axis',(0.,-1.,0.));
#37576=DIRECTION('',(0.,-1.,0.));
#37577=DIRECTION('',(-1.,0.,0.));
#37578=DIRECTION('',(0.,-1.,0.));
#37579=DIRECTION('',(-1.,0.,0.));
#37580=DIRECTION('center_axis',(0.,1.,0.));
#37581=DIRECTION('ref_axis',(0.,0.,-1.));
#37582=DIRECTION('',(0.,0.,-1.));
#37583=DIRECTION('',(-1.,0.,0.));
#37584=DIRECTION('',(0.,0.,-1.));
#37585=DIRECTION('center_axis',(0.,0.,1.));
#37586=DIRECTION('ref_axis',(0.,1.,0.));
#37587=DIRECTION('',(0.,1.,0.));
#37588=DIRECTION('',(-1.,0.,0.));
#37589=DIRECTION('',(0.,1.,0.));
#37590=DIRECTION('center_axis',(0.,-1.,0.));
#37591=DIRECTION('ref_axis',(0.,0.,1.));
#37592=DIRECTION('',(0.,0.,1.));
#37593=DIRECTION('',(0.,0.,1.));
#37594=DIRECTION('center_axis',(-1.,0.,0.));
#37595=DIRECTION('ref_axis',(0.,0.,1.));
#37596=DIRECTION('center_axis',(0.,0.,-1.));
#37597=DIRECTION('ref_axis',(0.,-1.,0.));
#37598=DIRECTION('',(0.,-1.,0.));
#37599=DIRECTION('',(-1.,0.,0.));
#37600=DIRECTION('',(0.,-1.,0.));
#37601=DIRECTION('',(-1.,0.,0.));
#37602=DIRECTION('center_axis',(0.,1.,0.));
#37603=DIRECTION('ref_axis',(0.,0.,-1.));
#37604=DIRECTION('',(0.,0.,-1.));
#37605=DIRECTION('',(-1.,0.,0.));
#37606=DIRECTION('',(0.,0.,-1.));
#37607=DIRECTION('center_axis',(0.,0.,1.));
#37608=DIRECTION('ref_axis',(0.,1.,0.));
#37609=DIRECTION('',(0.,1.,0.));
#37610=DIRECTION('',(-1.,0.,0.));
#37611=DIRECTION('',(0.,1.,0.));
#37612=DIRECTION('center_axis',(0.,-1.,0.));
#37613=DIRECTION('ref_axis',(0.,0.,1.));
#37614=DIRECTION('',(0.,0.,1.));
#37615=DIRECTION('',(0.,0.,1.));
#37616=DIRECTION('center_axis',(-1.,0.,0.));
#37617=DIRECTION('ref_axis',(0.,0.,1.));
#37618=DIRECTION('center_axis',(0.,0.,-1.));
#37619=DIRECTION('ref_axis',(0.,-1.,0.));
#37620=DIRECTION('',(0.,-1.,0.));
#37621=DIRECTION('',(-1.,0.,0.));
#37622=DIRECTION('',(0.,-1.,0.));
#37623=DIRECTION('',(-1.,0.,0.));
#37624=DIRECTION('center_axis',(0.,1.,0.));
#37625=DIRECTION('ref_axis',(0.,0.,-1.));
#37626=DIRECTION('',(0.,0.,-1.));
#37627=DIRECTION('',(-1.,0.,0.));
#37628=DIRECTION('',(0.,0.,-1.));
#37629=DIRECTION('center_axis',(0.,0.,1.));
#37630=DIRECTION('ref_axis',(0.,1.,0.));
#37631=DIRECTION('',(0.,1.,0.));
#37632=DIRECTION('',(-1.,0.,0.));
#37633=DIRECTION('',(0.,1.,0.));
#37634=DIRECTION('center_axis',(0.,-1.,0.));
#37635=DIRECTION('ref_axis',(0.,0.,1.));
#37636=DIRECTION('',(0.,0.,1.));
#37637=DIRECTION('',(0.,0.,1.));
#37638=DIRECTION('center_axis',(-1.,0.,0.));
#37639=DIRECTION('ref_axis',(0.,0.,1.));
#37640=DIRECTION('center_axis',(0.,0.,-1.));
#37641=DIRECTION('ref_axis',(0.,-1.,0.));
#37642=DIRECTION('',(0.,-1.,0.));
#37643=DIRECTION('',(-1.,0.,0.));
#37644=DIRECTION('',(0.,-1.,0.));
#37645=DIRECTION('',(-1.,0.,0.));
#37646=DIRECTION('center_axis',(0.,1.,0.));
#37647=DIRECTION('ref_axis',(0.,0.,-1.));
#37648=DIRECTION('',(0.,0.,-1.));
#37649=DIRECTION('',(-1.,0.,0.));
#37650=DIRECTION('',(0.,0.,-1.));
#37651=DIRECTION('center_axis',(0.,0.,1.));
#37652=DIRECTION('ref_axis',(0.,1.,0.));
#37653=DIRECTION('',(0.,1.,0.));
#37654=DIRECTION('',(-1.,0.,0.));
#37655=DIRECTION('',(0.,1.,0.));
#37656=DIRECTION('center_axis',(0.,-1.,0.));
#37657=DIRECTION('ref_axis',(0.,0.,1.));
#37658=DIRECTION('',(0.,0.,1.));
#37659=DIRECTION('',(0.,0.,1.));
#37660=DIRECTION('center_axis',(-1.,0.,0.));
#37661=DIRECTION('ref_axis',(0.,0.,1.));
#37662=DIRECTION('center_axis',(0.,0.,-1.));
#37663=DIRECTION('ref_axis',(0.,-1.,0.));
#37664=DIRECTION('',(0.,-1.,0.));
#37665=DIRECTION('',(-1.,0.,0.));
#37666=DIRECTION('',(0.,-1.,0.));
#37667=DIRECTION('',(-1.,0.,0.));
#37668=DIRECTION('center_axis',(0.,1.,0.));
#37669=DIRECTION('ref_axis',(0.,0.,-1.));
#37670=DIRECTION('',(0.,0.,-1.));
#37671=DIRECTION('',(-1.,0.,0.));
#37672=DIRECTION('',(0.,0.,-1.));
#37673=DIRECTION('center_axis',(0.,0.,1.));
#37674=DIRECTION('ref_axis',(0.,1.,0.));
#37675=DIRECTION('',(0.,1.,0.));
#37676=DIRECTION('',(-1.,0.,0.));
#37677=DIRECTION('',(0.,1.,0.));
#37678=DIRECTION('center_axis',(0.,-1.,0.));
#37679=DIRECTION('ref_axis',(0.,0.,1.));
#37680=DIRECTION('',(0.,0.,1.));
#37681=DIRECTION('',(0.,0.,1.));
#37682=DIRECTION('center_axis',(-1.,0.,0.));
#37683=DIRECTION('ref_axis',(0.,0.,1.));
#37684=DIRECTION('center_axis',(0.,0.,-1.));
#37685=DIRECTION('ref_axis',(0.,-1.,0.));
#37686=DIRECTION('',(0.,-1.,0.));
#37687=DIRECTION('',(-1.,0.,0.));
#37688=DIRECTION('',(0.,-1.,0.));
#37689=DIRECTION('',(-1.,0.,0.));
#37690=DIRECTION('center_axis',(0.,1.,0.));
#37691=DIRECTION('ref_axis',(0.,0.,-1.));
#37692=DIRECTION('',(0.,0.,-1.));
#37693=DIRECTION('',(-1.,0.,0.));
#37694=DIRECTION('',(0.,0.,-1.));
#37695=DIRECTION('center_axis',(0.,0.,1.));
#37696=DIRECTION('ref_axis',(0.,1.,0.));
#37697=DIRECTION('',(0.,1.,0.));
#37698=DIRECTION('',(-1.,0.,0.));
#37699=DIRECTION('',(0.,1.,0.));
#37700=DIRECTION('center_axis',(0.,-1.,0.));
#37701=DIRECTION('ref_axis',(0.,0.,1.));
#37702=DIRECTION('',(0.,0.,1.));
#37703=DIRECTION('',(0.,0.,1.));
#37704=DIRECTION('center_axis',(-1.,0.,0.));
#37705=DIRECTION('ref_axis',(0.,0.,1.));
#37706=DIRECTION('center_axis',(0.,0.,-1.));
#37707=DIRECTION('ref_axis',(0.,-1.,0.));
#37708=DIRECTION('',(0.,-1.,0.));
#37709=DIRECTION('',(-1.,0.,0.));
#37710=DIRECTION('',(0.,-1.,0.));
#37711=DIRECTION('',(-1.,0.,0.));
#37712=DIRECTION('center_axis',(0.,1.,0.));
#37713=DIRECTION('ref_axis',(0.,0.,-1.));
#37714=DIRECTION('',(0.,0.,-1.));
#37715=DIRECTION('',(-1.,0.,0.));
#37716=DIRECTION('',(0.,0.,-1.));
#37717=DIRECTION('center_axis',(0.,0.,1.));
#37718=DIRECTION('ref_axis',(0.,1.,0.));
#37719=DIRECTION('',(0.,1.,0.));
#37720=DIRECTION('',(-1.,0.,0.));
#37721=DIRECTION('',(0.,1.,0.));
#37722=DIRECTION('center_axis',(0.,-1.,0.));
#37723=DIRECTION('ref_axis',(0.,0.,1.));
#37724=DIRECTION('',(0.,0.,1.));
#37725=DIRECTION('',(0.,0.,1.));
#37726=DIRECTION('center_axis',(-1.,0.,0.));
#37727=DIRECTION('ref_axis',(0.,0.,1.));
#37728=DIRECTION('center_axis',(0.,0.,-1.));
#37729=DIRECTION('ref_axis',(0.,-1.,0.));
#37730=DIRECTION('',(0.,-1.,0.));
#37731=DIRECTION('',(-1.,0.,0.));
#37732=DIRECTION('',(0.,-1.,0.));
#37733=DIRECTION('',(-1.,0.,0.));
#37734=DIRECTION('center_axis',(0.,1.,0.));
#37735=DIRECTION('ref_axis',(0.,0.,-1.));
#37736=DIRECTION('',(0.,0.,-1.));
#37737=DIRECTION('',(-1.,0.,0.));
#37738=DIRECTION('',(0.,0.,-1.));
#37739=DIRECTION('center_axis',(0.,0.,1.));
#37740=DIRECTION('ref_axis',(0.,1.,0.));
#37741=DIRECTION('',(0.,1.,0.));
#37742=DIRECTION('',(-1.,0.,0.));
#37743=DIRECTION('',(0.,1.,0.));
#37744=DIRECTION('center_axis',(0.,-1.,0.));
#37745=DIRECTION('ref_axis',(0.,0.,1.));
#37746=DIRECTION('',(0.,0.,1.));
#37747=DIRECTION('',(0.,0.,1.));
#37748=DIRECTION('center_axis',(-1.,0.,0.));
#37749=DIRECTION('ref_axis',(0.,0.,1.));
#37750=DIRECTION('center_axis',(0.,0.,-1.));
#37751=DIRECTION('ref_axis',(0.,-1.,0.));
#37752=DIRECTION('',(0.,-1.,0.));
#37753=DIRECTION('',(-1.,0.,0.));
#37754=DIRECTION('',(0.,-1.,0.));
#37755=DIRECTION('',(-1.,0.,0.));
#37756=DIRECTION('center_axis',(0.,1.,0.));
#37757=DIRECTION('ref_axis',(0.,0.,-1.));
#37758=DIRECTION('',(0.,0.,-1.));
#37759=DIRECTION('',(-1.,0.,0.));
#37760=DIRECTION('',(0.,0.,-1.));
#37761=DIRECTION('center_axis',(0.,0.,1.));
#37762=DIRECTION('ref_axis',(0.,1.,0.));
#37763=DIRECTION('',(0.,1.,0.));
#37764=DIRECTION('',(-1.,0.,0.));
#37765=DIRECTION('',(0.,1.,0.));
#37766=DIRECTION('center_axis',(0.,-1.,0.));
#37767=DIRECTION('ref_axis',(0.,0.,1.));
#37768=DIRECTION('',(0.,0.,1.));
#37769=DIRECTION('',(0.,0.,1.));
#37770=DIRECTION('center_axis',(-1.,0.,0.));
#37771=DIRECTION('ref_axis',(0.,0.,1.));
#37772=DIRECTION('center_axis',(0.,0.,-1.));
#37773=DIRECTION('ref_axis',(0.,-1.,0.));
#37774=DIRECTION('',(0.,-1.,0.));
#37775=DIRECTION('',(-1.,0.,0.));
#37776=DIRECTION('',(0.,-1.,0.));
#37777=DIRECTION('',(-1.,0.,0.));
#37778=DIRECTION('center_axis',(0.,1.,0.));
#37779=DIRECTION('ref_axis',(0.,0.,-1.));
#37780=DIRECTION('',(0.,0.,-1.));
#37781=DIRECTION('',(-1.,0.,0.));
#37782=DIRECTION('',(0.,0.,-1.));
#37783=DIRECTION('center_axis',(0.,0.,1.));
#37784=DIRECTION('ref_axis',(0.,1.,0.));
#37785=DIRECTION('',(0.,1.,0.));
#37786=DIRECTION('',(-1.,0.,0.));
#37787=DIRECTION('',(0.,1.,0.));
#37788=DIRECTION('center_axis',(0.,-1.,0.));
#37789=DIRECTION('ref_axis',(0.,0.,1.));
#37790=DIRECTION('',(0.,0.,1.));
#37791=DIRECTION('',(0.,0.,1.));
#37792=DIRECTION('center_axis',(-1.,0.,0.));
#37793=DIRECTION('ref_axis',(0.,0.,1.));
#37794=DIRECTION('center_axis',(0.,0.,-1.));
#37795=DIRECTION('ref_axis',(0.,-1.,0.));
#37796=DIRECTION('',(0.,-1.,0.));
#37797=DIRECTION('',(-1.,0.,0.));
#37798=DIRECTION('',(0.,-1.,0.));
#37799=DIRECTION('',(-1.,0.,0.));
#37800=DIRECTION('center_axis',(0.,1.,0.));
#37801=DIRECTION('ref_axis',(0.,0.,-1.));
#37802=DIRECTION('',(0.,0.,-1.));
#37803=DIRECTION('',(-1.,0.,0.));
#37804=DIRECTION('',(0.,0.,-1.));
#37805=DIRECTION('center_axis',(0.,0.,1.));
#37806=DIRECTION('ref_axis',(0.,1.,0.));
#37807=DIRECTION('',(0.,1.,0.));
#37808=DIRECTION('',(-1.,0.,0.));
#37809=DIRECTION('',(0.,1.,0.));
#37810=DIRECTION('center_axis',(0.,-1.,0.));
#37811=DIRECTION('ref_axis',(0.,0.,1.));
#37812=DIRECTION('',(0.,0.,1.));
#37813=DIRECTION('',(0.,0.,1.));
#37814=DIRECTION('center_axis',(-1.,0.,0.));
#37815=DIRECTION('ref_axis',(0.,0.,1.));
#37816=DIRECTION('center_axis',(0.,0.,-1.));
#37817=DIRECTION('ref_axis',(0.,-1.,0.));
#37818=DIRECTION('',(0.,-1.,0.));
#37819=DIRECTION('',(-1.,0.,0.));
#37820=DIRECTION('',(0.,-1.,0.));
#37821=DIRECTION('',(-1.,0.,0.));
#37822=DIRECTION('center_axis',(0.,1.,0.));
#37823=DIRECTION('ref_axis',(0.,0.,-1.));
#37824=DIRECTION('',(0.,0.,-1.));
#37825=DIRECTION('',(-1.,0.,0.));
#37826=DIRECTION('',(0.,0.,-1.));
#37827=DIRECTION('center_axis',(0.,0.,1.));
#37828=DIRECTION('ref_axis',(0.,1.,0.));
#37829=DIRECTION('',(0.,1.,0.));
#37830=DIRECTION('',(-1.,0.,0.));
#37831=DIRECTION('',(0.,1.,0.));
#37832=DIRECTION('center_axis',(0.,-1.,0.));
#37833=DIRECTION('ref_axis',(0.,0.,1.));
#37834=DIRECTION('',(0.,0.,1.));
#37835=DIRECTION('',(0.,0.,1.));
#37836=DIRECTION('center_axis',(-1.,0.,0.));
#37837=DIRECTION('ref_axis',(0.,0.,1.));
#37838=DIRECTION('center_axis',(0.,0.,-1.));
#37839=DIRECTION('ref_axis',(0.,-1.,0.));
#37840=DIRECTION('',(0.,-1.,0.));
#37841=DIRECTION('',(-1.,0.,0.));
#37842=DIRECTION('',(0.,-1.,0.));
#37843=DIRECTION('',(-1.,0.,0.));
#37844=DIRECTION('center_axis',(0.,1.,0.));
#37845=DIRECTION('ref_axis',(0.,0.,-1.));
#37846=DIRECTION('',(0.,0.,-1.));
#37847=DIRECTION('',(-1.,0.,0.));
#37848=DIRECTION('',(0.,0.,-1.));
#37849=DIRECTION('center_axis',(0.,0.,1.));
#37850=DIRECTION('ref_axis',(0.,1.,0.));
#37851=DIRECTION('',(0.,1.,0.));
#37852=DIRECTION('',(-1.,0.,0.));
#37853=DIRECTION('',(0.,1.,0.));
#37854=DIRECTION('center_axis',(0.,-1.,0.));
#37855=DIRECTION('ref_axis',(0.,0.,1.));
#37856=DIRECTION('',(0.,0.,1.));
#37857=DIRECTION('',(0.,0.,1.));
#37858=DIRECTION('center_axis',(-1.,0.,0.));
#37859=DIRECTION('ref_axis',(0.,0.,1.));
#37860=DIRECTION('center_axis',(0.,0.,-1.));
#37861=DIRECTION('ref_axis',(0.,-1.,0.));
#37862=DIRECTION('',(0.,-1.,0.));
#37863=DIRECTION('',(-1.,0.,0.));
#37864=DIRECTION('',(0.,-1.,0.));
#37865=DIRECTION('',(-1.,0.,0.));
#37866=DIRECTION('center_axis',(0.,1.,0.));
#37867=DIRECTION('ref_axis',(0.,0.,-1.));
#37868=DIRECTION('',(0.,0.,-1.));
#37869=DIRECTION('',(-1.,0.,0.));
#37870=DIRECTION('',(0.,0.,-1.));
#37871=DIRECTION('center_axis',(0.,0.,1.));
#37872=DIRECTION('ref_axis',(0.,1.,0.));
#37873=DIRECTION('',(0.,1.,0.));
#37874=DIRECTION('',(-1.,0.,0.));
#37875=DIRECTION('',(0.,1.,0.));
#37876=DIRECTION('center_axis',(0.,-1.,0.));
#37877=DIRECTION('ref_axis',(0.,0.,1.));
#37878=DIRECTION('',(0.,0.,1.));
#37879=DIRECTION('',(0.,0.,1.));
#37880=DIRECTION('center_axis',(-1.,0.,0.));
#37881=DIRECTION('ref_axis',(0.,0.,1.));
#37882=DIRECTION('center_axis',(0.,0.,-1.));
#37883=DIRECTION('ref_axis',(0.,-1.,0.));
#37884=DIRECTION('',(0.,-1.,0.));
#37885=DIRECTION('',(-1.,0.,0.));
#37886=DIRECTION('',(0.,-1.,0.));
#37887=DIRECTION('',(-1.,0.,0.));
#37888=DIRECTION('center_axis',(0.,1.,0.));
#37889=DIRECTION('ref_axis',(0.,0.,-1.));
#37890=DIRECTION('',(0.,0.,-1.));
#37891=DIRECTION('',(-1.,0.,0.));
#37892=DIRECTION('',(0.,0.,-1.));
#37893=DIRECTION('center_axis',(0.,0.,1.));
#37894=DIRECTION('ref_axis',(0.,1.,0.));
#37895=DIRECTION('',(0.,1.,0.));
#37896=DIRECTION('',(-1.,0.,0.));
#37897=DIRECTION('',(0.,1.,0.));
#37898=DIRECTION('center_axis',(0.,-1.,0.));
#37899=DIRECTION('ref_axis',(0.,0.,1.));
#37900=DIRECTION('',(0.,0.,1.));
#37901=DIRECTION('',(0.,0.,1.));
#37902=DIRECTION('center_axis',(-1.,0.,0.));
#37903=DIRECTION('ref_axis',(0.,0.,1.));
#37904=DIRECTION('center_axis',(0.,0.,-1.));
#37905=DIRECTION('ref_axis',(0.,-1.,0.));
#37906=DIRECTION('',(0.,-1.,0.));
#37907=DIRECTION('',(-1.,0.,0.));
#37908=DIRECTION('',(0.,-1.,0.));
#37909=DIRECTION('',(-1.,0.,0.));
#37910=DIRECTION('center_axis',(0.,1.,0.));
#37911=DIRECTION('ref_axis',(0.,0.,-1.));
#37912=DIRECTION('',(0.,0.,-1.));
#37913=DIRECTION('',(-1.,0.,0.));
#37914=DIRECTION('',(0.,0.,-1.));
#37915=DIRECTION('center_axis',(0.,0.,1.));
#37916=DIRECTION('ref_axis',(0.,1.,0.));
#37917=DIRECTION('',(0.,1.,0.));
#37918=DIRECTION('',(-1.,0.,0.));
#37919=DIRECTION('',(0.,1.,0.));
#37920=DIRECTION('center_axis',(0.,-1.,0.));
#37921=DIRECTION('ref_axis',(0.,0.,1.));
#37922=DIRECTION('',(0.,0.,1.));
#37923=DIRECTION('',(0.,0.,1.));
#37924=DIRECTION('center_axis',(-1.,0.,0.));
#37925=DIRECTION('ref_axis',(0.,0.,1.));
#37926=DIRECTION('center_axis',(0.,0.,-1.));
#37927=DIRECTION('ref_axis',(0.,-1.,0.));
#37928=DIRECTION('',(0.,-1.,0.));
#37929=DIRECTION('',(-1.,0.,0.));
#37930=DIRECTION('',(0.,-1.,0.));
#37931=DIRECTION('',(-1.,0.,0.));
#37932=DIRECTION('center_axis',(0.,1.,0.));
#37933=DIRECTION('ref_axis',(0.,0.,-1.));
#37934=DIRECTION('',(0.,0.,-1.));
#37935=DIRECTION('',(-1.,0.,0.));
#37936=DIRECTION('',(0.,0.,-1.));
#37937=DIRECTION('center_axis',(0.,0.,1.));
#37938=DIRECTION('ref_axis',(0.,1.,0.));
#37939=DIRECTION('',(0.,1.,0.));
#37940=DIRECTION('',(-1.,0.,0.));
#37941=DIRECTION('',(0.,1.,0.));
#37942=DIRECTION('center_axis',(0.,-1.,0.));
#37943=DIRECTION('ref_axis',(0.,0.,1.));
#37944=DIRECTION('',(0.,0.,1.));
#37945=DIRECTION('',(0.,0.,1.));
#37946=DIRECTION('center_axis',(-1.,0.,0.));
#37947=DIRECTION('ref_axis',(0.,0.,1.));
#37948=DIRECTION('center_axis',(0.,0.,-1.));
#37949=DIRECTION('ref_axis',(0.,-1.,0.));
#37950=DIRECTION('',(0.,-1.,0.));
#37951=DIRECTION('',(-1.,0.,0.));
#37952=DIRECTION('',(0.,-1.,0.));
#37953=DIRECTION('',(-1.,0.,0.));
#37954=DIRECTION('center_axis',(0.,1.,0.));
#37955=DIRECTION('ref_axis',(0.,0.,-1.));
#37956=DIRECTION('',(0.,0.,-1.));
#37957=DIRECTION('',(-1.,0.,0.));
#37958=DIRECTION('',(0.,0.,-1.));
#37959=DIRECTION('center_axis',(0.,0.,1.));
#37960=DIRECTION('ref_axis',(0.,1.,0.));
#37961=DIRECTION('',(0.,1.,0.));
#37962=DIRECTION('',(-1.,0.,0.));
#37963=DIRECTION('',(0.,1.,0.));
#37964=DIRECTION('center_axis',(0.,-1.,0.));
#37965=DIRECTION('ref_axis',(0.,0.,1.));
#37966=DIRECTION('',(0.,0.,1.));
#37967=DIRECTION('',(0.,0.,1.));
#37968=DIRECTION('center_axis',(-1.,0.,0.));
#37969=DIRECTION('ref_axis',(0.,0.,1.));
#37970=DIRECTION('center_axis',(0.,0.,-1.));
#37971=DIRECTION('ref_axis',(0.,-1.,0.));
#37972=DIRECTION('',(0.,-1.,0.));
#37973=DIRECTION('',(-1.,0.,0.));
#37974=DIRECTION('',(0.,-1.,0.));
#37975=DIRECTION('',(-1.,0.,0.));
#37976=DIRECTION('center_axis',(0.,1.,0.));
#37977=DIRECTION('ref_axis',(0.,0.,-1.));
#37978=DIRECTION('',(0.,0.,-1.));
#37979=DIRECTION('',(-1.,0.,0.));
#37980=DIRECTION('',(0.,0.,-1.));
#37981=DIRECTION('center_axis',(0.,0.,1.));
#37982=DIRECTION('ref_axis',(0.,1.,0.));
#37983=DIRECTION('',(0.,1.,0.));
#37984=DIRECTION('',(-1.,0.,0.));
#37985=DIRECTION('',(0.,1.,0.));
#37986=DIRECTION('center_axis',(0.,-1.,0.));
#37987=DIRECTION('ref_axis',(0.,0.,1.));
#37988=DIRECTION('',(0.,0.,1.));
#37989=DIRECTION('',(0.,0.,1.));
#37990=DIRECTION('center_axis',(-1.,0.,0.));
#37991=DIRECTION('ref_axis',(0.,0.,1.));
#37992=DIRECTION('center_axis',(0.,0.,-1.));
#37993=DIRECTION('ref_axis',(0.,-1.,0.));
#37994=DIRECTION('',(0.,-1.,0.));
#37995=DIRECTION('',(-1.,0.,0.));
#37996=DIRECTION('',(0.,-1.,0.));
#37997=DIRECTION('',(-1.,0.,0.));
#37998=DIRECTION('center_axis',(0.,1.,0.));
#37999=DIRECTION('ref_axis',(0.,0.,-1.));
#38000=DIRECTION('',(0.,0.,-1.));
#38001=DIRECTION('',(-1.,0.,0.));
#38002=DIRECTION('',(0.,0.,-1.));
#38003=DIRECTION('center_axis',(0.,0.,1.));
#38004=DIRECTION('ref_axis',(0.,1.,0.));
#38005=DIRECTION('',(0.,1.,0.));
#38006=DIRECTION('',(-1.,0.,0.));
#38007=DIRECTION('',(0.,1.,0.));
#38008=DIRECTION('center_axis',(0.,-1.,0.));
#38009=DIRECTION('ref_axis',(0.,0.,1.));
#38010=DIRECTION('',(0.,0.,1.));
#38011=DIRECTION('',(0.,0.,1.));
#38012=DIRECTION('center_axis',(-1.,0.,0.));
#38013=DIRECTION('ref_axis',(0.,0.,1.));
#38014=DIRECTION('center_axis',(0.,0.,-1.));
#38015=DIRECTION('ref_axis',(0.,-1.,0.));
#38016=DIRECTION('',(0.,-1.,0.));
#38017=DIRECTION('',(-1.,0.,0.));
#38018=DIRECTION('',(0.,-1.,0.));
#38019=DIRECTION('',(-1.,0.,0.));
#38020=DIRECTION('center_axis',(0.,1.,0.));
#38021=DIRECTION('ref_axis',(0.,0.,-1.));
#38022=DIRECTION('',(0.,0.,-1.));
#38023=DIRECTION('',(-1.,0.,0.));
#38024=DIRECTION('',(0.,0.,-1.));
#38025=DIRECTION('center_axis',(0.,0.,1.));
#38026=DIRECTION('ref_axis',(0.,1.,0.));
#38027=DIRECTION('',(0.,1.,0.));
#38028=DIRECTION('',(-1.,0.,0.));
#38029=DIRECTION('',(0.,1.,0.));
#38030=DIRECTION('center_axis',(0.,-1.,0.));
#38031=DIRECTION('ref_axis',(0.,0.,1.));
#38032=DIRECTION('',(0.,0.,1.));
#38033=DIRECTION('',(0.,0.,1.));
#38034=DIRECTION('center_axis',(-1.,0.,0.));
#38035=DIRECTION('ref_axis',(0.,0.,1.));
#38036=DIRECTION('center_axis',(0.,0.,-1.));
#38037=DIRECTION('ref_axis',(0.,-1.,0.));
#38038=DIRECTION('',(0.,-1.,0.));
#38039=DIRECTION('',(-1.,0.,0.));
#38040=DIRECTION('',(0.,-1.,0.));
#38041=DIRECTION('',(-1.,0.,0.));
#38042=DIRECTION('center_axis',(0.,1.,0.));
#38043=DIRECTION('ref_axis',(0.,0.,-1.));
#38044=DIRECTION('',(0.,0.,-1.));
#38045=DIRECTION('',(-1.,0.,0.));
#38046=DIRECTION('',(0.,0.,-1.));
#38047=DIRECTION('center_axis',(0.,0.,1.));
#38048=DIRECTION('ref_axis',(0.,1.,0.));
#38049=DIRECTION('',(0.,1.,0.));
#38050=DIRECTION('',(-1.,0.,0.));
#38051=DIRECTION('',(0.,1.,0.));
#38052=DIRECTION('center_axis',(0.,-1.,0.));
#38053=DIRECTION('ref_axis',(0.,0.,1.));
#38054=DIRECTION('',(0.,0.,1.));
#38055=DIRECTION('',(0.,0.,1.));
#38056=DIRECTION('center_axis',(-1.,0.,0.));
#38057=DIRECTION('ref_axis',(0.,0.,1.));
#38058=DIRECTION('center_axis',(0.,0.,-1.));
#38059=DIRECTION('ref_axis',(0.,-1.,0.));
#38060=DIRECTION('',(0.,-1.,0.));
#38061=DIRECTION('',(-1.,0.,0.));
#38062=DIRECTION('',(0.,-1.,0.));
#38063=DIRECTION('',(-1.,0.,0.));
#38064=DIRECTION('center_axis',(0.,1.,0.));
#38065=DIRECTION('ref_axis',(0.,0.,-1.));
#38066=DIRECTION('',(0.,0.,-1.));
#38067=DIRECTION('',(-1.,0.,0.));
#38068=DIRECTION('',(0.,0.,-1.));
#38069=DIRECTION('center_axis',(0.,0.,1.));
#38070=DIRECTION('ref_axis',(0.,1.,0.));
#38071=DIRECTION('',(0.,1.,0.));
#38072=DIRECTION('',(-1.,0.,0.));
#38073=DIRECTION('',(0.,1.,0.));
#38074=DIRECTION('center_axis',(0.,-1.,0.));
#38075=DIRECTION('ref_axis',(0.,0.,1.));
#38076=DIRECTION('',(0.,0.,1.));
#38077=DIRECTION('',(0.,0.,1.));
#38078=DIRECTION('center_axis',(-1.,0.,0.));
#38079=DIRECTION('ref_axis',(0.,0.,1.));
#38080=DIRECTION('center_axis',(0.,0.,-1.));
#38081=DIRECTION('ref_axis',(0.,-1.,0.));
#38082=DIRECTION('',(0.,-1.,0.));
#38083=DIRECTION('',(-1.,0.,0.));
#38084=DIRECTION('',(0.,-1.,0.));
#38085=DIRECTION('',(-1.,0.,0.));
#38086=DIRECTION('center_axis',(0.,1.,0.));
#38087=DIRECTION('ref_axis',(0.,0.,-1.));
#38088=DIRECTION('',(0.,0.,-1.));
#38089=DIRECTION('',(-1.,0.,0.));
#38090=DIRECTION('',(0.,0.,-1.));
#38091=DIRECTION('center_axis',(0.,0.,1.));
#38092=DIRECTION('ref_axis',(0.,1.,0.));
#38093=DIRECTION('',(0.,1.,0.));
#38094=DIRECTION('',(-1.,0.,0.));
#38095=DIRECTION('',(0.,1.,0.));
#38096=DIRECTION('center_axis',(0.,-1.,0.));
#38097=DIRECTION('ref_axis',(0.,0.,1.));
#38098=DIRECTION('',(0.,0.,1.));
#38099=DIRECTION('',(0.,0.,1.));
#38100=DIRECTION('center_axis',(-1.,0.,0.));
#38101=DIRECTION('ref_axis',(0.,0.,1.));
#38102=DIRECTION('center_axis',(0.,0.,-1.));
#38103=DIRECTION('ref_axis',(0.,-1.,0.));
#38104=DIRECTION('',(0.,-1.,0.));
#38105=DIRECTION('',(-1.,0.,0.));
#38106=DIRECTION('',(0.,-1.,0.));
#38107=DIRECTION('',(-1.,0.,0.));
#38108=DIRECTION('center_axis',(0.,1.,0.));
#38109=DIRECTION('ref_axis',(0.,0.,-1.));
#38110=DIRECTION('',(0.,0.,-1.));
#38111=DIRECTION('',(-1.,0.,0.));
#38112=DIRECTION('',(0.,0.,-1.));
#38113=DIRECTION('center_axis',(0.,0.,1.));
#38114=DIRECTION('ref_axis',(0.,1.,0.));
#38115=DIRECTION('',(0.,1.,0.));
#38116=DIRECTION('',(-1.,0.,0.));
#38117=DIRECTION('',(0.,1.,0.));
#38118=DIRECTION('center_axis',(0.,-1.,0.));
#38119=DIRECTION('ref_axis',(0.,0.,1.));
#38120=DIRECTION('',(0.,0.,1.));
#38121=DIRECTION('',(0.,0.,1.));
#38122=DIRECTION('center_axis',(-1.,0.,0.));
#38123=DIRECTION('ref_axis',(0.,0.,1.));
#38124=DIRECTION('center_axis',(0.,0.,-1.));
#38125=DIRECTION('ref_axis',(0.,-1.,0.));
#38126=DIRECTION('',(0.,-1.,0.));
#38127=DIRECTION('',(-1.,0.,0.));
#38128=DIRECTION('',(0.,-1.,0.));
#38129=DIRECTION('',(-1.,0.,0.));
#38130=DIRECTION('center_axis',(0.,1.,0.));
#38131=DIRECTION('ref_axis',(0.,0.,-1.));
#38132=DIRECTION('',(0.,0.,-1.));
#38133=DIRECTION('',(-1.,0.,0.));
#38134=DIRECTION('',(0.,0.,-1.));
#38135=DIRECTION('center_axis',(0.,0.,1.));
#38136=DIRECTION('ref_axis',(0.,1.,0.));
#38137=DIRECTION('',(0.,1.,0.));
#38138=DIRECTION('',(-1.,0.,0.));
#38139=DIRECTION('',(0.,1.,0.));
#38140=DIRECTION('center_axis',(0.,-1.,0.));
#38141=DIRECTION('ref_axis',(0.,0.,1.));
#38142=DIRECTION('',(0.,0.,1.));
#38143=DIRECTION('',(0.,0.,1.));
#38144=DIRECTION('center_axis',(-1.,0.,0.));
#38145=DIRECTION('ref_axis',(0.,0.,1.));
#38146=DIRECTION('center_axis',(0.,0.,-1.));
#38147=DIRECTION('ref_axis',(0.,-1.,0.));
#38148=DIRECTION('',(0.,-1.,0.));
#38149=DIRECTION('',(-1.,0.,0.));
#38150=DIRECTION('',(0.,-1.,0.));
#38151=DIRECTION('',(-1.,0.,0.));
#38152=DIRECTION('center_axis',(0.,1.,0.));
#38153=DIRECTION('ref_axis',(0.,0.,-1.));
#38154=DIRECTION('',(0.,0.,-1.));
#38155=DIRECTION('',(-1.,0.,0.));
#38156=DIRECTION('',(0.,0.,-1.));
#38157=DIRECTION('center_axis',(0.,0.,1.));
#38158=DIRECTION('ref_axis',(0.,1.,0.));
#38159=DIRECTION('',(0.,1.,0.));
#38160=DIRECTION('',(-1.,0.,0.));
#38161=DIRECTION('',(0.,1.,0.));
#38162=DIRECTION('center_axis',(0.,-1.,0.));
#38163=DIRECTION('ref_axis',(0.,0.,1.));
#38164=DIRECTION('',(0.,0.,1.));
#38165=DIRECTION('',(0.,0.,1.));
#38166=DIRECTION('center_axis',(-1.,0.,0.));
#38167=DIRECTION('ref_axis',(0.,0.,1.));
#38168=DIRECTION('center_axis',(0.,0.,-1.));
#38169=DIRECTION('ref_axis',(0.,-1.,0.));
#38170=DIRECTION('',(0.,-1.,0.));
#38171=DIRECTION('',(-1.,0.,0.));
#38172=DIRECTION('',(0.,-1.,0.));
#38173=DIRECTION('',(-1.,0.,0.));
#38174=DIRECTION('center_axis',(0.,1.,0.));
#38175=DIRECTION('ref_axis',(0.,0.,-1.));
#38176=DIRECTION('',(0.,0.,-1.));
#38177=DIRECTION('',(-1.,0.,0.));
#38178=DIRECTION('',(0.,0.,-1.));
#38179=DIRECTION('center_axis',(0.,0.,1.));
#38180=DIRECTION('ref_axis',(0.,1.,0.));
#38181=DIRECTION('',(0.,1.,0.));
#38182=DIRECTION('',(-1.,0.,0.));
#38183=DIRECTION('',(0.,1.,0.));
#38184=DIRECTION('center_axis',(0.,-1.,0.));
#38185=DIRECTION('ref_axis',(0.,0.,1.));
#38186=DIRECTION('',(0.,0.,1.));
#38187=DIRECTION('',(0.,0.,1.));
#38188=DIRECTION('center_axis',(-1.,0.,0.));
#38189=DIRECTION('ref_axis',(0.,0.,1.));
#38190=DIRECTION('center_axis',(0.,0.,-1.));
#38191=DIRECTION('ref_axis',(0.,-1.,0.));
#38192=DIRECTION('',(0.,-1.,0.));
#38193=DIRECTION('',(-1.,0.,0.));
#38194=DIRECTION('',(0.,-1.,0.));
#38195=DIRECTION('',(-1.,0.,0.));
#38196=DIRECTION('center_axis',(0.,1.,0.));
#38197=DIRECTION('ref_axis',(0.,0.,-1.));
#38198=DIRECTION('',(0.,0.,-1.));
#38199=DIRECTION('',(-1.,0.,0.));
#38200=DIRECTION('',(0.,0.,-1.));
#38201=DIRECTION('center_axis',(0.,0.,1.));
#38202=DIRECTION('ref_axis',(0.,1.,0.));
#38203=DIRECTION('',(0.,1.,0.));
#38204=DIRECTION('',(-1.,0.,0.));
#38205=DIRECTION('',(0.,1.,0.));
#38206=DIRECTION('center_axis',(0.,-1.,0.));
#38207=DIRECTION('ref_axis',(0.,0.,1.));
#38208=DIRECTION('',(0.,0.,1.));
#38209=DIRECTION('',(0.,0.,1.));
#38210=DIRECTION('center_axis',(-1.,0.,0.));
#38211=DIRECTION('ref_axis',(0.,0.,1.));
#38212=DIRECTION('center_axis',(0.,0.,-1.));
#38213=DIRECTION('ref_axis',(0.,-1.,0.));
#38214=DIRECTION('',(0.,-1.,0.));
#38215=DIRECTION('',(-1.,0.,0.));
#38216=DIRECTION('',(0.,-1.,0.));
#38217=DIRECTION('',(-1.,0.,0.));
#38218=DIRECTION('center_axis',(0.,1.,0.));
#38219=DIRECTION('ref_axis',(0.,0.,-1.));
#38220=DIRECTION('',(0.,0.,-1.));
#38221=DIRECTION('',(-1.,0.,0.));
#38222=DIRECTION('',(0.,0.,-1.));
#38223=DIRECTION('center_axis',(0.,0.,1.));
#38224=DIRECTION('ref_axis',(0.,1.,0.));
#38225=DIRECTION('',(0.,1.,0.));
#38226=DIRECTION('',(-1.,0.,0.));
#38227=DIRECTION('',(0.,1.,0.));
#38228=DIRECTION('center_axis',(0.,-1.,0.));
#38229=DIRECTION('ref_axis',(0.,0.,1.));
#38230=DIRECTION('',(0.,0.,1.));
#38231=DIRECTION('',(0.,0.,1.));
#38232=DIRECTION('center_axis',(-1.,0.,0.));
#38233=DIRECTION('ref_axis',(0.,0.,1.));
#38234=DIRECTION('center_axis',(0.,0.,-1.));
#38235=DIRECTION('ref_axis',(0.,-1.,0.));
#38236=DIRECTION('',(0.,-1.,0.));
#38237=DIRECTION('',(-1.,0.,0.));
#38238=DIRECTION('',(0.,-1.,0.));
#38239=DIRECTION('',(-1.,0.,0.));
#38240=DIRECTION('center_axis',(0.,1.,0.));
#38241=DIRECTION('ref_axis',(0.,0.,-1.));
#38242=DIRECTION('',(0.,0.,-1.));
#38243=DIRECTION('',(-1.,0.,0.));
#38244=DIRECTION('',(0.,0.,-1.));
#38245=DIRECTION('center_axis',(0.,0.,1.));
#38246=DIRECTION('ref_axis',(0.,1.,0.));
#38247=DIRECTION('',(0.,1.,0.));
#38248=DIRECTION('',(-1.,0.,0.));
#38249=DIRECTION('',(0.,1.,0.));
#38250=DIRECTION('center_axis',(0.,-1.,0.));
#38251=DIRECTION('ref_axis',(0.,0.,1.));
#38252=DIRECTION('',(0.,0.,1.));
#38253=DIRECTION('',(0.,0.,1.));
#38254=DIRECTION('center_axis',(-1.,0.,0.));
#38255=DIRECTION('ref_axis',(0.,0.,1.));
#38256=DIRECTION('center_axis',(1.,0.,0.));
#38257=DIRECTION('ref_axis',(0.,0.,-1.));
#38258=DIRECTION('center_axis',(1.,0.,0.));
#38259=DIRECTION('ref_axis',(0.,0.,-1.));
#38260=DIRECTION('',(1.,0.,0.));
#38261=DIRECTION('center_axis',(-1.,0.,0.));
#38262=DIRECTION('ref_axis',(0.,0.,-1.));
#38263=DIRECTION('center_axis',(1.,0.,0.));
#38264=DIRECTION('ref_axis',(0.,0.,-1.));
#38265=DIRECTION('center_axis',(1.,0.,0.));
#38266=DIRECTION('ref_axis',(0.,0.,-1.));
#38267=DIRECTION('',(1.,0.,0.));
#38268=DIRECTION('center_axis',(-1.,0.,0.));
#38269=DIRECTION('ref_axis',(0.,0.,-1.));
#38270=DIRECTION('center_axis',(0.,-1.,0.));
#38271=DIRECTION('ref_axis',(0.,0.,-1.));
#38272=DIRECTION('',(0.,0.,-1.));
#38273=DIRECTION('',(1.,0.,0.));
#38274=DIRECTION('',(0.,0.,-1.));
#38275=DIRECTION('',(1.,0.,0.));
#38276=DIRECTION('center_axis',(1.,0.,0.));
#38277=DIRECTION('ref_axis',(0.,2.7755575615629E-15,1.));
#38278=DIRECTION('center_axis',(1.,0.,0.));
#38279=DIRECTION('ref_axis',(0.,2.7755575615629E-15,1.));
#38280=DIRECTION('center_axis',(1.,0.,0.));
#38281=DIRECTION('ref_axis',(0.,2.7755575615629E-15,1.));
#38282=DIRECTION('',(1.,0.,0.));
#38283=DIRECTION('center_axis',(0.,0.,1.));
#38284=DIRECTION('ref_axis',(0.,-1.,0.));
#38285=DIRECTION('',(0.,-1.,0.));
#38286=DIRECTION('',(0.,-1.,0.));
#38287=DIRECTION('',(1.,0.,0.));
#38288=DIRECTION('center_axis',(1.,0.,0.));
#38289=DIRECTION('ref_axis',(0.,1.,3.33066907387539E-14));
#38290=DIRECTION('center_axis',(1.,0.,0.));
#38291=DIRECTION('ref_axis',(0.,1.,3.33066907387539E-14));
#38292=DIRECTION('center_axis',(1.,0.,0.));
#38293=DIRECTION('ref_axis',(0.,1.,3.33066907387539E-14));
#38294=DIRECTION('',(1.,0.,0.));
#38295=DIRECTION('center_axis',(0.,1.,0.));
#38296=DIRECTION('ref_axis',(0.,0.,1.));
#38297=DIRECTION('',(0.,0.,1.));
#38298=DIRECTION('',(0.,0.,1.));
#38299=DIRECTION('',(1.,0.,0.));
#38300=DIRECTION('center_axis',(1.,0.,0.));
#38301=DIRECTION('ref_axis',(0.,0.,-1.));
#38302=DIRECTION('center_axis',(1.,0.,0.));
#38303=DIRECTION('ref_axis',(0.,0.,-1.));
#38304=DIRECTION('center_axis',(1.,0.,0.));
#38305=DIRECTION('ref_axis',(0.,0.,-1.));
#38306=DIRECTION('',(1.,0.,0.));
#38307=DIRECTION('center_axis',(0.,0.,-1.));
#38308=DIRECTION('ref_axis',(0.,1.,0.));
#38309=DIRECTION('',(0.,1.,0.));
#38310=DIRECTION('',(0.,1.,0.));
#38311=DIRECTION('',(1.,0.,0.));
#38312=DIRECTION('center_axis',(1.,0.,0.));
#38313=DIRECTION('ref_axis',(0.,-1.,3.81639164714899E-15));
#38314=DIRECTION('center_axis',(1.,0.,0.));
#38315=DIRECTION('ref_axis',(0.,-1.,3.81639164714899E-15));
#38316=DIRECTION('center_axis',(1.,0.,0.));
#38317=DIRECTION('ref_axis',(0.,-1.,3.81639164714899E-15));
#38318=DIRECTION('center_axis',(1.,0.,0.));
#38319=DIRECTION('ref_axis',(0.,0.,-1.));
#38320=DIRECTION('center_axis',(1.,0.,0.));
#38321=DIRECTION('ref_axis',(0.,0.,-1.));
#69950=CARTESIAN_POINT('',(0.,0.,0.));
#69951=CARTESIAN_POINT('Ctrl Pts',(18.3,110.643929117918,2.64843108169734));
#69952=CARTESIAN_POINT('Ctrl Pts',(18.1272,110.643929117918,2.64843108169734));
#69953=CARTESIAN_POINT('Ctrl Pts',(18.3,110.643929117918,2.78376536481082));
#69954=CARTESIAN_POINT('Ctrl Pts',(18.1272,110.643929117918,2.78376536481082));
#69955=CARTESIAN_POINT('Ctrl Pts',(18.3,110.529331588745,2.86452936045825));
#69956=CARTESIAN_POINT('Ctrl Pts',(18.1272,110.529331588745,2.86452936045825));
#69957=CARTESIAN_POINT('',(18.3,110.643929117918,2.64843108169734));
#69958=CARTESIAN_POINT('',(18.3,110.529331588745,2.86452936045825));
#69959=CARTESIAN_POINT('Ctrl Pts',(18.3,110.643929117918,2.64843108169734));
#69960=CARTESIAN_POINT('Ctrl Pts',(18.3,110.643929117918,2.78376536481082));
#69961=CARTESIAN_POINT('Ctrl Pts',(18.3,110.529331588745,2.86452936045825));
#69962=CARTESIAN_POINT('',(18.18,110.643929117918,2.64843108169734));
#69963=CARTESIAN_POINT('',(18.3,110.643929117918,2.64843108169734));
#69964=CARTESIAN_POINT('',(18.18,110.529331588745,2.86452936045825));
#69965=CARTESIAN_POINT('Ctrl Pts',(18.18,110.643929117918,2.64843108169734));
#69966=CARTESIAN_POINT('Ctrl Pts',(18.18,110.643929117918,2.78376536481082));
#69967=CARTESIAN_POINT('Ctrl Pts',(18.18,110.529331588745,2.86452936045825));
#69968=CARTESIAN_POINT('',(18.3,110.529331588745,2.86452936045825));
#69969=CARTESIAN_POINT('Ctrl Pts',(18.3,110.514051938057,2.41869034282863));
#69970=CARTESIAN_POINT('Ctrl Pts',(18.1272,110.514051938057,2.41869034282863));
#69971=CARTESIAN_POINT('Ctrl Pts',(18.3,110.643929117918,2.51091407649219));
#69972=CARTESIAN_POINT('Ctrl Pts',(18.1272,110.643929117918,2.51091407649219));
#69973=CARTESIAN_POINT('Ctrl Pts',(18.3,110.643929117918,2.64843108169734));
#69974=CARTESIAN_POINT('Ctrl Pts',(18.1272,110.643929117918,2.64843108169734));
#69975=CARTESIAN_POINT('',(18.3,110.514051938057,2.41869034282863));
#69976=CARTESIAN_POINT('Ctrl Pts',(18.3,110.514051938057,2.41869034282863));
#69977=CARTESIAN_POINT('Ctrl Pts',(18.3,110.643929117918,2.51091407649219));
#69978=CARTESIAN_POINT('Ctrl Pts',(18.3,110.643929117918,2.64843108169734));
#69979=CARTESIAN_POINT('',(18.18,110.514051938057,2.41869034282863));
#69980=CARTESIAN_POINT('',(18.3,110.514051938057,2.41869034282863));
#69981=CARTESIAN_POINT('Ctrl Pts',(18.18,110.514051938057,2.41869034282863));
#69982=CARTESIAN_POINT('Ctrl Pts',(18.18,110.643929117918,2.51091407649219));
#69983=CARTESIAN_POINT('Ctrl Pts',(18.18,110.643929117918,2.64843108169734));
#69984=CARTESIAN_POINT('Ctrl Pts',(18.3,109.989085966349,2.32646660916507));
#69985=CARTESIAN_POINT('Ctrl Pts',(18.1272,109.989085966349,2.32646660916507));
#69986=CARTESIAN_POINT('Ctrl Pts',(18.3,110.384174609184,2.32646660916507));
#69987=CARTESIAN_POINT('Ctrl Pts',(18.1272,110.384174609184,2.32646660916507));
#69988=CARTESIAN_POINT('Ctrl Pts',(18.3,110.514051938057,2.41869034282863));
#69989=CARTESIAN_POINT('Ctrl Pts',(18.1272,110.514051938057,2.41869034282863));
#69990=CARTESIAN_POINT('',(18.3,109.989085966349,2.32646660916507));
#69991=CARTESIAN_POINT('Ctrl Pts',(18.3,109.989085966349,2.32646660916507));
#69992=CARTESIAN_POINT('Ctrl Pts',(18.3,110.384174609184,2.32646660916507));
#69993=CARTESIAN_POINT('Ctrl Pts',(18.3,110.514051938057,2.41869034282863));
#69994=CARTESIAN_POINT('',(18.18,109.989085966349,2.32646660916507));
#69995=CARTESIAN_POINT('',(18.3,109.989085966349,2.32646660916507));
#69996=CARTESIAN_POINT('Ctrl Pts',(18.18,109.989085966349,2.32646660916507));
#69997=CARTESIAN_POINT('Ctrl Pts',(18.18,110.384174609184,2.32646660916507));
#69998=CARTESIAN_POINT('Ctrl Pts',(18.18,110.514051938057,2.41869034282863));
#69999=CARTESIAN_POINT('Ctrl Pts',(18.3,109.465211504698,2.41869034282863));
#70000=CARTESIAN_POINT('Ctrl Pts',(18.1272,109.465211504698,2.41869034282863));
#70001=CARTESIAN_POINT('Ctrl Pts',(18.3,109.596180194616,2.32646660916507));
#70002=CARTESIAN_POINT('Ctrl Pts',(18.1272,109.596180194616,2.32646660916507));
#70003=CARTESIAN_POINT('Ctrl Pts',(18.3,109.989085966349,2.32646660916507));
#70004=CARTESIAN_POINT('Ctrl Pts',(18.1272,109.989085966349,2.32646660916507));
#70005=CARTESIAN_POINT('',(18.3,109.465211504698,2.41869034282863));
#70006=CARTESIAN_POINT('Ctrl Pts',(18.3,109.465211504698,2.41869034282863));
#70007=CARTESIAN_POINT('Ctrl Pts',(18.3,109.596180194616,2.32646660916507));
#70008=CARTESIAN_POINT('Ctrl Pts',(18.3,109.989085966349,2.32646660916507));
#70009=CARTESIAN_POINT('',(18.18,109.465211504698,2.41869034282863));
#70010=CARTESIAN_POINT('',(18.3,109.465211504698,2.41869034282863));
#70011=CARTESIAN_POINT('Ctrl Pts',(18.18,109.465211504698,2.41869034282863));
#70012=CARTESIAN_POINT('Ctrl Pts',(18.18,109.596180194616,2.32646660916507));
#70013=CARTESIAN_POINT('Ctrl Pts',(18.18,109.989085966349,2.32646660916507));
#70014=CARTESIAN_POINT('Ctrl Pts',(18.3,109.334242814779,2.64624821059406));
#70015=CARTESIAN_POINT('Ctrl Pts',(18.1272,109.334242814779,2.64624821059406));
#70016=CARTESIAN_POINT('Ctrl Pts',(18.3,109.334242814779,2.51091407649219));
#70017=CARTESIAN_POINT('Ctrl Pts',(18.1272,109.334242814779,2.51091407649219));
#70018=CARTESIAN_POINT('Ctrl Pts',(18.3,109.465211504698,2.41869034282863));
#70019=CARTESIAN_POINT('Ctrl Pts',(18.1272,109.465211504698,2.41869034282863));
#70020=CARTESIAN_POINT('',(18.3,109.334242814779,2.64624821059406));
#70021=CARTESIAN_POINT('Ctrl Pts',(18.3,109.334242814779,2.64624821059406));
#70022=CARTESIAN_POINT('Ctrl Pts',(18.3,109.334242814779,2.51091407649219));
#70023=CARTESIAN_POINT('Ctrl Pts',(18.3,109.465211504698,2.41869034282863));
#70024=CARTESIAN_POINT('',(18.18,109.334242814779,2.64624821059406));
#70025=CARTESIAN_POINT('',(18.3,109.334242814779,2.64624821059406));
#70026=CARTESIAN_POINT('Ctrl Pts',(18.18,109.334242814779,2.64624821059406));
#70027=CARTESIAN_POINT('Ctrl Pts',(18.18,109.334242814779,2.51091407649219));
#70028=CARTESIAN_POINT('Ctrl Pts',(18.18,109.465211504698,2.41869034282863));
#70029=CARTESIAN_POINT('Ctrl Pts',(18.3,109.464665824175,2.8738062273711));
#70030=CARTESIAN_POINT('Ctrl Pts',(18.1272,109.464665824175,2.8738062273711));
#70031=CARTESIAN_POINT('Ctrl Pts',(18.3,109.334242814779,2.78158249370754));
#70032=CARTESIAN_POINT('Ctrl Pts',(18.1272,109.334242814779,2.78158249370754));
#70033=CARTESIAN_POINT('Ctrl Pts',(18.3,109.334242814779,2.64624821059406));
#70034=CARTESIAN_POINT('Ctrl Pts',(18.1272,109.334242814779,2.64624821059406));
#70035=CARTESIAN_POINT('',(18.3,109.464665824175,2.8738062273711));
#70036=CARTESIAN_POINT('Ctrl Pts',(18.3,109.464665824175,2.8738062273711));
#70037=CARTESIAN_POINT('Ctrl Pts',(18.3,109.334242814779,2.78158249370754));
#70038=CARTESIAN_POINT('Ctrl Pts',(18.3,109.334242814779,2.64624821059406));
#70039=CARTESIAN_POINT('',(18.18,109.464665824175,2.8738062273711));
#70040=CARTESIAN_POINT('',(18.3,109.464665824175,2.8738062273711));
#70041=CARTESIAN_POINT('Ctrl Pts',(18.18,109.464665824175,2.8738062273711));
#70042=CARTESIAN_POINT('Ctrl Pts',(18.18,109.334242814779,2.78158249370754));
#70043=CARTESIAN_POINT('Ctrl Pts',(18.18,109.334242814779,2.64624821059406));
#70044=CARTESIAN_POINT('Ctrl Pts',(18.3,109.989085966349,2.96602996103466));
#70045=CARTESIAN_POINT('Ctrl Pts',(18.1272,109.989085966349,2.96602996103466));
#70046=CARTESIAN_POINT('Ctrl Pts',(18.3,109.59508883357,2.96602996103466));
#70047=CARTESIAN_POINT('Ctrl Pts',(18.1272,109.59508883357,2.96602996103466));
#70048=CARTESIAN_POINT('Ctrl Pts',(18.3,109.464665824175,2.8738062273711));
#70049=CARTESIAN_POINT('Ctrl Pts',(18.1272,109.464665824175,2.8738062273711));
#70050=CARTESIAN_POINT('',(18.3,109.989085966349,2.96602996103466));
#70051=CARTESIAN_POINT('Ctrl Pts',(18.3,109.989085966349,2.96602996103466));
#70052=CARTESIAN_POINT('Ctrl Pts',(18.3,109.59508883357,2.96602996103466));
#70053=CARTESIAN_POINT('Ctrl Pts',(18.3,109.464665824175,2.8738062273711));
#70054=CARTESIAN_POINT('',(18.18,109.989085966349,2.96602996103466));
#70055=CARTESIAN_POINT('',(18.3,109.989085966349,2.96602996103466));
#70056=CARTESIAN_POINT('Ctrl Pts',(18.18,109.989085966349,2.96602996103466));
#70057=CARTESIAN_POINT('Ctrl Pts',(18.18,109.59508883357,2.96602996103466));
#70058=CARTESIAN_POINT('Ctrl Pts',(18.18,109.464665824175,2.8738062273711));
#70059=CARTESIAN_POINT('Ctrl Pts',(18.3,110.529331588745,2.86452936045825));
#70060=CARTESIAN_POINT('Ctrl Pts',(18.1272,110.529331588745,2.86452936045825));
#70061=CARTESIAN_POINT('Ctrl Pts',(18.3,110.383083099127,2.96602996103466));
#70062=CARTESIAN_POINT('Ctrl Pts',(18.1272,110.383083099127,2.96602996103466));
#70063=CARTESIAN_POINT('Ctrl Pts',(18.3,109.989085966349,2.96602996103466));
#70064=CARTESIAN_POINT('Ctrl Pts',(18.1272,109.989085966349,2.96602996103466));
#70065=CARTESIAN_POINT('Ctrl Pts',(18.3,110.529331588745,2.86452936045825));
#70066=CARTESIAN_POINT('Ctrl Pts',(18.3,110.383083099127,2.96602996103466));
#70067=CARTESIAN_POINT('Ctrl Pts',(18.3,109.989085966349,2.96602996103466));
#70068=CARTESIAN_POINT('Ctrl Pts',(18.18,110.529331588745,2.86452936045825));
#70069=CARTESIAN_POINT('Ctrl Pts',(18.18,110.383083099127,2.96602996103466));
#70070=CARTESIAN_POINT('Ctrl Pts',(18.18,109.989085966349,2.96602996103466));
#70071=CARTESIAN_POINT('Ctrl Pts',(18.3,109.172714823484,2.64624821059406));
#70072=CARTESIAN_POINT('Ctrl Pts',(18.1272,109.172714823484,2.64624821059406));
#70073=CARTESIAN_POINT('Ctrl Pts',(18.3,109.172714823484,2.87762614004314));
#70074=CARTESIAN_POINT('Ctrl Pts',(18.1272,109.172714823484,2.87762614004314));
#70075=CARTESIAN_POINT('Ctrl Pts',(18.3,109.338608556986,3.00968619100749));
#70076=CARTESIAN_POINT('Ctrl Pts',(18.1272,109.338608556986,3.00968619100749));
#70077=CARTESIAN_POINT('',(18.3,109.172714823484,2.64624821059406));
#70078=CARTESIAN_POINT('',(18.3,109.338608556986,3.00968619100749));
#70079=CARTESIAN_POINT('Ctrl Pts',(18.3,109.172714823484,2.64624821059406));
#70080=CARTESIAN_POINT('Ctrl Pts',(18.3,109.172714823484,2.87762614004314));
#70081=CARTESIAN_POINT('Ctrl Pts',(18.3,109.338608556986,3.00968619100749));
#70082=CARTESIAN_POINT('',(18.18,109.172714823484,2.64624821059406));
#70083=CARTESIAN_POINT('',(18.3,109.172714823484,2.64624821059406));
#70084=CARTESIAN_POINT('',(18.18,109.338608556986,3.00968619100749));
#70085=CARTESIAN_POINT('Ctrl Pts',(18.18,109.172714823484,2.64624821059406));
#70086=CARTESIAN_POINT('Ctrl Pts',(18.18,109.172714823484,2.87762614004314));
#70087=CARTESIAN_POINT('Ctrl Pts',(18.18,109.338608556986,3.00968619100749));
#70088=CARTESIAN_POINT('',(18.3,109.338608556986,3.00968619100749));
#70089=CARTESIAN_POINT('Ctrl Pts',(18.3,109.267121428251,2.35538886897266));
#70090=CARTESIAN_POINT('Ctrl Pts',(18.1272,109.267121428251,2.35538886897266));
#70091=CARTESIAN_POINT('Ctrl Pts',(18.3,109.172714823484,2.47053207866847));
#70092=CARTESIAN_POINT('Ctrl Pts',(18.1272,109.172714823484,2.47053207866847));
#70093=CARTESIAN_POINT('Ctrl Pts',(18.3,109.172714823484,2.64624821059406));
#70094=CARTESIAN_POINT('Ctrl Pts',(18.1272,109.172714823484,2.64624821059406));
#70095=CARTESIAN_POINT('',(18.3,109.267121428251,2.35538886897266));
#70096=CARTESIAN_POINT('Ctrl Pts',(18.3,109.267121428251,2.35538886897266));
#70097=CARTESIAN_POINT('Ctrl Pts',(18.3,109.172714823484,2.47053207866847));
#70098=CARTESIAN_POINT('Ctrl Pts',(18.3,109.172714823484,2.64624821059406));
#70099=CARTESIAN_POINT('',(18.18,109.267121428251,2.35538886897266));
#70100=CARTESIAN_POINT('',(18.3,109.267121428251,2.35538886897266));
#70101=CARTESIAN_POINT('Ctrl Pts',(18.18,109.267121428251,2.35538886897266));
#70102=CARTESIAN_POINT('Ctrl Pts',(18.18,109.172714823484,2.47053207866847));
#70103=CARTESIAN_POINT('Ctrl Pts',(18.18,109.172714823484,2.64624821059406));
#70104=CARTESIAN_POINT('Ctrl Pts',(18.3,109.534515613317,2.18240113966167));
#70105=CARTESIAN_POINT('Ctrl Pts',(18.1272,109.534515613317,2.18240113966167));
#70106=CARTESIAN_POINT('Ctrl Pts',(18.3,109.361528033018,2.24024551026523));
#70107=CARTESIAN_POINT('Ctrl Pts',(18.1272,109.361528033018,2.24024551026523));
#70108=CARTESIAN_POINT('Ctrl Pts',(18.3,109.267121428251,2.35538886897266));
#70109=CARTESIAN_POINT('Ctrl Pts',(18.1272,109.267121428251,2.35538886897266));
#70110=CARTESIAN_POINT('',(18.3,109.534515613317,2.18240113966167));
#70111=CARTESIAN_POINT('Ctrl Pts',(18.3,109.534515613317,2.18240113966167));
#70112=CARTESIAN_POINT('Ctrl Pts',(18.3,109.361528033018,2.24024551026523));
#70113=CARTESIAN_POINT('Ctrl Pts',(18.3,109.267121428251,2.35538886897266));
#70114=CARTESIAN_POINT('',(18.18,109.534515613317,2.18240113966167));
#70115=CARTESIAN_POINT('',(18.3,109.534515613317,2.18240113966167));
#70116=CARTESIAN_POINT('Ctrl Pts',(18.18,109.534515613317,2.18240113966167));
#70117=CARTESIAN_POINT('Ctrl Pts',(18.18,109.361528033018,2.24024551026523));
#70118=CARTESIAN_POINT('Ctrl Pts',(18.18,109.267121428251,2.35538886897266));
#70119=CARTESIAN_POINT('Ctrl Pts',(18.3,109.989085966349,2.12455647103488));
#70120=CARTESIAN_POINT('Ctrl Pts',(18.1272,109.989085966349,2.12455647103488));
#70121=CARTESIAN_POINT('Ctrl Pts',(18.3,109.70750349164,2.12455647103488));
#70122=CARTESIAN_POINT('Ctrl Pts',(18.1272,109.70750349164,2.12455647103488));
#70123=CARTESIAN_POINT('Ctrl Pts',(18.3,109.534515613317,2.18240113966167));
#70124=CARTESIAN_POINT('Ctrl Pts',(18.1272,109.534515613317,2.18240113966167));
#70125=CARTESIAN_POINT('',(18.3,109.989085966349,2.12455647103488));
#70126=CARTESIAN_POINT('Ctrl Pts',(18.3,109.989085966349,2.12455647103488));
#70127=CARTESIAN_POINT('Ctrl Pts',(18.3,109.70750349164,2.12455647103488));
#70128=CARTESIAN_POINT('Ctrl Pts',(18.3,109.534515613317,2.18240113966167));
#70129=CARTESIAN_POINT('',(18.18,109.989085966349,2.12455647103488));
#70130=CARTESIAN_POINT('',(18.3,109.989085966349,2.12455647103488));
#70131=CARTESIAN_POINT('Ctrl Pts',(18.18,109.989085966349,2.12455647103488));
#70132=CARTESIAN_POINT('Ctrl Pts',(18.18,109.70750349164,2.12455647103488));
#70133=CARTESIAN_POINT('Ctrl Pts',(18.18,109.534515613317,2.18240113966167));
#70134=CARTESIAN_POINT('Ctrl Pts',(18.3,110.367257767916,2.16057302467525));
#70135=CARTESIAN_POINT('Ctrl Pts',(18.1272,110.367257767916,2.16057302467525));
#70136=CARTESIAN_POINT('Ctrl Pts',(18.3,110.227012211084,2.12455647103488));
#70137=CARTESIAN_POINT('Ctrl Pts',(18.1272,110.227012211084,2.12455647103488));
#70138=CARTESIAN_POINT('Ctrl Pts',(18.3,109.989085966349,2.12455647103488));
#70139=CARTESIAN_POINT('Ctrl Pts',(18.1272,109.989085966349,2.12455647103488));
#70140=CARTESIAN_POINT('',(18.3,110.367257767916,2.16057302467525));
#70141=CARTESIAN_POINT('Ctrl Pts',(18.3,110.367257767916,2.16057302467525));
#70142=CARTESIAN_POINT('Ctrl Pts',(18.3,110.227012211084,2.12455647103488));
#70143=CARTESIAN_POINT('Ctrl Pts',(18.3,109.989085966349,2.12455647103488));
#70144=CARTESIAN_POINT('',(18.18,110.367257767916,2.16057302467525));
#70145=CARTESIAN_POINT('',(18.3,110.367257767916,2.16057302467525));
#70146=CARTESIAN_POINT('Ctrl Pts',(18.18,110.367257767916,2.16057302467525));
#70147=CARTESIAN_POINT('Ctrl Pts',(18.18,110.227012211084,2.12455647103488));
#70148=CARTESIAN_POINT('Ctrl Pts',(18.18,109.989085966349,2.12455647103488));
#70149=CARTESIAN_POINT('Ctrl Pts',(18.3,110.605184161663,2.25989090315998));
#70150=CARTESIAN_POINT('Ctrl Pts',(18.1272,110.605184161663,2.25989090315998));
#70151=CARTESIAN_POINT('Ctrl Pts',(18.3,110.507503473759,2.19658928029239));
#70152=CARTESIAN_POINT('Ctrl Pts',(18.1272,110.507503473759,2.19658928029239));
#70153=CARTESIAN_POINT('Ctrl Pts',(18.3,110.367257767916,2.16057302467525));
#70154=CARTESIAN_POINT('Ctrl Pts',(18.1272,110.367257767916,2.16057302467525));
#70155=CARTESIAN_POINT('',(18.3,110.605184161663,2.25989090315998));
#70156=CARTESIAN_POINT('Ctrl Pts',(18.3,110.605184161663,2.25989090315998));
#70157=CARTESIAN_POINT('Ctrl Pts',(18.3,110.507503473759,2.19658928029239));
#70158=CARTESIAN_POINT('Ctrl Pts',(18.3,110.367257767916,2.16057302467525));
#70159=CARTESIAN_POINT('',(18.18,110.605184161663,2.25989090315998));
#70160=CARTESIAN_POINT('',(18.3,110.605184161663,2.25989090315998));
#70161=CARTESIAN_POINT('Ctrl Pts',(18.18,110.605184161663,2.25989090315998));
#70162=CARTESIAN_POINT('Ctrl Pts',(18.18,110.507503473759,2.19658928029239));
#70163=CARTESIAN_POINT('Ctrl Pts',(18.18,110.367257767916,2.16057302467525));
#70164=CARTESIAN_POINT('Ctrl Pts',(18.3,110.754706734419,2.420327533409));
#70165=CARTESIAN_POINT('Ctrl Pts',(18.1272,110.754706734419,2.420327533409));
#70166=CARTESIAN_POINT('Ctrl Pts',(18.3,110.702864998579,2.32319237701595));
#70167=CARTESIAN_POINT('Ctrl Pts',(18.1272,110.702864998579,2.32319237701595));
#70168=CARTESIAN_POINT('Ctrl Pts',(18.3,110.605184161663,2.25989090315998));
#70169=CARTESIAN_POINT('Ctrl Pts',(18.1272,110.605184161663,2.25989090315998));
#70170=CARTESIAN_POINT('',(18.3,110.754706734419,2.420327533409));
#70171=CARTESIAN_POINT('Ctrl Pts',(18.3,110.754706734419,2.420327533409));
#70172=CARTESIAN_POINT('Ctrl Pts',(18.3,110.702864998579,2.32319237701595));
#70173=CARTESIAN_POINT('Ctrl Pts',(18.3,110.605184161663,2.25989090315998));
#70174=CARTESIAN_POINT('',(18.18,110.754706734419,2.420327533409));
#70175=CARTESIAN_POINT('',(18.3,110.754706734419,2.420327533409));
#70176=CARTESIAN_POINT('Ctrl Pts',(18.18,110.754706734419,2.420327533409));
#70177=CARTESIAN_POINT('Ctrl Pts',(18.18,110.702864998579,2.32319237701595));
#70178=CARTESIAN_POINT('Ctrl Pts',(18.18,110.605184161663,2.25989090315998));
#70179=CARTESIAN_POINT('Ctrl Pts',(18.3,110.806548470259,2.64624821059406));
#70180=CARTESIAN_POINT('Ctrl Pts',(18.1272,110.806548470259,2.64624821059406));
#70181=CARTESIAN_POINT('Ctrl Pts',(18.3,110.806548470259,2.51746254079044));
#70182=CARTESIAN_POINT('Ctrl Pts',(18.1272,110.806548470259,2.51746254079044));
#70183=CARTESIAN_POINT('Ctrl Pts',(18.3,110.754706734419,2.420327533409));
#70184=CARTESIAN_POINT('Ctrl Pts',(18.1272,110.754706734419,2.420327533409));
#70185=CARTESIAN_POINT('',(18.3,110.806548470259,2.64624821059406));
#70186=CARTESIAN_POINT('Ctrl Pts',(18.3,110.806548470259,2.64624821059406));
#70187=CARTESIAN_POINT('Ctrl Pts',(18.3,110.806548470259,2.51746254079044));
#70188=CARTESIAN_POINT('Ctrl Pts',(18.3,110.754706734419,2.420327533409));
#70189=CARTESIAN_POINT('',(18.18,110.806548470259,2.64624821059406));
#70190=CARTESIAN_POINT('',(18.3,110.806548470259,2.64624821059406));
#70191=CARTESIAN_POINT('Ctrl Pts',(18.18,110.806548470259,2.64624821059406));
#70192=CARTESIAN_POINT('Ctrl Pts',(18.18,110.806548470259,2.51746254079044));
#70193=CARTESIAN_POINT('Ctrl Pts',(18.18,110.754706734419,2.420327533409));
#70194=CARTESIAN_POINT('Ctrl Pts',(18.3,110.712687695026,2.93601634018123));
#70195=CARTESIAN_POINT('Ctrl Pts',(18.1272,110.712687695026,2.93601634018123));
#70196=CARTESIAN_POINT('Ctrl Pts',(18.3,110.806548470259,2.82087313048542));
#70197=CARTESIAN_POINT('Ctrl Pts',(18.1272,110.806548470259,2.82087313048542));
#70198=CARTESIAN_POINT('Ctrl Pts',(18.3,110.806548470259,2.64624821059406));
#70199=CARTESIAN_POINT('Ctrl Pts',(18.1272,110.806548470259,2.64624821059406));
#70200=CARTESIAN_POINT('',(18.3,110.712687695026,2.93601634018123));
#70201=CARTESIAN_POINT('Ctrl Pts',(18.3,110.712687695026,2.93601634018123));
#70202=CARTESIAN_POINT('Ctrl Pts',(18.3,110.806548470259,2.82087313048542));
#70203=CARTESIAN_POINT('Ctrl Pts',(18.3,110.806548470259,2.64624821059406));
#70204=CARTESIAN_POINT('',(18.18,110.712687695026,2.93601634018123));
#70205=CARTESIAN_POINT('',(18.3,110.712687695026,2.93601634018123));
#70206=CARTESIAN_POINT('Ctrl Pts',(18.18,110.712687695026,2.93601634018123));
#70207=CARTESIAN_POINT('Ctrl Pts',(18.18,110.806548470259,2.82087313048542));
#70208=CARTESIAN_POINT('Ctrl Pts',(18.18,110.806548470259,2.64624821059406));
#70209=CARTESIAN_POINT('Ctrl Pts',(18.3,110.445839041471,3.10954975001514));
#70210=CARTESIAN_POINT('Ctrl Pts',(18.1272,110.445839041471,3.10954975001514));
#70211=CARTESIAN_POINT('Ctrl Pts',(18.3,110.618826770782,3.05115954987705));
#70212=CARTESIAN_POINT('Ctrl Pts',(18.1272,110.618826770782,3.05115954987705));
#70213=CARTESIAN_POINT('Ctrl Pts',(18.3,110.712687695026,2.93601634018123));
#70214=CARTESIAN_POINT('Ctrl Pts',(18.1272,110.712687695026,2.93601634018123));
#70215=CARTESIAN_POINT('',(18.3,110.445839041471,3.10954975001514));
#70216=CARTESIAN_POINT('Ctrl Pts',(18.3,110.445839041471,3.10954975001514));
#70217=CARTESIAN_POINT('Ctrl Pts',(18.3,110.618826770782,3.05115954987705));
#70218=CARTESIAN_POINT('Ctrl Pts',(18.3,110.712687695026,2.93601634018123));
#70219=CARTESIAN_POINT('',(18.18,110.445839041471,3.10954975001514));
#70220=CARTESIAN_POINT('',(18.3,110.445839041471,3.10954975001514));
#70221=CARTESIAN_POINT('Ctrl Pts',(18.18,110.445839041471,3.10954975001514));
#70222=CARTESIAN_POINT('Ctrl Pts',(18.18,110.618826770782,3.05115954987705));
#70223=CARTESIAN_POINT('Ctrl Pts',(18.18,110.712687695026,2.93601634018123));
#70224=CARTESIAN_POINT('Ctrl Pts',(18.3,109.989085966349,3.16793995015323));
#70225=CARTESIAN_POINT('Ctrl Pts',(18.1272,109.989085966349,3.16793995015323));
#70226=CARTESIAN_POINT('Ctrl Pts',(18.3,110.27285131216,3.16793995015323));
#70227=CARTESIAN_POINT('Ctrl Pts',(18.1272,110.27285131216,3.16793995015323));
#70228=CARTESIAN_POINT('Ctrl Pts',(18.3,110.445839041471,3.10954975001514));
#70229=CARTESIAN_POINT('Ctrl Pts',(18.1272,110.445839041471,3.10954975001514));
#70230=CARTESIAN_POINT('',(18.3,109.989085966349,3.16793995015323));
#70231=CARTESIAN_POINT('Ctrl Pts',(18.3,109.989085966349,3.16793995015323));
#70232=CARTESIAN_POINT('Ctrl Pts',(18.3,110.27285131216,3.16793995015323));
#70233=CARTESIAN_POINT('Ctrl Pts',(18.3,110.445839041471,3.10954975001514));
#70234=CARTESIAN_POINT('',(18.18,109.989085966349,3.16793995015323));
#70235=CARTESIAN_POINT('',(18.3,109.989085966349,3.16793995015323));
#70236=CARTESIAN_POINT('Ctrl Pts',(18.18,109.989085966349,3.16793995015323));
#70237=CARTESIAN_POINT('Ctrl Pts',(18.18,110.27285131216,3.16793995015323));
#70238=CARTESIAN_POINT('Ctrl Pts',(18.18,110.445839041471,3.10954975001514));
#70239=CARTESIAN_POINT('Ctrl Pts',(18.3,109.338608556986,3.00968619100749));
#70240=CARTESIAN_POINT('Ctrl Pts',(18.1272,109.338608556986,3.00968619100749));
#70241=CARTESIAN_POINT('Ctrl Pts',(18.3,109.538335675001,3.16793995015323));
#70242=CARTESIAN_POINT('Ctrl Pts',(18.1272,109.538335675001,3.16793995015323));
#70243=CARTESIAN_POINT('Ctrl Pts',(18.3,109.989085966349,3.16793995015323));
#70244=CARTESIAN_POINT('Ctrl Pts',(18.1272,109.989085966349,3.16793995015323));
#70245=CARTESIAN_POINT('Ctrl Pts',(18.3,109.338608556986,3.00968619100749));
#70246=CARTESIAN_POINT('Ctrl Pts',(18.3,109.538335675001,3.16793995015323));
#70247=CARTESIAN_POINT('Ctrl Pts',(18.3,109.989085966349,3.16793995015323));
#70248=CARTESIAN_POINT('Ctrl Pts',(18.18,109.338608556986,3.00968619100749));
#70249=CARTESIAN_POINT('Ctrl Pts',(18.18,109.538335675001,3.16793995015323));
#70250=CARTESIAN_POINT('Ctrl Pts',(18.18,109.989085966349,3.16793995015323));
#70251=CARTESIAN_POINT('Origin',(18.18,109.989631646872,3.29999987538904));
#70252=CARTESIAN_POINT('Origin',(18.3,110.484583848715,3.78130966834724));
#70253=CARTESIAN_POINT('',(18.3,110.484583848715,3.78130966834724));
#70254=CARTESIAN_POINT('',(18.3,109.76316499114,4.28226457946002));
#70255=CARTESIAN_POINT('',(18.3,96.4250103615061,13.5443097793353));
#70256=CARTESIAN_POINT('',(18.18,110.484583848715,3.78130966834724));
#70257=CARTESIAN_POINT('',(18.3,110.484583848715,3.78130966834724));
#70258=CARTESIAN_POINT('',(18.18,109.76316499114,4.28226457946002));
#70259=CARTESIAN_POINT('',(18.18,110.484583848715,3.78130966834724));
#70260=CARTESIAN_POINT('',(18.3,109.76316499114,4.28226457946002));
#70261=CARTESIAN_POINT('Origin',(18.3,109.76316499114,3.78130966834724));
#70262=CARTESIAN_POINT('',(18.3,109.76316499114,3.78130966834724));
#70263=CARTESIAN_POINT('',(18.3,89.8815824955702,3.78130966834724));
#70264=CARTESIAN_POINT('',(18.18,109.76316499114,3.78130966834724));
#70265=CARTESIAN_POINT('',(18.3,109.76316499114,3.78130966834724));
#70266=CARTESIAN_POINT('',(18.18,109.76316499114,3.78130966834724));
#70267=CARTESIAN_POINT('Origin',(18.3,109.76316499114,4.28226457946002));
#70268=CARTESIAN_POINT('',(18.3,109.76316499114,4.89113228973001));
#70269=CARTESIAN_POINT('',(18.18,109.76316499114,4.28226457946002));
#70270=CARTESIAN_POINT('Origin',(18.3,109.58308326602,3.58485670797527));
#70271=CARTESIAN_POINT('',(18.3,109.58308326602,3.58485670797527));
#70272=CARTESIAN_POINT('',(18.3,109.200000041723,3.58485670797527));
#70273=CARTESIAN_POINT('',(18.3,89.7915416330099,3.58485670797527));
#70274=CARTESIAN_POINT('',(18.18,109.58308326602,3.58485670797527));
#70275=CARTESIAN_POINT('',(18.3,109.58308326602,3.58485670797527));
#70276=CARTESIAN_POINT('',(18.18,109.200000041723,3.58485670797527));
#70277=CARTESIAN_POINT('',(18.18,109.58308326602,3.58485670797527));
#70278=CARTESIAN_POINT('',(18.3,109.200000041723,3.58485670797527));
#70279=CARTESIAN_POINT('Origin',(18.3,109.58308326602,3.36875842921436));
#70280=CARTESIAN_POINT('',(18.3,109.58308326602,3.36875842921436));
#70281=CARTESIAN_POINT('',(18.3,109.58308326602,4.43437921460718));
#70282=CARTESIAN_POINT('',(18.18,109.58308326602,3.36875842921436));
#70283=CARTESIAN_POINT('',(18.3,109.58308326602,3.36875842921436));
#70284=CARTESIAN_POINT('',(18.18,109.58308326602,3.36875842921436));
#70285=CARTESIAN_POINT('Origin',(18.3,109.76316499114,3.36875842921436));
#70286=CARTESIAN_POINT('',(18.3,109.76316499114,3.36875842921436));
#70287=CARTESIAN_POINT('',(18.3,89.8815824955702,3.36875842921436));
#70288=CARTESIAN_POINT('',(18.18,109.76316499114,3.36875842921436));
#70289=CARTESIAN_POINT('',(18.3,109.76316499114,3.36875842921436));
#70290=CARTESIAN_POINT('',(18.18,109.76316499114,3.36875842921436));
#70291=CARTESIAN_POINT('Origin',(18.3,109.76316499114,3.58485670797527));
#70292=CARTESIAN_POINT('',(18.3,109.76316499114,3.58485670797527));
#70293=CARTESIAN_POINT('',(18.3,109.76316499114,4.54242835398763));
#70294=CARTESIAN_POINT('',(18.18,109.76316499114,3.58485670797527));
#70295=CARTESIAN_POINT('',(18.3,109.76316499114,3.58485670797527));
#70296=CARTESIAN_POINT('',(18.18,109.76316499114,3.58485670797527));
#70297=CARTESIAN_POINT('Origin',(18.3,110.80000000596,3.58485670797527));
#70298=CARTESIAN_POINT('',(18.3,110.80000000596,3.58485670797527));
#70299=CARTESIAN_POINT('',(18.3,90.4000000029802,3.58485670797527));
#70300=CARTESIAN_POINT('',(18.18,110.80000000596,3.58485670797527));
#70301=CARTESIAN_POINT('',(18.3,110.80000000596,3.58485670797527));
#70302=CARTESIAN_POINT('',(18.18,110.80000000596,3.58485670797527));
#70303=CARTESIAN_POINT('Origin',(18.3,110.80000000596,3.74529326371849));
#70304=CARTESIAN_POINT('',(18.3,110.80000000596,3.74529326371849));
#70305=CARTESIAN_POINT('',(18.3,110.80000000596,4.62264663185924));
#70306=CARTESIAN_POINT('',(18.18,110.80000000596,3.74529326371849));
#70307=CARTESIAN_POINT('',(18.3,110.80000000596,3.74529326371849));
#70308=CARTESIAN_POINT('',(18.18,110.80000000596,3.74529326371849));
#70309=CARTESIAN_POINT('Origin',(18.3,109.76316499114,4.47544327974319));
#70310=CARTESIAN_POINT('',(18.3,109.76316499114,4.47544327974319));
#70311=CARTESIAN_POINT('',(18.3,96.2313997020141,14.0046533290512));
#70312=CARTESIAN_POINT('',(18.18,109.76316499114,4.47544327974319));
#70313=CARTESIAN_POINT('',(18.3,109.76316499114,4.47544327974319));
#70314=CARTESIAN_POINT('',(18.18,109.76316499114,4.47544327974319));
#70315=CARTESIAN_POINT('Origin',(18.3,109.58308326602,4.47544327974319));
#70316=CARTESIAN_POINT('',(18.3,109.58308326602,4.47544327974319));
#70317=CARTESIAN_POINT('',(18.3,89.7915416330099,4.47544327974319));
#70318=CARTESIAN_POINT('',(18.18,109.58308326602,4.47544327974319));
#70319=CARTESIAN_POINT('',(18.3,109.58308326602,4.47544327974319));
#70320=CARTESIAN_POINT('',(18.18,109.58308326602,4.47544327974319));
#70321=CARTESIAN_POINT('Origin',(18.3,109.58308326602,3.78130966834724));
#70322=CARTESIAN_POINT('',(18.3,109.58308326602,3.78130966834724));
#70323=CARTESIAN_POINT('',(18.3,109.58308326602,4.64065483417362));
#70324=CARTESIAN_POINT('',(18.18,109.58308326602,3.78130966834724));
#70325=CARTESIAN_POINT('',(18.3,109.58308326602,3.78130966834724));
#70326=CARTESIAN_POINT('',(18.18,109.58308326602,3.78130966834724));
#70327=CARTESIAN_POINT('Origin',(18.3,109.200000041723,3.78130966834724));
#70328=CARTESIAN_POINT('',(18.3,109.200000041723,3.78130966834724));
#70329=CARTESIAN_POINT('',(18.3,89.6000000208616,3.78130966834724));
#70330=CARTESIAN_POINT('',(18.18,109.200000041723,3.78130966834724));
#70331=CARTESIAN_POINT('',(18.3,109.200000041723,3.78130966834724));
#70332=CARTESIAN_POINT('',(18.18,109.200000041723,3.78130966834724));
#70333=CARTESIAN_POINT('Origin',(18.3,109.200000041723,3.58485670797527));
#70334=CARTESIAN_POINT('',(18.3,109.200000041723,4.54242835398763));
#70335=CARTESIAN_POINT('',(18.18,109.200000041723,3.58485670797527));
#70336=CARTESIAN_POINT('Origin',(18.18,109.989631646872,3.29999987538904));
#70337=CARTESIAN_POINT('Origin',(18.3,70.,5.5));
#70338=CARTESIAN_POINT('Origin',(18.3,70.,5.5));
#70339=CARTESIAN_POINT('Ctrl Pts',(18.3,100.643929117918,2.68117321692407));
#70340=CARTESIAN_POINT('Ctrl Pts',(18.1272,100.643929117918,2.68117321692407));
#70341=CARTESIAN_POINT('Ctrl Pts',(18.3,100.643929117918,2.81650750003755));
#70342=CARTESIAN_POINT('Ctrl Pts',(18.1272,100.643929117918,2.81650750003755));
#70343=CARTESIAN_POINT('Ctrl Pts',(18.3,100.529331588745,2.89727149568498));
#70344=CARTESIAN_POINT('Ctrl Pts',(18.1272,100.529331588745,2.89727149568498));
#70345=CARTESIAN_POINT('',(18.3,100.643929117918,2.68117321692407));
#70346=CARTESIAN_POINT('',(18.3,100.529331588745,2.89727149568498));
#70347=CARTESIAN_POINT('Ctrl Pts',(18.3,100.643929117918,2.68117321692407));
#70348=CARTESIAN_POINT('Ctrl Pts',(18.3,100.643929117918,2.81650750003755));
#70349=CARTESIAN_POINT('Ctrl Pts',(18.3,100.529331588745,2.89727149568498));
#70350=CARTESIAN_POINT('',(18.18,100.643929117918,2.68117321692407));
#70351=CARTESIAN_POINT('',(18.3,100.643929117918,2.68117321692407));
#70352=CARTESIAN_POINT('',(18.18,100.529331588745,2.89727149568498));
#70353=CARTESIAN_POINT('Ctrl Pts',(18.18,100.643929117918,2.68117321692407));
#70354=CARTESIAN_POINT('Ctrl Pts',(18.18,100.643929117918,2.81650750003755));
#70355=CARTESIAN_POINT('Ctrl Pts',(18.18,100.529331588745,2.89727149568498));
#70356=CARTESIAN_POINT('',(18.3,100.529331588745,2.89727149568498));
#70357=CARTESIAN_POINT('Ctrl Pts',(18.3,100.514051938057,2.45143247805536));
#70358=CARTESIAN_POINT('Ctrl Pts',(18.1272,100.514051938057,2.45143247805536));
#70359=CARTESIAN_POINT('Ctrl Pts',(18.3,100.643929117918,2.54365621171892));
#70360=CARTESIAN_POINT('Ctrl Pts',(18.1272,100.643929117918,2.54365621171892));
#70361=CARTESIAN_POINT('Ctrl Pts',(18.3,100.643929117918,2.68117321692407));
#70362=CARTESIAN_POINT('Ctrl Pts',(18.1272,100.643929117918,2.68117321692407));
#70363=CARTESIAN_POINT('',(18.3,100.514051938057,2.45143247805536));
#70364=CARTESIAN_POINT('Ctrl Pts',(18.3,100.514051938057,2.45143247805536));
#70365=CARTESIAN_POINT('Ctrl Pts',(18.3,100.643929117918,2.54365621171892));
#70366=CARTESIAN_POINT('Ctrl Pts',(18.3,100.643929117918,2.68117321692407));
#70367=CARTESIAN_POINT('',(18.18,100.514051938057,2.45143247805536));
#70368=CARTESIAN_POINT('',(18.3,100.514051938057,2.45143247805536));
#70369=CARTESIAN_POINT('Ctrl Pts',(18.18,100.514051938057,2.45143247805536));
#70370=CARTESIAN_POINT('Ctrl Pts',(18.18,100.643929117918,2.54365621171892));
#70371=CARTESIAN_POINT('Ctrl Pts',(18.18,100.643929117918,2.68117321692407));
#70372=CARTESIAN_POINT('Ctrl Pts',(18.3,99.9890859663486,2.3592087443918));
#70373=CARTESIAN_POINT('Ctrl Pts',(18.1272,99.9890859663486,2.3592087443918));
#70374=CARTESIAN_POINT('Ctrl Pts',(18.3,100.384174609184,2.3592087443918));
#70375=CARTESIAN_POINT('Ctrl Pts',(18.1272,100.384174609184,2.3592087443918));
#70376=CARTESIAN_POINT('Ctrl Pts',(18.3,100.514051938057,2.45143247805536));
#70377=CARTESIAN_POINT('Ctrl Pts',(18.1272,100.514051938057,2.45143247805536));
#70378=CARTESIAN_POINT('',(18.3,99.9890859663486,2.3592087443918));
#70379=CARTESIAN_POINT('Ctrl Pts',(18.3,99.9890859663486,2.3592087443918));
#70380=CARTESIAN_POINT('Ctrl Pts',(18.3,100.384174609184,2.3592087443918));
#70381=CARTESIAN_POINT('Ctrl Pts',(18.3,100.514051938057,2.45143247805536));
#70382=CARTESIAN_POINT('',(18.18,99.9890859663486,2.3592087443918));
#70383=CARTESIAN_POINT('',(18.3,99.9890859663486,2.3592087443918));
#70384=CARTESIAN_POINT('Ctrl Pts',(18.18,99.9890859663486,2.3592087443918));
#70385=CARTESIAN_POINT('Ctrl Pts',(18.18,100.384174609184,2.3592087443918));
#70386=CARTESIAN_POINT('Ctrl Pts',(18.18,100.514051938057,2.45143247805536));
#70387=CARTESIAN_POINT('Ctrl Pts',(18.3,99.4652115046978,2.45143247805536));
#70388=CARTESIAN_POINT('Ctrl Pts',(18.1272,99.4652115046978,2.45143247805536));
#70389=CARTESIAN_POINT('Ctrl Pts',(18.3,99.5961801946163,2.3592087443918));
#70390=CARTESIAN_POINT('Ctrl Pts',(18.1272,99.5961801946163,2.3592087443918));
#70391=CARTESIAN_POINT('Ctrl Pts',(18.3,99.9890859663486,2.3592087443918));
#70392=CARTESIAN_POINT('Ctrl Pts',(18.1272,99.9890859663486,2.3592087443918));
#70393=CARTESIAN_POINT('',(18.3,99.4652115046978,2.45143247805536));
#70394=CARTESIAN_POINT('Ctrl Pts',(18.3,99.4652115046978,2.45143247805536));
#70395=CARTESIAN_POINT('Ctrl Pts',(18.3,99.5961801946163,2.3592087443918));
#70396=CARTESIAN_POINT('Ctrl Pts',(18.3,99.9890859663486,2.3592087443918));
#70397=CARTESIAN_POINT('',(18.18,99.4652115046978,2.45143247805536));
#70398=CARTESIAN_POINT('',(18.3,99.4652115046978,2.45143247805536));
#70399=CARTESIAN_POINT('Ctrl Pts',(18.18,99.4652115046978,2.45143247805536));
#70400=CARTESIAN_POINT('Ctrl Pts',(18.18,99.5961801946163,2.3592087443918));
#70401=CARTESIAN_POINT('Ctrl Pts',(18.18,99.9890859663486,2.3592087443918));
#70402=CARTESIAN_POINT('Ctrl Pts',(18.3,99.3342428147793,2.67899034582078));
#70403=CARTESIAN_POINT('Ctrl Pts',(18.1272,99.3342428147793,2.67899034582078));
#70404=CARTESIAN_POINT('Ctrl Pts',(18.3,99.3342428147793,2.54365621171892));
#70405=CARTESIAN_POINT('Ctrl Pts',(18.1272,99.3342428147793,2.54365621171892));
#70406=CARTESIAN_POINT('Ctrl Pts',(18.3,99.4652115046978,2.45143247805536));
#70407=CARTESIAN_POINT('Ctrl Pts',(18.1272,99.4652115046978,2.45143247805536));
#70408=CARTESIAN_POINT('',(18.3,99.3342428147793,2.67899034582078));
#70409=CARTESIAN_POINT('Ctrl Pts',(18.3,99.3342428147793,2.67899034582078));
#70410=CARTESIAN_POINT('Ctrl Pts',(18.3,99.3342428147793,2.54365621171892));
#70411=CARTESIAN_POINT('Ctrl Pts',(18.3,99.4652115046978,2.45143247805536));
#70412=CARTESIAN_POINT('',(18.18,99.3342428147793,2.67899034582078));
#70413=CARTESIAN_POINT('',(18.3,99.3342428147793,2.67899034582078));
#70414=CARTESIAN_POINT('Ctrl Pts',(18.18,99.3342428147793,2.67899034582078));
#70415=CARTESIAN_POINT('Ctrl Pts',(18.18,99.3342428147793,2.54365621171892));
#70416=CARTESIAN_POINT('Ctrl Pts',(18.18,99.4652115046978,2.45143247805536));
#70417=CARTESIAN_POINT('Ctrl Pts',(18.3,99.4646658241749,2.90654836259782));
#70418=CARTESIAN_POINT('Ctrl Pts',(18.1272,99.4646658241749,2.90654836259782));
#70419=CARTESIAN_POINT('Ctrl Pts',(18.3,99.3342428147793,2.81432462893426));
#70420=CARTESIAN_POINT('Ctrl Pts',(18.1272,99.3342428147793,2.81432462893426));
#70421=CARTESIAN_POINT('Ctrl Pts',(18.3,99.3342428147793,2.67899034582078));
#70422=CARTESIAN_POINT('Ctrl Pts',(18.1272,99.3342428147793,2.67899034582078));
#70423=CARTESIAN_POINT('',(18.3,99.4646658241749,2.90654836259782));
#70424=CARTESIAN_POINT('Ctrl Pts',(18.3,99.4646658241749,2.90654836259782));
#70425=CARTESIAN_POINT('Ctrl Pts',(18.3,99.3342428147793,2.81432462893426));
#70426=CARTESIAN_POINT('Ctrl Pts',(18.3,99.3342428147793,2.67899034582078));
#70427=CARTESIAN_POINT('',(18.18,99.4646658241749,2.90654836259782));
#70428=CARTESIAN_POINT('',(18.3,99.4646658241749,2.90654836259782));
#70429=CARTESIAN_POINT('Ctrl Pts',(18.18,99.4646658241749,2.90654836259782));
#70430=CARTESIAN_POINT('Ctrl Pts',(18.18,99.3342428147793,2.81432462893426));
#70431=CARTESIAN_POINT('Ctrl Pts',(18.18,99.3342428147793,2.67899034582078));
#70432=CARTESIAN_POINT('Ctrl Pts',(18.3,99.9890859663486,2.99877209626138));
#70433=CARTESIAN_POINT('Ctrl Pts',(18.1272,99.9890859663486,2.99877209626138));
#70434=CARTESIAN_POINT('Ctrl Pts',(18.3,99.5950888335705,2.99877209626138));
#70435=CARTESIAN_POINT('Ctrl Pts',(18.1272,99.5950888335705,2.99877209626138));
#70436=CARTESIAN_POINT('Ctrl Pts',(18.3,99.4646658241749,2.90654836259782));
#70437=CARTESIAN_POINT('Ctrl Pts',(18.1272,99.4646658241749,2.90654836259782));
#70438=CARTESIAN_POINT('',(18.3,99.9890859663486,2.99877209626138));
#70439=CARTESIAN_POINT('Ctrl Pts',(18.3,99.9890859663486,2.99877209626138));
#70440=CARTESIAN_POINT('Ctrl Pts',(18.3,99.5950888335705,2.99877209626138));
#70441=CARTESIAN_POINT('Ctrl Pts',(18.3,99.4646658241749,2.90654836259782));
#70442=CARTESIAN_POINT('',(18.18,99.9890859663486,2.99877209626138));
#70443=CARTESIAN_POINT('',(18.3,99.9890859663486,2.99877209626138));
#70444=CARTESIAN_POINT('Ctrl Pts',(18.18,99.9890859663486,2.99877209626138));
#70445=CARTESIAN_POINT('Ctrl Pts',(18.18,99.5950888335705,2.99877209626138));
#70446=CARTESIAN_POINT('Ctrl Pts',(18.18,99.4646658241749,2.90654836259782));
#70447=CARTESIAN_POINT('Ctrl Pts',(18.3,100.529331588745,2.89727149568498));
#70448=CARTESIAN_POINT('Ctrl Pts',(18.1272,100.529331588745,2.89727149568498));
#70449=CARTESIAN_POINT('Ctrl Pts',(18.3,100.383083099127,2.99877209626138));
#70450=CARTESIAN_POINT('Ctrl Pts',(18.1272,100.383083099127,2.99877209626138));
#70451=CARTESIAN_POINT('Ctrl Pts',(18.3,99.9890859663486,2.99877209626138));
#70452=CARTESIAN_POINT('Ctrl Pts',(18.1272,99.9890859663486,2.99877209626138));
#70453=CARTESIAN_POINT('Ctrl Pts',(18.3,100.529331588745,2.89727149568498));
#70454=CARTESIAN_POINT('Ctrl Pts',(18.3,100.383083099127,2.99877209626138));
#70455=CARTESIAN_POINT('Ctrl Pts',(18.3,99.9890859663486,2.99877209626138));
#70456=CARTESIAN_POINT('Ctrl Pts',(18.18,100.529331588745,2.89727149568498));
#70457=CARTESIAN_POINT('Ctrl Pts',(18.18,100.383083099127,2.99877209626138));
#70458=CARTESIAN_POINT('Ctrl Pts',(18.18,99.9890859663486,2.99877209626138));
#70459=CARTESIAN_POINT('Ctrl Pts',(18.3,99.1727148234844,2.67899034582078));
#70460=CARTESIAN_POINT('Ctrl Pts',(18.1272,99.1727148234844,2.67899034582078));
#70461=CARTESIAN_POINT('Ctrl Pts',(18.3,99.1727148234844,2.91036827526987));
#70462=CARTESIAN_POINT('Ctrl Pts',(18.1272,99.1727148234844,2.91036827526987));
#70463=CARTESIAN_POINT('Ctrl Pts',(18.3,99.3386085569858,3.04242832623422));
#70464=CARTESIAN_POINT('Ctrl Pts',(18.1272,99.3386085569858,3.04242832623422));
#70465=CARTESIAN_POINT('',(18.3,99.1727148234844,2.67899034582078));
#70466=CARTESIAN_POINT('',(18.3,99.3386085569858,3.04242832623422));
#70467=CARTESIAN_POINT('Ctrl Pts',(18.3,99.1727148234844,2.67899034582078));
#70468=CARTESIAN_POINT('Ctrl Pts',(18.3,99.1727148234844,2.91036827526987));
#70469=CARTESIAN_POINT('Ctrl Pts',(18.3,99.3386085569858,3.04242832623422));
#70470=CARTESIAN_POINT('',(18.18,99.1727148234844,2.67899034582078));
#70471=CARTESIAN_POINT('',(18.3,99.1727148234844,2.67899034582078));
#70472=CARTESIAN_POINT('',(18.18,99.3386085569858,3.04242832623422));
#70473=CARTESIAN_POINT('Ctrl Pts',(18.18,99.1727148234844,2.67899034582078));
#70474=CARTESIAN_POINT('Ctrl Pts',(18.18,99.1727148234844,2.91036827526987));
#70475=CARTESIAN_POINT('Ctrl Pts',(18.18,99.3386085569858,3.04242832623422));
#70476=CARTESIAN_POINT('',(18.3,99.3386085569858,3.04242832623422));
#70477=CARTESIAN_POINT('Ctrl Pts',(18.3,99.2671214282513,2.38813100419939));
#70478=CARTESIAN_POINT('Ctrl Pts',(18.1272,99.2671214282513,2.38813100419939));
#70479=CARTESIAN_POINT('Ctrl Pts',(18.3,99.1727148234844,2.5032742138952));
#70480=CARTESIAN_POINT('Ctrl Pts',(18.1272,99.1727148234844,2.5032742138952));
#70481=CARTESIAN_POINT('Ctrl Pts',(18.3,99.1727148234844,2.67899034582078));
#70482=CARTESIAN_POINT('Ctrl Pts',(18.1272,99.1727148234844,2.67899034582078));
#70483=CARTESIAN_POINT('',(18.3,99.2671214282513,2.38813100419939));
#70484=CARTESIAN_POINT('Ctrl Pts',(18.3,99.2671214282513,2.38813100419939));
#70485=CARTESIAN_POINT('Ctrl Pts',(18.3,99.1727148234844,2.5032742138952));
#70486=CARTESIAN_POINT('Ctrl Pts',(18.3,99.1727148234844,2.67899034582078));
#70487=CARTESIAN_POINT('',(18.18,99.2671214282513,2.38813100419939));
#70488=CARTESIAN_POINT('',(18.3,99.2671214282513,2.38813100419939));
#70489=CARTESIAN_POINT('Ctrl Pts',(18.18,99.2671214282513,2.38813100419939));
#70490=CARTESIAN_POINT('Ctrl Pts',(18.18,99.1727148234844,2.5032742138952));
#70491=CARTESIAN_POINT('Ctrl Pts',(18.18,99.1727148234844,2.67899034582078));
#70492=CARTESIAN_POINT('Ctrl Pts',(18.3,99.5345156133175,2.2151432748884));
#70493=CARTESIAN_POINT('Ctrl Pts',(18.1272,99.5345156133175,2.2151432748884));
#70494=CARTESIAN_POINT('Ctrl Pts',(18.3,99.3615280330181,2.27298764549196));
#70495=CARTESIAN_POINT('Ctrl Pts',(18.1272,99.3615280330181,2.27298764549196));
#70496=CARTESIAN_POINT('Ctrl Pts',(18.3,99.2671214282513,2.38813100419939));
#70497=CARTESIAN_POINT('Ctrl Pts',(18.1272,99.2671214282513,2.38813100419939));
#70498=CARTESIAN_POINT('',(18.3,99.5345156133175,2.2151432748884));
#70499=CARTESIAN_POINT('Ctrl Pts',(18.3,99.5345156133175,2.2151432748884));
#70500=CARTESIAN_POINT('Ctrl Pts',(18.3,99.3615280330181,2.27298764549196));
#70501=CARTESIAN_POINT('Ctrl Pts',(18.3,99.2671214282513,2.38813100419939));
#70502=CARTESIAN_POINT('',(18.18,99.5345156133175,2.2151432748884));
#70503=CARTESIAN_POINT('',(18.3,99.5345156133175,2.2151432748884));
#70504=CARTESIAN_POINT('Ctrl Pts',(18.18,99.5345156133175,2.2151432748884));
#70505=CARTESIAN_POINT('Ctrl Pts',(18.18,99.3615280330181,2.27298764549196));
#70506=CARTESIAN_POINT('Ctrl Pts',(18.18,99.2671214282513,2.38813100419939));
#70507=CARTESIAN_POINT('Ctrl Pts',(18.3,99.9890859663486,2.15729875527322));
#70508=CARTESIAN_POINT('Ctrl Pts',(18.1272,99.9890859663486,2.15729875527322));
#70509=CARTESIAN_POINT('Ctrl Pts',(18.3,99.7075034916401,2.15729875527322));
#70510=CARTESIAN_POINT('Ctrl Pts',(18.1272,99.7075034916401,2.15729875527322));
#70511=CARTESIAN_POINT('Ctrl Pts',(18.3,99.5345156133175,2.2151432748884));
#70512=CARTESIAN_POINT('Ctrl Pts',(18.1272,99.5345156133175,2.2151432748884));
#70513=CARTESIAN_POINT('',(18.3,99.9890859663486,2.15729875527322));
#70514=CARTESIAN_POINT('Ctrl Pts',(18.3,99.9890859663486,2.15729875527322));
#70515=CARTESIAN_POINT('Ctrl Pts',(18.3,99.7075034916401,2.15729875527322));
#70516=CARTESIAN_POINT('Ctrl Pts',(18.3,99.5345156133175,2.2151432748884));
#70517=CARTESIAN_POINT('',(18.18,99.9890859663486,2.15729875527322));
#70518=CARTESIAN_POINT('',(18.3,99.9890859663486,2.15729875527322));
#70519=CARTESIAN_POINT('Ctrl Pts',(18.18,99.9890859663486,2.15729875527322));
#70520=CARTESIAN_POINT('Ctrl Pts',(18.18,99.7075034916401,2.15729875527322));
#70521=CARTESIAN_POINT('Ctrl Pts',(18.18,99.5345156133175,2.2151432748884));
#70522=CARTESIAN_POINT('Ctrl Pts',(18.3,100.367257767916,2.19331515990198));
#70523=CARTESIAN_POINT('Ctrl Pts',(18.1272,100.367257767916,2.19331515990198));
#70524=CARTESIAN_POINT('Ctrl Pts',(18.3,100.227012211084,2.15729875527322));
#70525=CARTESIAN_POINT('Ctrl Pts',(18.1272,100.227012211084,2.15729875527322));
#70526=CARTESIAN_POINT('Ctrl Pts',(18.3,99.9890859663486,2.15729875527322));
#70527=CARTESIAN_POINT('Ctrl Pts',(18.1272,99.9890859663486,2.15729875527322));
#70528=CARTESIAN_POINT('',(18.3,100.367257767916,2.19331515990198));
#70529=CARTESIAN_POINT('Ctrl Pts',(18.3,100.367257767916,2.19331515990198));
#70530=CARTESIAN_POINT('Ctrl Pts',(18.3,100.227012211084,2.15729875527322));
#70531=CARTESIAN_POINT('Ctrl Pts',(18.3,99.9890859663486,2.15729875527322));
#70532=CARTESIAN_POINT('',(18.18,100.367257767916,2.19331515990198));
#70533=CARTESIAN_POINT('',(18.3,100.367257767916,2.19331515990198));
#70534=CARTESIAN_POINT('Ctrl Pts',(18.18,100.367257767916,2.19331515990198));
#70535=CARTESIAN_POINT('Ctrl Pts',(18.18,100.227012211084,2.15729875527322));
#70536=CARTESIAN_POINT('Ctrl Pts',(18.18,99.9890859663486,2.15729875527322));
#70537=CARTESIAN_POINT('Ctrl Pts',(18.3,100.605184161663,2.2926330383867));
#70538=CARTESIAN_POINT('Ctrl Pts',(18.1272,100.605184161663,2.2926330383867));
#70539=CARTESIAN_POINT('Ctrl Pts',(18.3,100.507503473759,2.22933141551912));
#70540=CARTESIAN_POINT('Ctrl Pts',(18.1272,100.507503473759,2.22933141551912));
#70541=CARTESIAN_POINT('Ctrl Pts',(18.3,100.367257767916,2.19331515990198));
#70542=CARTESIAN_POINT('Ctrl Pts',(18.1272,100.367257767916,2.19331515990198));
#70543=CARTESIAN_POINT('',(18.3,100.605184161663,2.2926330383867));
#70544=CARTESIAN_POINT('Ctrl Pts',(18.3,100.605184161663,2.2926330383867));
#70545=CARTESIAN_POINT('Ctrl Pts',(18.3,100.507503473759,2.22933141551912));
#70546=CARTESIAN_POINT('Ctrl Pts',(18.3,100.367257767916,2.19331515990198));
#70547=CARTESIAN_POINT('',(18.18,100.605184161663,2.2926330383867));
#70548=CARTESIAN_POINT('',(18.3,100.605184161663,2.2926330383867));
#70549=CARTESIAN_POINT('Ctrl Pts',(18.18,100.605184161663,2.2926330383867));
#70550=CARTESIAN_POINT('Ctrl Pts',(18.18,100.507503473759,2.22933141551912));
#70551=CARTESIAN_POINT('Ctrl Pts',(18.18,100.367257767916,2.19331515990198));
#70552=CARTESIAN_POINT('Ctrl Pts',(18.3,100.754706734419,2.45306966863573));
#70553=CARTESIAN_POINT('Ctrl Pts',(18.1272,100.754706734419,2.45306966863573));
#70554=CARTESIAN_POINT('Ctrl Pts',(18.3,100.702864998579,2.35593451224267));
#70555=CARTESIAN_POINT('Ctrl Pts',(18.1272,100.702864998579,2.35593451224267));
#70556=CARTESIAN_POINT('Ctrl Pts',(18.3,100.605184161663,2.2926330383867));
#70557=CARTESIAN_POINT('Ctrl Pts',(18.1272,100.605184161663,2.2926330383867));
#70558=CARTESIAN_POINT('',(18.3,100.754706734419,2.45306966863573));
#70559=CARTESIAN_POINT('Ctrl Pts',(18.3,100.754706734419,2.45306966863573));
#70560=CARTESIAN_POINT('Ctrl Pts',(18.3,100.702864998579,2.35593451224267));
#70561=CARTESIAN_POINT('Ctrl Pts',(18.3,100.605184161663,2.2926330383867));
#70562=CARTESIAN_POINT('',(18.18,100.754706734419,2.45306966863573));
#70563=CARTESIAN_POINT('',(18.3,100.754706734419,2.45306966863573));
#70564=CARTESIAN_POINT('Ctrl Pts',(18.18,100.754706734419,2.45306966863573));
#70565=CARTESIAN_POINT('Ctrl Pts',(18.18,100.702864998579,2.35593451224267));
#70566=CARTESIAN_POINT('Ctrl Pts',(18.18,100.605184161663,2.2926330383867));
#70567=CARTESIAN_POINT('Ctrl Pts',(18.3,100.806548470259,2.67899034582078));
#70568=CARTESIAN_POINT('Ctrl Pts',(18.1272,100.806548470259,2.67899034582078));
#70569=CARTESIAN_POINT('Ctrl Pts',(18.3,100.806548470259,2.55020467601716));
#70570=CARTESIAN_POINT('Ctrl Pts',(18.1272,100.806548470259,2.55020467601716));
#70571=CARTESIAN_POINT('Ctrl Pts',(18.3,100.754706734419,2.45306966863573));
#70572=CARTESIAN_POINT('Ctrl Pts',(18.1272,100.754706734419,2.45306966863573));
#70573=CARTESIAN_POINT('',(18.3,100.806548470259,2.67899034582078));
#70574=CARTESIAN_POINT('Ctrl Pts',(18.3,100.806548470259,2.67899034582078));
#70575=CARTESIAN_POINT('Ctrl Pts',(18.3,100.806548470259,2.55020467601716));
#70576=CARTESIAN_POINT('Ctrl Pts',(18.3,100.754706734419,2.45306966863573));
#70577=CARTESIAN_POINT('',(18.18,100.806548470259,2.67899034582078));
#70578=CARTESIAN_POINT('',(18.3,100.806548470259,2.67899034582078));
#70579=CARTESIAN_POINT('Ctrl Pts',(18.18,100.806548470259,2.67899034582078));
#70580=CARTESIAN_POINT('Ctrl Pts',(18.18,100.806548470259,2.55020467601716));
#70581=CARTESIAN_POINT('Ctrl Pts',(18.18,100.754706734419,2.45306966863573));
#70582=CARTESIAN_POINT('Ctrl Pts',(18.3,100.712687695026,2.96875847540796));
#70583=CARTESIAN_POINT('Ctrl Pts',(18.1272,100.712687695026,2.96875847540796));
#70584=CARTESIAN_POINT('Ctrl Pts',(18.3,100.806548470259,2.85361526571214));
#70585=CARTESIAN_POINT('Ctrl Pts',(18.1272,100.806548470259,2.85361526571214));
#70586=CARTESIAN_POINT('Ctrl Pts',(18.3,100.806548470259,2.67899034582078));
#70587=CARTESIAN_POINT('Ctrl Pts',(18.1272,100.806548470259,2.67899034582078));
#70588=CARTESIAN_POINT('',(18.3,100.712687695026,2.96875847540796));
#70589=CARTESIAN_POINT('Ctrl Pts',(18.3,100.712687695026,2.96875847540796));
#70590=CARTESIAN_POINT('Ctrl Pts',(18.3,100.806548470259,2.85361526571214));
#70591=CARTESIAN_POINT('Ctrl Pts',(18.3,100.806548470259,2.67899034582078));
#70592=CARTESIAN_POINT('',(18.18,100.712687695026,2.96875847540796));
#70593=CARTESIAN_POINT('',(18.3,100.712687695026,2.96875847540796));
#70594=CARTESIAN_POINT('Ctrl Pts',(18.18,100.712687695026,2.96875847540796));
#70595=CARTESIAN_POINT('Ctrl Pts',(18.18,100.806548470259,2.85361526571214));
#70596=CARTESIAN_POINT('Ctrl Pts',(18.18,100.806548470259,2.67899034582078));
#70597=CARTESIAN_POINT('Ctrl Pts',(18.3,100.445839041471,3.14229188524187));
#70598=CARTESIAN_POINT('Ctrl Pts',(18.1272,100.445839041471,3.14229188524187));
#70599=CARTESIAN_POINT('Ctrl Pts',(18.3,100.618826770782,3.08390168510377));
#70600=CARTESIAN_POINT('Ctrl Pts',(18.1272,100.618826770782,3.08390168510377));
#70601=CARTESIAN_POINT('Ctrl Pts',(18.3,100.712687695026,2.96875847540796));
#70602=CARTESIAN_POINT('Ctrl Pts',(18.1272,100.712687695026,2.96875847540796));
#70603=CARTESIAN_POINT('',(18.3,100.445839041471,3.14229188524187));
#70604=CARTESIAN_POINT('Ctrl Pts',(18.3,100.445839041471,3.14229188524187));
#70605=CARTESIAN_POINT('Ctrl Pts',(18.3,100.618826770782,3.08390168510377));
#70606=CARTESIAN_POINT('Ctrl Pts',(18.3,100.712687695026,2.96875847540796));
#70607=CARTESIAN_POINT('',(18.18,100.445839041471,3.14229188524187));
#70608=CARTESIAN_POINT('',(18.3,100.445839041471,3.14229188524187));
#70609=CARTESIAN_POINT('Ctrl Pts',(18.18,100.445839041471,3.14229188524187));
#70610=CARTESIAN_POINT('Ctrl Pts',(18.18,100.618826770782,3.08390168510377));
#70611=CARTESIAN_POINT('Ctrl Pts',(18.18,100.712687695026,2.96875847540796));
#70612=CARTESIAN_POINT('Ctrl Pts',(18.3,99.9890859663486,3.20068208537996));
#70613=CARTESIAN_POINT('Ctrl Pts',(18.1272,99.9890859663486,3.20068208537996));
#70614=CARTESIAN_POINT('Ctrl Pts',(18.3,100.27285131216,3.20068208537996));
#70615=CARTESIAN_POINT('Ctrl Pts',(18.1272,100.27285131216,3.20068208537996));
#70616=CARTESIAN_POINT('Ctrl Pts',(18.3,100.445839041471,3.14229188524187));
#70617=CARTESIAN_POINT('Ctrl Pts',(18.1272,100.445839041471,3.14229188524187));
#70618=CARTESIAN_POINT('',(18.3,99.9890859663486,3.20068208537996));
#70619=CARTESIAN_POINT('Ctrl Pts',(18.3,99.9890859663486,3.20068208537996));
#70620=CARTESIAN_POINT('Ctrl Pts',(18.3,100.27285131216,3.20068208537996));
#70621=CARTESIAN_POINT('Ctrl Pts',(18.3,100.445839041471,3.14229188524187));
#70622=CARTESIAN_POINT('',(18.18,99.9890859663486,3.20068208537996));
#70623=CARTESIAN_POINT('',(18.3,99.9890859663486,3.20068208537996));
#70624=CARTESIAN_POINT('Ctrl Pts',(18.18,99.9890859663486,3.20068208537996));
#70625=CARTESIAN_POINT('Ctrl Pts',(18.18,100.27285131216,3.20068208537996));
#70626=CARTESIAN_POINT('Ctrl Pts',(18.18,100.445839041471,3.14229188524187));
#70627=CARTESIAN_POINT('Ctrl Pts',(18.3,99.3386085569858,3.04242832623422));
#70628=CARTESIAN_POINT('Ctrl Pts',(18.1272,99.3386085569858,3.04242832623422));
#70629=CARTESIAN_POINT('Ctrl Pts',(18.3,99.5383356750011,3.20068208537996));
#70630=CARTESIAN_POINT('Ctrl Pts',(18.1272,99.5383356750011,3.20068208537996));
#70631=CARTESIAN_POINT('Ctrl Pts',(18.3,99.9890859663486,3.20068208537996));
#70632=CARTESIAN_POINT('Ctrl Pts',(18.1272,99.9890859663486,3.20068208537996));
#70633=CARTESIAN_POINT('Ctrl Pts',(18.3,99.3386085569858,3.04242832623422));
#70634=CARTESIAN_POINT('Ctrl Pts',(18.3,99.5383356750011,3.20068208537996));
#70635=CARTESIAN_POINT('Ctrl Pts',(18.3,99.9890859663486,3.20068208537996));
#70636=CARTESIAN_POINT('Ctrl Pts',(18.18,99.3386085569858,3.04242832623422));
#70637=CARTESIAN_POINT('Ctrl Pts',(18.18,99.5383356750011,3.20068208537996));
#70638=CARTESIAN_POINT('Ctrl Pts',(18.18,99.9890859663486,3.20068208537996));
#70639=CARTESIAN_POINT('Origin',(18.18,99.9890859663486,3.29999992661178));
#70640=CARTESIAN_POINT('Ctrl Pts',(18.3,99.1716234624386,3.93410628698766));
#70641=CARTESIAN_POINT('Ctrl Pts',(18.1272,99.1716234624386,3.93410628698766));
#70642=CARTESIAN_POINT('Ctrl Pts',(18.3,99.1716234624386,4.14474749974906));
#70643=CARTESIAN_POINT('Ctrl Pts',(18.1272,99.1716234624386,4.14474749974906));
#70644=CARTESIAN_POINT('Ctrl Pts',(18.3,99.2971350491047,4.28390165828168));
#70645=CARTESIAN_POINT('Ctrl Pts',(18.1272,99.2971350491047,4.28390165828168));
#70646=CARTESIAN_POINT('',(18.3,99.1716234624386,3.93410628698766));
#70647=CARTESIAN_POINT('',(18.3,99.2971350491047,4.28390165828168));
#70648=CARTESIAN_POINT('Ctrl Pts',(18.3,99.1716234624386,3.93410628698766));
#70649=CARTESIAN_POINT('Ctrl Pts',(18.3,99.1716234624386,4.14474749974906));
#70650=CARTESIAN_POINT('Ctrl Pts',(18.3,99.2971350491047,4.28390165828168));
#70651=CARTESIAN_POINT('',(18.18,99.1716234624386,3.93410628698766));
#70652=CARTESIAN_POINT('',(18.3,99.1716234624386,3.93410628698766));
#70653=CARTESIAN_POINT('',(18.18,99.2971350491047,4.28390165828168));
#70654=CARTESIAN_POINT('Ctrl Pts',(18.18,99.1716234624386,3.93410628698766));
#70655=CARTESIAN_POINT('Ctrl Pts',(18.18,99.1716234624386,4.14474749974906));
#70656=CARTESIAN_POINT('Ctrl Pts',(18.18,99.2971350491047,4.28390165828168));
#70657=CARTESIAN_POINT('',(18.3,99.2971350491047,4.28390165828168));
#70658=CARTESIAN_POINT('Ctrl Pts',(18.3,99.3173261225223,3.54774890504777));
#70659=CARTESIAN_POINT('Ctrl Pts',(18.1272,99.3173261225223,3.54774890504777));
#70660=CARTESIAN_POINT('Ctrl Pts',(18.3,99.1716234624386,3.70054563544691));
#70661=CARTESIAN_POINT('Ctrl Pts',(18.1272,99.1716234624386,3.70054563544691));
#70662=CARTESIAN_POINT('Ctrl Pts',(18.3,99.1716234624386,3.93410628698766));
#70663=CARTESIAN_POINT('Ctrl Pts',(18.1272,99.1716234624386,3.93410628698766));
#70664=CARTESIAN_POINT('',(18.3,99.3173261225223,3.54774890504777));
#70665=CARTESIAN_POINT('Ctrl Pts',(18.3,99.3173261225223,3.54774890504777));
#70666=CARTESIAN_POINT('Ctrl Pts',(18.3,99.1716234624386,3.70054563544691));
#70667=CARTESIAN_POINT('Ctrl Pts',(18.3,99.1716234624386,3.93410628698766));
#70668=CARTESIAN_POINT('',(18.18,99.3173261225223,3.54774890504777));
#70669=CARTESIAN_POINT('',(18.3,99.3173261225223,3.54774890504777));
#70670=CARTESIAN_POINT('Ctrl Pts',(18.18,99.3173261225223,3.54774890504777));
#70671=CARTESIAN_POINT('Ctrl Pts',(18.18,99.1716234624386,3.70054563544691));
#70672=CARTESIAN_POINT('Ctrl Pts',(18.18,99.1716234624386,3.93410628698766));
#70673=CARTESIAN_POINT('Ctrl Pts',(18.3,99.6725784480572,3.39495224915445));
#70674=CARTESIAN_POINT('Ctrl Pts',(18.1272,99.6725784480572,3.39495224915445));
#70675=CARTESIAN_POINT('Ctrl Pts',(18.3,99.4630287826061,3.39495224915445));
#70676=CARTESIAN_POINT('Ctrl Pts',(18.1272,99.4630287826061,3.39495224915445));
#70677=CARTESIAN_POINT('Ctrl Pts',(18.3,99.3173261225223,3.54774890504777));
#70678=CARTESIAN_POINT('Ctrl Pts',(18.1272,99.3173261225223,3.54774890504777));
#70679=CARTESIAN_POINT('',(18.3,99.6725784480572,3.39495224915445));
#70680=CARTESIAN_POINT('Ctrl Pts',(18.3,99.6725784480572,3.39495224915445));
#70681=CARTESIAN_POINT('Ctrl Pts',(18.3,99.4630287826061,3.39495224915445));
#70682=CARTESIAN_POINT('Ctrl Pts',(18.3,99.3173261225223,3.54774890504777));
#70683=CARTESIAN_POINT('',(18.18,99.6725784480572,3.39495224915445));
#70684=CARTESIAN_POINT('',(18.3,99.6725784480572,3.39495224915445));
#70685=CARTESIAN_POINT('Ctrl Pts',(18.18,99.6725784480572,3.39495224915445));
#70686=CARTESIAN_POINT('Ctrl Pts',(18.18,99.4630287826061,3.39495224915445));
#70687=CARTESIAN_POINT('Ctrl Pts',(18.18,99.3173261225223,3.54774890504777));
#70688=CARTESIAN_POINT('Ctrl Pts',(18.3,99.9306957662105,3.47353329919279));
#70689=CARTESIAN_POINT('Ctrl Pts',(18.1272,99.9306957662105,3.47353329919279));
#70690=CARTESIAN_POINT('Ctrl Pts',(18.3,99.8275579750538,3.39495224915445));
#70691=CARTESIAN_POINT('Ctrl Pts',(18.1272,99.8275579750538,3.39495224915445));
#70692=CARTESIAN_POINT('Ctrl Pts',(18.3,99.6725784480572,3.39495224915445));
#70693=CARTESIAN_POINT('Ctrl Pts',(18.1272,99.6725784480572,3.39495224915445));
#70694=CARTESIAN_POINT('',(18.3,99.9306957662105,3.47353329919279));
#70695=CARTESIAN_POINT('Ctrl Pts',(18.3,99.9306957662105,3.47353329919279));
#70696=CARTESIAN_POINT('Ctrl Pts',(18.3,99.8275579750538,3.39495224915445));
#70697=CARTESIAN_POINT('Ctrl Pts',(18.3,99.6725784480572,3.39495224915445));
#70698=CARTESIAN_POINT('',(18.18,99.9306957662105,3.47353329919279));
#70699=CARTESIAN_POINT('',(18.3,99.9306957662105,3.47353329919279));
#70700=CARTESIAN_POINT('Ctrl Pts',(18.18,99.9306957662105,3.47353329919279));
#70701=CARTESIAN_POINT('Ctrl Pts',(18.18,99.8275579750538,3.39495224915445));
#70702=CARTESIAN_POINT('Ctrl Pts',(18.18,99.6725784480572,3.39495224915445));
#70703=CARTESIAN_POINT('Ctrl Pts',(18.3,100.066575729847,3.69399717114866));
#70704=CARTESIAN_POINT('Ctrl Pts',(18.1272,100.066575729847,3.69399717114866));
#70705=CARTESIAN_POINT('Ctrl Pts',(18.3,100.033833557367,3.55211449824274));
#70706=CARTESIAN_POINT('Ctrl Pts',(18.1272,100.033833557367,3.55211449824274));
#70707=CARTESIAN_POINT('Ctrl Pts',(18.3,99.9306957662105,3.47353329919279));
#70708=CARTESIAN_POINT('Ctrl Pts',(18.1272,99.9306957662105,3.47353329919279));
#70709=CARTESIAN_POINT('',(18.3,100.066575729847,3.69399717114866));
#70710=CARTESIAN_POINT('Ctrl Pts',(18.3,100.066575729847,3.69399717114866));
#70711=CARTESIAN_POINT('Ctrl Pts',(18.3,100.033833557367,3.55211449824274));
#70712=CARTESIAN_POINT('Ctrl Pts',(18.3,99.9306957662105,3.47353329919279));
#70713=CARTESIAN_POINT('',(18.18,100.066575729847,3.69399717114866));
#70714=CARTESIAN_POINT('',(18.3,100.066575729847,3.69399717114866));
#70715=CARTESIAN_POINT('Ctrl Pts',(18.18,100.066575729847,3.69399717114866));
#70716=CARTESIAN_POINT('Ctrl Pts',(18.18,100.033833557367,3.55211449824274));
#70717=CARTESIAN_POINT('Ctrl Pts',(18.18,99.9306957662105,3.47353329919279));
#70718=CARTESIAN_POINT('Ctrl Pts',(18.3,100.20191001296,3.52919502221048));
#70719=CARTESIAN_POINT('Ctrl Pts',(18.1272,100.20191001296,3.52919502221048));
#70720=CARTESIAN_POINT('Ctrl Pts',(18.3,100.116780275106,3.58485667072237));
#70721=CARTESIAN_POINT('Ctrl Pts',(18.1272,100.116780275106,3.58485667072237));
#70722=CARTESIAN_POINT('Ctrl Pts',(18.3,100.066575729847,3.69399717114866));
#70723=CARTESIAN_POINT('Ctrl Pts',(18.1272,100.066575729847,3.69399717114866));
#70724=CARTESIAN_POINT('',(18.3,100.20191001296,3.52919502221048));
#70725=CARTESIAN_POINT('Ctrl Pts',(18.3,100.20191001296,3.52919502221048));
#70726=CARTESIAN_POINT('Ctrl Pts',(18.3,100.116780275106,3.58485667072237));
#70727=CARTESIAN_POINT('Ctrl Pts',(18.3,100.066575729847,3.69399717114866));
#70728=CARTESIAN_POINT('',(18.18,100.20191001296,3.52919502221048));
#70729=CARTESIAN_POINT('',(18.3,100.20191001296,3.52919502221048));
#70730=CARTESIAN_POINT('Ctrl Pts',(18.18,100.20191001296,3.52919502221048));
#70731=CARTESIAN_POINT('Ctrl Pts',(18.18,100.116780275106,3.58485667072237));
#70732=CARTESIAN_POINT('Ctrl Pts',(18.18,100.066575729847,3.69399717114866));
#70733=CARTESIAN_POINT('Ctrl Pts',(18.3,100.390723073483,3.47353329919279));
#70734=CARTESIAN_POINT('Ctrl Pts',(18.1272,100.390723073483,3.47353329919279));
#70735=CARTESIAN_POINT('Ctrl Pts',(18.3,100.287039601803,3.47353329919279));
#70736=CARTESIAN_POINT('Ctrl Pts',(18.1272,100.287039601803,3.47353329919279));
#70737=CARTESIAN_POINT('Ctrl Pts',(18.3,100.20191001296,3.52919502221048));
#70738=CARTESIAN_POINT('Ctrl Pts',(18.1272,100.20191001296,3.52919502221048));
#70739=CARTESIAN_POINT('',(18.3,100.390723073483,3.47353329919279));
#70740=CARTESIAN_POINT('Ctrl Pts',(18.3,100.390723073483,3.47353329919279));
#70741=CARTESIAN_POINT('Ctrl Pts',(18.3,100.287039601803,3.47353329919279));
#70742=CARTESIAN_POINT('Ctrl Pts',(18.3,100.20191001296,3.52919502221048));
#70743=CARTESIAN_POINT('',(18.18,100.390723073483,3.47353329919279));
#70744=CARTESIAN_POINT('',(18.3,100.390723073483,3.47353329919279));
#70745=CARTESIAN_POINT('Ctrl Pts',(18.18,100.390723073483,3.47353329919279));
#70746=CARTESIAN_POINT('Ctrl Pts',(18.18,100.287039601803,3.47353329919279));
#70747=CARTESIAN_POINT('Ctrl Pts',(18.18,100.20191001296,3.52919502221048));
#70748=CARTESIAN_POINT('Ctrl Pts',(18.3,100.596998506784,3.53192349933088));
#70749=CARTESIAN_POINT('Ctrl Pts',(18.1272,100.596998506784,3.53192349933088));
#70750=CARTESIAN_POINT('Ctrl Pts',(18.3,100.499863499403,3.47353329919279));
#70751=CARTESIAN_POINT('Ctrl Pts',(18.1272,100.499863499403,3.47353329919279));
#70752=CARTESIAN_POINT('Ctrl Pts',(18.3,100.390723073483,3.47353329919279));
#70753=CARTESIAN_POINT('Ctrl Pts',(18.1272,100.390723073483,3.47353329919279));
#70754=CARTESIAN_POINT('',(18.3,100.596998506784,3.53192349933088));
#70755=CARTESIAN_POINT('Ctrl Pts',(18.3,100.596998506784,3.53192349933088));
#70756=CARTESIAN_POINT('Ctrl Pts',(18.3,100.499863499403,3.47353329919279));
#70757=CARTESIAN_POINT('Ctrl Pts',(18.3,100.390723073483,3.47353329919279));
#70758=CARTESIAN_POINT('',(18.18,100.596998506784,3.53192349933088));
#70759=CARTESIAN_POINT('',(18.3,100.596998506784,3.53192349933088));
#70760=CARTESIAN_POINT('Ctrl Pts',(18.18,100.596998506784,3.53192349933088));
#70761=CARTESIAN_POINT('Ctrl Pts',(18.18,100.499863499403,3.47353329919279));
#70762=CARTESIAN_POINT('Ctrl Pts',(18.18,100.390723073483,3.47353329919279));
#70763=CARTESIAN_POINT('Ctrl Pts',(18.3,100.750340992212,3.70054563544691));
#70764=CARTESIAN_POINT('Ctrl Pts',(18.1272,100.750340992212,3.70054563544691));
#70765=CARTESIAN_POINT('Ctrl Pts',(18.3,100.694133663177,3.59031369946897));
#70766=CARTESIAN_POINT('Ctrl Pts',(18.1272,100.694133663177,3.59031369946897));
#70767=CARTESIAN_POINT('Ctrl Pts',(18.3,100.596998506784,3.53192349933088));
#70768=CARTESIAN_POINT('Ctrl Pts',(18.1272,100.596998506784,3.53192349933088));
#70769=CARTESIAN_POINT('',(18.3,100.750340992212,3.70054563544691));
#70770=CARTESIAN_POINT('Ctrl Pts',(18.3,100.750340992212,3.70054563544691));
#70771=CARTESIAN_POINT('Ctrl Pts',(18.3,100.694133663177,3.59031369946897));
#70772=CARTESIAN_POINT('Ctrl Pts',(18.3,100.596998506784,3.53192349933088));
#70773=CARTESIAN_POINT('',(18.18,100.750340992212,3.70054563544691));
#70774=CARTESIAN_POINT('',(18.3,100.750340992212,3.70054563544691));
#70775=CARTESIAN_POINT('Ctrl Pts',(18.18,100.750340992212,3.70054563544691));
#70776=CARTESIAN_POINT('Ctrl Pts',(18.18,100.694133663177,3.59031369946897));
#70777=CARTESIAN_POINT('Ctrl Pts',(18.18,100.596998506784,3.53192349933088));
#70778=CARTESIAN_POINT('Ctrl Pts',(18.3,100.806548321247,3.94174618683755));
#70779=CARTESIAN_POINT('Ctrl Pts',(18.1272,100.806548321247,3.94174618683755));
#70780=CARTESIAN_POINT('Ctrl Pts',(18.3,100.806548321247,3.81077749691904));
#70781=CARTESIAN_POINT('Ctrl Pts',(18.1272,100.806548321247,3.81077749691904));
#70782=CARTESIAN_POINT('Ctrl Pts',(18.3,100.750340992212,3.70054563544691));
#70783=CARTESIAN_POINT('Ctrl Pts',(18.1272,100.750340992212,3.70054563544691));
#70784=CARTESIAN_POINT('',(18.3,100.806548321247,3.94174618683755));
#70785=CARTESIAN_POINT('Ctrl Pts',(18.3,100.806548321247,3.94174618683755));
#70786=CARTESIAN_POINT('Ctrl Pts',(18.3,100.806548321247,3.81077749691904));
#70787=CARTESIAN_POINT('Ctrl Pts',(18.3,100.750340992212,3.70054563544691));
#70788=CARTESIAN_POINT('',(18.18,100.806548321247,3.94174618683755));
#70789=CARTESIAN_POINT('',(18.3,100.806548321247,3.94174618683755));
#70790=CARTESIAN_POINT('Ctrl Pts',(18.18,100.806548321247,3.94174618683755));
#70791=CARTESIAN_POINT('Ctrl Pts',(18.18,100.806548321247,3.81077749691904));
#70792=CARTESIAN_POINT('Ctrl Pts',(18.18,100.750340992212,3.70054563544691));
#70793=CARTESIAN_POINT('Ctrl Pts',(18.3,100.69795357585,4.25934502892196));
#70794=CARTESIAN_POINT('Ctrl Pts',(18.1272,100.69795357585,4.25934502892196));
#70795=CARTESIAN_POINT('Ctrl Pts',(18.3,100.806548321247,4.13165064565837));
#70796=CARTESIAN_POINT('Ctrl Pts',(18.1272,100.806548321247,4.13165064565837));
#70797=CARTESIAN_POINT('Ctrl Pts',(18.3,100.806548321247,3.94174618683755));
#70798=CARTESIAN_POINT('Ctrl Pts',(18.1272,100.806548321247,3.94174618683755));
#70799=CARTESIAN_POINT('',(18.3,100.69795357585,4.25934502892196));
#70800=CARTESIAN_POINT('Ctrl Pts',(18.3,100.69795357585,4.25934502892196));
#70801=CARTESIAN_POINT('Ctrl Pts',(18.3,100.806548321247,4.13165064565837));
#70802=CARTESIAN_POINT('Ctrl Pts',(18.3,100.806548321247,3.94174618683755));
#70803=CARTESIAN_POINT('',(18.18,100.69795357585,4.25934502892196));
#70804=CARTESIAN_POINT('',(18.3,100.69795357585,4.25934502892196));
#70805=CARTESIAN_POINT('Ctrl Pts',(18.18,100.69795357585,4.25934502892196));
#70806=CARTESIAN_POINT('Ctrl Pts',(18.18,100.806548321247,4.13165064565837));
#70807=CARTESIAN_POINT('Ctrl Pts',(18.18,100.806548321247,3.94174618683755));
#70808=CARTESIAN_POINT('Ctrl Pts',(18.3,100.39181458354,4.4230558168143));
#70809=CARTESIAN_POINT('Ctrl Pts',(18.1272,100.39181458354,4.4230558168143));
#70810=CARTESIAN_POINT('Ctrl Pts',(18.3,100.58935868144,4.38703944943845));
#70811=CARTESIAN_POINT('Ctrl Pts',(18.1272,100.58935868144,4.38703944943845));
#70812=CARTESIAN_POINT('Ctrl Pts',(18.3,100.69795357585,4.25934502892196));
#70813=CARTESIAN_POINT('Ctrl Pts',(18.1272,100.69795357585,4.25934502892196));
#70814=CARTESIAN_POINT('',(18.3,100.39181458354,4.4230558168143));
#70815=CARTESIAN_POINT('Ctrl Pts',(18.3,100.39181458354,4.4230558168143));
#70816=CARTESIAN_POINT('Ctrl Pts',(18.3,100.58935868144,4.38703944943845));
#70817=CARTESIAN_POINT('Ctrl Pts',(18.3,100.69795357585,4.25934502892196));
#70818=CARTESIAN_POINT('',(18.18,100.39181458354,4.4230558168143));
#70819=CARTESIAN_POINT('',(18.3,100.39181458354,4.4230558168143));
#70820=CARTESIAN_POINT('Ctrl Pts',(18.18,100.39181458354,4.4230558168143));
#70821=CARTESIAN_POINT('Ctrl Pts',(18.18,100.58935868144,4.38703944943845));
#70822=CARTESIAN_POINT('Ctrl Pts',(18.18,100.69795357585,4.25934502892196));
#70823=CARTESIAN_POINT('Origin',(18.3,100.356889539957,4.22660289369523));
#70824=CARTESIAN_POINT('',(18.3,100.356889539957,4.22660289369523));
#70825=CARTESIAN_POINT('',(18.3,100.001593808947,2.22806895448985));
#70826=CARTESIAN_POINT('',(18.18,100.356889539957,4.22660289369523));
#70827=CARTESIAN_POINT('',(18.3,100.356889539957,4.22660289369523));
#70828=CARTESIAN_POINT('',(18.18,100.356889539957,4.22660289369523));
#70829=CARTESIAN_POINT('Ctrl Pts',(18.3,100.572987669706,4.12837641350925));
#70830=CARTESIAN_POINT('Ctrl Pts',(18.1272,100.572987669706,4.12837641350925));
#70831=CARTESIAN_POINT('Ctrl Pts',(18.3,100.500954860449,4.20477477870882));
#70832=CARTESIAN_POINT('Ctrl Pts',(18.1272,100.500954860449,4.20477477870882));
#70833=CARTESIAN_POINT('Ctrl Pts',(18.3,100.356889539957,4.22660289369523));
#70834=CARTESIAN_POINT('Ctrl Pts',(18.1272,100.356889539957,4.22660289369523));
#70835=CARTESIAN_POINT('',(18.3,100.572987669706,4.12837641350925));
#70836=CARTESIAN_POINT('Ctrl Pts',(18.3,100.572987669706,4.12837641350925));
#70837=CARTESIAN_POINT('Ctrl Pts',(18.3,100.500954860449,4.20477477870882));
#70838=CARTESIAN_POINT('Ctrl Pts',(18.3,100.356889539957,4.22660289369523));
#70839=CARTESIAN_POINT('',(18.18,100.572987669706,4.12837641350925));
#70840=CARTESIAN_POINT('',(18.3,100.572987669706,4.12837641350925));
#70841=CARTESIAN_POINT('Ctrl Pts',(18.18,100.572987669706,4.12837641350925));
#70842=CARTESIAN_POINT('Ctrl Pts',(18.18,100.500954860449,4.20477477870882));
#70843=CARTESIAN_POINT('Ctrl Pts',(18.18,100.356889539957,4.22660289369523));
#70844=CARTESIAN_POINT('Ctrl Pts',(18.3,100.645020329952,3.93738051913679));
#70845=CARTESIAN_POINT('Ctrl Pts',(18.1272,100.645020329952,3.93738051913679));
#70846=CARTESIAN_POINT('Ctrl Pts',(18.3,100.645020329952,4.05197804830968));
#70847=CARTESIAN_POINT('Ctrl Pts',(18.1272,100.645020329952,4.05197804830968));
#70848=CARTESIAN_POINT('Ctrl Pts',(18.3,100.572987669706,4.12837641350925));
#70849=CARTESIAN_POINT('Ctrl Pts',(18.1272,100.572987669706,4.12837641350925));
#70850=CARTESIAN_POINT('',(18.3,100.645020329952,3.93738051913679));
#70851=CARTESIAN_POINT('Ctrl Pts',(18.3,100.645020329952,3.93738051913679));
#70852=CARTESIAN_POINT('Ctrl Pts',(18.3,100.645020329952,4.05197804830968));
#70853=CARTESIAN_POINT('Ctrl Pts',(18.3,100.572987669706,4.12837641350925));
#70854=CARTESIAN_POINT('',(18.18,100.645020329952,3.93738051913679));
#70855=CARTESIAN_POINT('',(18.3,100.645020329952,3.93738051913679));
#70856=CARTESIAN_POINT('Ctrl Pts',(18.18,100.645020329952,3.93738051913679));
#70857=CARTESIAN_POINT('Ctrl Pts',(18.18,100.645020329952,4.05197804830968));
#70858=CARTESIAN_POINT('Ctrl Pts',(18.18,100.572987669706,4.12837641350925));
#70859=CARTESIAN_POINT('Ctrl Pts',(18.3,100.574079030752,3.74856745861471));
#70860=CARTESIAN_POINT('Ctrl Pts',(18.1272,100.574079030752,3.74856745861471));
#70861=CARTESIAN_POINT('Ctrl Pts',(18.3,100.645020329952,3.82169162891805));
#70862=CARTESIAN_POINT('Ctrl Pts',(18.1272,100.645020329952,3.82169162891805));
#70863=CARTESIAN_POINT('Ctrl Pts',(18.3,100.645020329952,3.93738051913679));
#70864=CARTESIAN_POINT('Ctrl Pts',(18.1272,100.645020329952,3.93738051913679));
#70865=CARTESIAN_POINT('',(18.3,100.574079030752,3.74856745861471));
#70866=CARTESIAN_POINT('Ctrl Pts',(18.3,100.574079030752,3.74856745861471));
#70867=CARTESIAN_POINT('Ctrl Pts',(18.3,100.645020329952,3.82169162891805));
#70868=CARTESIAN_POINT('Ctrl Pts',(18.3,100.645020329952,3.93738051913679));
#70869=CARTESIAN_POINT('',(18.18,100.574079030752,3.74856745861471));
#70870=CARTESIAN_POINT('',(18.3,100.574079030752,3.74856745861471));
#70871=CARTESIAN_POINT('Ctrl Pts',(18.18,100.574079030752,3.74856745861471));
#70872=CARTESIAN_POINT('Ctrl Pts',(18.18,100.645020329952,3.82169162891805));
#70873=CARTESIAN_POINT('Ctrl Pts',(18.18,100.645020329952,3.93738051913679));
#70874=CARTESIAN_POINT('Ctrl Pts',(18.3,100.395088666677,3.67544328831136));
#70875=CARTESIAN_POINT('Ctrl Pts',(18.1272,100.395088666677,3.67544328831136));
#70876=CARTESIAN_POINT('Ctrl Pts',(18.3,100.503137731552,3.67544328831136));
#70877=CARTESIAN_POINT('Ctrl Pts',(18.1272,100.503137731552,3.67544328831136));
#70878=CARTESIAN_POINT('Ctrl Pts',(18.3,100.574079030752,3.74856745861471));
#70879=CARTESIAN_POINT('Ctrl Pts',(18.1272,100.574079030752,3.74856745861471));
#70880=CARTESIAN_POINT('',(18.3,100.395088666677,3.67544328831136));
#70881=CARTESIAN_POINT('Ctrl Pts',(18.3,100.395088666677,3.67544328831136));
#70882=CARTESIAN_POINT('Ctrl Pts',(18.3,100.503137731552,3.67544328831136));
#70883=CARTESIAN_POINT('Ctrl Pts',(18.3,100.574079030752,3.74856745861471));
#70884=CARTESIAN_POINT('',(18.18,100.395088666677,3.67544328831136));
#70885=CARTESIAN_POINT('',(18.3,100.395088666677,3.67544328831136));
#70886=CARTESIAN_POINT('Ctrl Pts',(18.18,100.395088666677,3.67544328831136));
#70887=CARTESIAN_POINT('Ctrl Pts',(18.18,100.503137731552,3.67544328831136));
#70888=CARTESIAN_POINT('Ctrl Pts',(18.18,100.574079030752,3.74856745861471));
#70889=CARTESIAN_POINT('Ctrl Pts',(18.3,100.193178826571,3.77585252784193));
#70890=CARTESIAN_POINT('Ctrl Pts',(18.1272,100.193178826571,3.77585252784193));
#70891=CARTESIAN_POINT('Ctrl Pts',(18.3,100.258663022518,3.67544328831136));
#70892=CARTESIAN_POINT('Ctrl Pts',(18.1272,100.258663022518,3.67544328831136));
#70893=CARTESIAN_POINT('Ctrl Pts',(18.3,100.395088666677,3.67544328831136));
#70894=CARTESIAN_POINT('Ctrl Pts',(18.1272,100.395088666677,3.67544328831136));
#70895=CARTESIAN_POINT('',(18.3,100.193178826571,3.77585252784193));
#70896=CARTESIAN_POINT('Ctrl Pts',(18.3,100.193178826571,3.77585252784193));
#70897=CARTESIAN_POINT('Ctrl Pts',(18.3,100.258663022518,3.67544328831136));
#70898=CARTESIAN_POINT('Ctrl Pts',(18.3,100.395088666677,3.67544328831136));
#70899=CARTESIAN_POINT('',(18.18,100.193178826571,3.77585252784193));
#70900=CARTESIAN_POINT('',(18.3,100.193178826571,3.77585252784193));
#70901=CARTESIAN_POINT('Ctrl Pts',(18.18,100.193178826571,3.77585252784193));
#70902=CARTESIAN_POINT('Ctrl Pts',(18.18,100.258663022518,3.67544328831136));
#70903=CARTESIAN_POINT('Ctrl Pts',(18.18,100.395088666677,3.67544328831136));
#70904=CARTESIAN_POINT('Ctrl Pts',(18.3,100.127694481611,4.0017734285444));
#70905=CARTESIAN_POINT('Ctrl Pts',(18.1272,100.127694481611,4.0017734285444));
#70906=CARTESIAN_POINT('Ctrl Pts',(18.3,100.127694481611,3.87626184187829));
#70907=CARTESIAN_POINT('Ctrl Pts',(18.1272,100.127694481611,3.87626184187829));
#70908=CARTESIAN_POINT('Ctrl Pts',(18.3,100.193178826571,3.77585252784193));
#70909=CARTESIAN_POINT('Ctrl Pts',(18.1272,100.193178826571,3.77585252784193));
#70910=CARTESIAN_POINT('',(18.3,100.127694481611,4.0017734285444));
#70911=CARTESIAN_POINT('Ctrl Pts',(18.3,100.127694481611,4.0017734285444));
#70912=CARTESIAN_POINT('Ctrl Pts',(18.3,100.127694481611,3.87626184187829));
#70913=CARTESIAN_POINT('Ctrl Pts',(18.3,100.193178826571,3.77585252784193));
#70914=CARTESIAN_POINT('',(18.18,100.127694481611,4.0017734285444));
#70915=CARTESIAN_POINT('',(18.3,100.127694481611,4.0017734285444));
#70916=CARTESIAN_POINT('Ctrl Pts',(18.18,100.127694481611,4.0017734285444));
#70917=CARTESIAN_POINT('Ctrl Pts',(18.18,100.127694481611,3.87626184187829));
#70918=CARTESIAN_POINT('Ctrl Pts',(18.18,100.193178826571,3.77585252784193));
#70919=CARTESIAN_POINT('Ctrl Pts',(18.3,100.129877203703,4.03342416547239));
#70920=CARTESIAN_POINT('Ctrl Pts',(18.1272,100.129877203703,4.03342416547239));
#70921=CARTESIAN_POINT('Ctrl Pts',(18.3,100.127694481611,4.01377884708345));
#70922=CARTESIAN_POINT('Ctrl Pts',(18.1272,100.127694481611,4.01377884708345));
#70923=CARTESIAN_POINT('Ctrl Pts',(18.3,100.127694481611,4.0017734285444));
#70924=CARTESIAN_POINT('Ctrl Pts',(18.1272,100.127694481611,4.0017734285444));
#70925=CARTESIAN_POINT('',(18.3,100.129877203703,4.03342416547239));
#70926=CARTESIAN_POINT('Ctrl Pts',(18.3,100.129877203703,4.03342416547239));
#70927=CARTESIAN_POINT('Ctrl Pts',(18.3,100.127694481611,4.01377884708345));
#70928=CARTESIAN_POINT('Ctrl Pts',(18.3,100.127694481611,4.0017734285444));
#70929=CARTESIAN_POINT('',(18.18,100.129877203703,4.03342416547239));
#70930=CARTESIAN_POINT('',(18.3,100.129877203703,4.03342416547239));
#70931=CARTESIAN_POINT('Ctrl Pts',(18.18,100.129877203703,4.03342416547239));
#70932=CARTESIAN_POINT('Ctrl Pts',(18.18,100.127694481611,4.01377884708345));
#70933=CARTESIAN_POINT('Ctrl Pts',(18.18,100.127694481611,4.0017734285444));
#70934=CARTESIAN_POINT('Origin',(18.3,99.9574353039265,4.05525228045881));
#70935=CARTESIAN_POINT('',(18.3,99.9574353039265,4.05525228045881));
#70936=CARTESIAN_POINT('',(18.3,85.124940537059,5.93278553500053));
#70937=CARTESIAN_POINT('',(18.18,99.9574353039265,4.05525228045881));
#70938=CARTESIAN_POINT('',(18.3,99.9574353039265,4.05525228045881));
#70939=CARTESIAN_POINT('',(18.18,99.9574353039265,4.05525228045881));
#70940=CARTESIAN_POINT('Ctrl Pts',(18.3,99.9792634189129,3.91664383970201));
#70941=CARTESIAN_POINT('Ctrl Pts',(18.1272,99.9792634189129,3.91664383970201));
#70942=CARTESIAN_POINT('Ctrl Pts',(18.3,99.9792634189129,3.9723054882139));
#70943=CARTESIAN_POINT('Ctrl Pts',(18.1272,99.9792634189129,3.9723054882139));
#70944=CARTESIAN_POINT('Ctrl Pts',(18.3,99.9574353039265,4.05525228045881));
#70945=CARTESIAN_POINT('Ctrl Pts',(18.1272,99.9574353039265,4.05525228045881));
#70946=CARTESIAN_POINT('',(18.3,99.9792634189129,3.91664383970201));
#70947=CARTESIAN_POINT('Ctrl Pts',(18.3,99.9792634189129,3.91664383970201));
#70948=CARTESIAN_POINT('Ctrl Pts',(18.3,99.9792634189129,3.9723054882139));
#70949=CARTESIAN_POINT('Ctrl Pts',(18.3,99.9574353039265,4.05525228045881));
#70950=CARTESIAN_POINT('',(18.18,99.9792634189129,3.91664383970201));
#70951=CARTESIAN_POINT('',(18.3,99.9792634189129,3.91664383970201));
#70952=CARTESIAN_POINT('Ctrl Pts',(18.18,99.9792634189129,3.91664383970201));
#70953=CARTESIAN_POINT('Ctrl Pts',(18.18,99.9792634189129,3.9723054882139));
#70954=CARTESIAN_POINT('Ctrl Pts',(18.18,99.9574353039265,4.05525228045881));
#70955=CARTESIAN_POINT('Ctrl Pts',(18.3,99.8914052784443,3.69181437455118));
#70956=CARTESIAN_POINT('Ctrl Pts',(18.1272,99.8914052784443,3.69181437455118));
#70957=CARTESIAN_POINT('Ctrl Pts',(18.3,99.9792634189129,3.78021819554269));
#70958=CARTESIAN_POINT('Ctrl Pts',(18.1272,99.9792634189129,3.78021819554269));
#70959=CARTESIAN_POINT('Ctrl Pts',(18.3,99.9792634189129,3.91664383970201));
#70960=CARTESIAN_POINT('Ctrl Pts',(18.1272,99.9792634189129,3.91664383970201));
#70961=CARTESIAN_POINT('',(18.3,99.8914052784443,3.69181437455118));
#70962=CARTESIAN_POINT('Ctrl Pts',(18.3,99.8914052784443,3.69181437455118));
#70963=CARTESIAN_POINT('Ctrl Pts',(18.3,99.9792634189129,3.78021819554269));
#70964=CARTESIAN_POINT('Ctrl Pts',(18.3,99.9792634189129,3.91664383970201));
#70965=CARTESIAN_POINT('',(18.18,99.8914052784443,3.69181437455118));
#70966=CARTESIAN_POINT('',(18.3,99.8914052784443,3.69181437455118));
#70967=CARTESIAN_POINT('Ctrl Pts',(18.18,99.8914052784443,3.69181437455118));
#70968=CARTESIAN_POINT('Ctrl Pts',(18.18,99.9792634189129,3.78021819554269));
#70969=CARTESIAN_POINT('Ctrl Pts',(18.18,99.9792634189129,3.91664383970201));
#70970=CARTESIAN_POINT('Ctrl Pts',(18.3,99.6682130038738,3.60341055355966));
#70971=CARTESIAN_POINT('Ctrl Pts',(18.1272,99.6682130038738,3.60341055355966));
#70972=CARTESIAN_POINT('Ctrl Pts',(18.3,99.8035471379757,3.60341055355966));
#70973=CARTESIAN_POINT('Ctrl Pts',(18.1272,99.8035471379757,3.60341055355966));
#70974=CARTESIAN_POINT('Ctrl Pts',(18.3,99.8914052784443,3.69181437455118));
#70975=CARTESIAN_POINT('Ctrl Pts',(18.1272,99.8914052784443,3.69181437455118));
#70976=CARTESIAN_POINT('',(18.3,99.6682130038738,3.60341055355966));
#70977=CARTESIAN_POINT('Ctrl Pts',(18.3,99.6682130038738,3.60341055355966));
#70978=CARTESIAN_POINT('Ctrl Pts',(18.3,99.8035471379757,3.60341055355966));
#70979=CARTESIAN_POINT('Ctrl Pts',(18.3,99.8914052784443,3.69181437455118));
#70980=CARTESIAN_POINT('',(18.18,99.6682130038738,3.60341055355966));
#70981=CARTESIAN_POINT('',(18.3,99.6682130038738,3.60341055355966));
#70982=CARTESIAN_POINT('Ctrl Pts',(18.18,99.6682130038738,3.60341055355966));
#70983=CARTESIAN_POINT('Ctrl Pts',(18.18,99.8035471379757,3.60341055355966));
#70984=CARTESIAN_POINT('Ctrl Pts',(18.18,99.8914052784443,3.69181437455118));
#70985=CARTESIAN_POINT('Ctrl Pts',(18.3,99.4302864611149,3.69890851937234));
#70986=CARTESIAN_POINT('Ctrl Pts',(18.1272,99.4302864611149,3.69890851937234));
#70987=CARTESIAN_POINT('Ctrl Pts',(18.3,99.5263301074505,3.60341055355966));
#70988=CARTESIAN_POINT('Ctrl Pts',(18.1272,99.5263301074505,3.60341055355966));
#70989=CARTESIAN_POINT('Ctrl Pts',(18.3,99.6682130038738,3.60341055355966));
#70990=CARTESIAN_POINT('Ctrl Pts',(18.1272,99.6682130038738,3.60341055355966));
#70991=CARTESIAN_POINT('',(18.3,99.4302864611149,3.69890851937234));
#70992=CARTESIAN_POINT('Ctrl Pts',(18.3,99.4302864611149,3.69890851937234));
#70993=CARTESIAN_POINT('Ctrl Pts',(18.3,99.5263301074505,3.60341055355966));
#70994=CARTESIAN_POINT('Ctrl Pts',(18.3,99.6682130038738,3.60341055355966));
#70995=CARTESIAN_POINT('',(18.18,99.4302864611149,3.69890851937234));
#70996=CARTESIAN_POINT('',(18.3,99.4302864611149,3.69890851937234));
#70997=CARTESIAN_POINT('Ctrl Pts',(18.18,99.4302864611149,3.69890851937234));
#70998=CARTESIAN_POINT('Ctrl Pts',(18.18,99.5263301074505,3.60341055355966));
#70999=CARTESIAN_POINT('Ctrl Pts',(18.18,99.6682130038738,3.60341055355966));
#71000=CARTESIAN_POINT('Ctrl Pts',(18.3,99.3342428147793,3.93301485143602));
#71001=CARTESIAN_POINT('Ctrl Pts',(18.1272,99.3342428147793,3.93301485143602));
#71002=CARTESIAN_POINT('Ctrl Pts',(18.3,99.3342428147793,3.79440641067922));
#71003=CARTESIAN_POINT('Ctrl Pts',(18.1272,99.3342428147793,3.79440641067922));
#71004=CARTESIAN_POINT('Ctrl Pts',(18.3,99.4302864611149,3.69890851937234));
#71005=CARTESIAN_POINT('Ctrl Pts',(18.1272,99.4302864611149,3.69890851937234));
#71006=CARTESIAN_POINT('',(18.3,99.3342428147793,3.93301485143602));
#71007=CARTESIAN_POINT('Ctrl Pts',(18.3,99.3342428147793,3.93301485143602));
#71008=CARTESIAN_POINT('Ctrl Pts',(18.3,99.3342428147793,3.79440641067922));
#71009=CARTESIAN_POINT('Ctrl Pts',(18.3,99.4302864611149,3.69890851937234));
#71010=CARTESIAN_POINT('',(18.18,99.3342428147793,3.93301485143602));
#71011=CARTESIAN_POINT('',(18.3,99.3342428147793,3.93301485143602));
#71012=CARTESIAN_POINT('Ctrl Pts',(18.18,99.3342428147793,3.93301485143602));
#71013=CARTESIAN_POINT('Ctrl Pts',(18.18,99.3342428147793,3.79440641067922));
#71014=CARTESIAN_POINT('Ctrl Pts',(18.18,99.4302864611149,3.69890851937234));
#71015=CARTESIAN_POINT('Ctrl Pts',(18.3,99.4079126656055,4.13110492788255));
#71016=CARTESIAN_POINT('Ctrl Pts',(18.1272,99.4079126656055,4.13110492788255));
#71017=CARTESIAN_POINT('Ctrl Pts',(18.3,99.3342428147793,4.0497952517122));
#71018=CARTESIAN_POINT('Ctrl Pts',(18.1272,99.3342428147793,4.0497952517122));
#71019=CARTESIAN_POINT('Ctrl Pts',(18.3,99.3342428147793,3.93301485143602));
#71020=CARTESIAN_POINT('Ctrl Pts',(18.1272,99.3342428147793,3.93301485143602));
#71021=CARTESIAN_POINT('',(18.3,99.4079126656055,4.13110492788255));
#71022=CARTESIAN_POINT('Ctrl Pts',(18.3,99.4079126656055,4.13110492788255));
#71023=CARTESIAN_POINT('Ctrl Pts',(18.3,99.3342428147793,4.0497952517122));
#71024=CARTESIAN_POINT('Ctrl Pts',(18.3,99.3342428147793,3.93301485143602));
#71025=CARTESIAN_POINT('',(18.18,99.4079126656055,4.13110492788255));
#71026=CARTESIAN_POINT('',(18.3,99.4079126656055,4.13110492788255));
#71027=CARTESIAN_POINT('Ctrl Pts',(18.18,99.4079126656055,4.13110492788255));
#71028=CARTESIAN_POINT('Ctrl Pts',(18.18,99.3342428147793,4.0497952517122));
#71029=CARTESIAN_POINT('Ctrl Pts',(18.18,99.3342428147793,3.93301485143602));
#71030=CARTESIAN_POINT('Ctrl Pts',(18.3,99.6485676109791,4.24624817483127));
#71031=CARTESIAN_POINT('Ctrl Pts',(18.1272,99.6485676109791,4.24624817483127));
#71032=CARTESIAN_POINT('Ctrl Pts',(18.3,99.4815825164318,4.2124146413058));
#71033=CARTESIAN_POINT('Ctrl Pts',(18.1272,99.4815825164318,4.2124146413058));
#71034=CARTESIAN_POINT('Ctrl Pts',(18.3,99.4079126656055,4.13110492788255));
#71035=CARTESIAN_POINT('Ctrl Pts',(18.1272,99.4079126656055,4.13110492788255));
#71036=CARTESIAN_POINT('',(18.3,99.6485676109791,4.24624817483127));
#71037=CARTESIAN_POINT('Ctrl Pts',(18.3,99.6485676109791,4.24624817483127));
#71038=CARTESIAN_POINT('Ctrl Pts',(18.3,99.4815825164318,4.2124146413058));
#71039=CARTESIAN_POINT('Ctrl Pts',(18.3,99.4079126656055,4.13110492788255));
#71040=CARTESIAN_POINT('',(18.18,99.6485676109791,4.24624817483127));
#71041=CARTESIAN_POINT('',(18.3,99.6485676109791,4.24624817483127));
#71042=CARTESIAN_POINT('Ctrl Pts',(18.18,99.6485676109791,4.24624817483127));
#71043=CARTESIAN_POINT('Ctrl Pts',(18.18,99.4815825164318,4.2124146413058));
#71044=CARTESIAN_POINT('Ctrl Pts',(18.18,99.4079126656055,4.13110492788255));
#71045=CARTESIAN_POINT('Origin',(18.3,99.6223737537861,4.44270109795034));
#71046=CARTESIAN_POINT('',(18.3,99.6223737537861,4.44270109795034));
#71047=CARTESIAN_POINT('',(18.3,99.2944047342843,6.90245615040001));
#71048=CARTESIAN_POINT('',(18.18,99.6223737537861,4.44270109795034));
#71049=CARTESIAN_POINT('',(18.3,99.6223737537861,4.44270109795034));
#71050=CARTESIAN_POINT('',(18.18,99.6223737537861,4.44270109795034));
#71051=CARTESIAN_POINT('Ctrl Pts',(18.3,99.2971350491047,4.28390165828168));
#71052=CARTESIAN_POINT('Ctrl Pts',(18.1272,99.2971350491047,4.28390165828168));
#71053=CARTESIAN_POINT('Ctrl Pts',(18.3,99.4226466357708,4.4230558168143));
#71054=CARTESIAN_POINT('Ctrl Pts',(18.1272,99.4226466357708,4.4230558168143));
#71055=CARTESIAN_POINT('Ctrl Pts',(18.3,99.6223737537861,4.44270109795034));
#71056=CARTESIAN_POINT('Ctrl Pts',(18.1272,99.6223737537861,4.44270109795034));
#71057=CARTESIAN_POINT('Ctrl Pts',(18.3,99.2971350491047,4.28390165828168));
#71058=CARTESIAN_POINT('Ctrl Pts',(18.3,99.4226466357708,4.4230558168143));
#71059=CARTESIAN_POINT('Ctrl Pts',(18.3,99.6223737537861,4.44270109795034));
#71060=CARTESIAN_POINT('Ctrl Pts',(18.18,99.2971350491047,4.28390165828168));
#71061=CARTESIAN_POINT('Ctrl Pts',(18.18,99.4226466357708,4.4230558168143));
#71062=CARTESIAN_POINT('Ctrl Pts',(18.18,99.6223737537861,4.44270109795034));
#71063=CARTESIAN_POINT('Origin',(18.18,99.9890859663486,3.29999992661178));
#71064=CARTESIAN_POINT('Origin',(18.3,70.,5.5));
#71065=CARTESIAN_POINT('Ctrl Pts',(18.3,90.643929117918,2.66698497384787));
#71066=CARTESIAN_POINT('Ctrl Pts',(18.1272,90.643929117918,2.66698497384787));
#71067=CARTESIAN_POINT('Ctrl Pts',(18.3,90.643929117918,2.80231925696135));
#71068=CARTESIAN_POINT('Ctrl Pts',(18.1272,90.643929117918,2.80231925696135));
#71069=CARTESIAN_POINT('Ctrl Pts',(18.3,90.5293315887451,2.88308325260878));
#71070=CARTESIAN_POINT('Ctrl Pts',(18.1272,90.5293315887451,2.88308325260878));
#71071=CARTESIAN_POINT('',(18.3,90.643929117918,2.66698497384787));
#71072=CARTESIAN_POINT('',(18.3,90.5293315887451,2.88308325260878));
#71073=CARTESIAN_POINT('Ctrl Pts',(18.3,90.643929117918,2.66698497384787));
#71074=CARTESIAN_POINT('Ctrl Pts',(18.3,90.643929117918,2.80231925696135));
#71075=CARTESIAN_POINT('Ctrl Pts',(18.3,90.5293315887451,2.88308325260878));
#71076=CARTESIAN_POINT('',(18.18,90.643929117918,2.66698497384787));
#71077=CARTESIAN_POINT('',(18.3,90.643929117918,2.66698497384787));
#71078=CARTESIAN_POINT('',(18.18,90.5293315887451,2.88308325260878));
#71079=CARTESIAN_POINT('Ctrl Pts',(18.18,90.643929117918,2.66698497384787));
#71080=CARTESIAN_POINT('Ctrl Pts',(18.18,90.643929117918,2.80231925696135));
#71081=CARTESIAN_POINT('Ctrl Pts',(18.18,90.5293315887451,2.88308325260878));
#71082=CARTESIAN_POINT('',(18.3,90.5293315887451,2.88308325260878));
#71083=CARTESIAN_POINT('Ctrl Pts',(18.3,90.5140519380569,2.43724423497915));
#71084=CARTESIAN_POINT('Ctrl Pts',(18.1272,90.5140519380569,2.43724423497915));
#71085=CARTESIAN_POINT('Ctrl Pts',(18.3,90.643929117918,2.52946796864271));
#71086=CARTESIAN_POINT('Ctrl Pts',(18.1272,90.643929117918,2.52946796864271));
#71087=CARTESIAN_POINT('Ctrl Pts',(18.3,90.643929117918,2.66698497384787));
#71088=CARTESIAN_POINT('Ctrl Pts',(18.1272,90.643929117918,2.66698497384787));
#71089=CARTESIAN_POINT('',(18.3,90.5140519380569,2.43724423497915));
#71090=CARTESIAN_POINT('Ctrl Pts',(18.3,90.5140519380569,2.43724423497915));
#71091=CARTESIAN_POINT('Ctrl Pts',(18.3,90.643929117918,2.52946796864271));
#71092=CARTESIAN_POINT('Ctrl Pts',(18.3,90.643929117918,2.66698497384787));
#71093=CARTESIAN_POINT('',(18.18,90.5140519380569,2.43724423497915));
#71094=CARTESIAN_POINT('',(18.3,90.5140519380569,2.43724423497915));
#71095=CARTESIAN_POINT('Ctrl Pts',(18.18,90.5140519380569,2.43724423497915));
#71096=CARTESIAN_POINT('Ctrl Pts',(18.18,90.643929117918,2.52946796864271));
#71097=CARTESIAN_POINT('Ctrl Pts',(18.18,90.643929117918,2.66698497384787));
#71098=CARTESIAN_POINT('Ctrl Pts',(18.3,89.9890859663486,2.34502050131559));
#71099=CARTESIAN_POINT('Ctrl Pts',(18.1272,89.9890859663486,2.34502050131559));
#71100=CARTESIAN_POINT('Ctrl Pts',(18.3,90.3841746091843,2.34502050131559));
#71101=CARTESIAN_POINT('Ctrl Pts',(18.1272,90.3841746091843,2.34502050131559));
#71102=CARTESIAN_POINT('Ctrl Pts',(18.3,90.5140519380569,2.43724423497915));
#71103=CARTESIAN_POINT('Ctrl Pts',(18.1272,90.5140519380569,2.43724423497915));
#71104=CARTESIAN_POINT('',(18.3,89.9890859663486,2.34502050131559));
#71105=CARTESIAN_POINT('Ctrl Pts',(18.3,89.9890859663486,2.34502050131559));
#71106=CARTESIAN_POINT('Ctrl Pts',(18.3,90.3841746091843,2.34502050131559));
#71107=CARTESIAN_POINT('Ctrl Pts',(18.3,90.5140519380569,2.43724423497915));
#71108=CARTESIAN_POINT('',(18.18,89.9890859663486,2.34502050131559));
#71109=CARTESIAN_POINT('',(18.3,89.9890859663486,2.34502050131559));
#71110=CARTESIAN_POINT('Ctrl Pts',(18.18,89.9890859663486,2.34502050131559));
#71111=CARTESIAN_POINT('Ctrl Pts',(18.18,90.3841746091843,2.34502050131559));
#71112=CARTESIAN_POINT('Ctrl Pts',(18.18,90.5140519380569,2.43724423497915));
#71113=CARTESIAN_POINT('Ctrl Pts',(18.3,89.4652115046978,2.43724423497915));
#71114=CARTESIAN_POINT('Ctrl Pts',(18.1272,89.4652115046978,2.43724423497915));
#71115=CARTESIAN_POINT('Ctrl Pts',(18.3,89.5961801946163,2.34502050131559));
#71116=CARTESIAN_POINT('Ctrl Pts',(18.1272,89.5961801946163,2.34502050131559));
#71117=CARTESIAN_POINT('Ctrl Pts',(18.3,89.9890859663486,2.34502050131559));
#71118=CARTESIAN_POINT('Ctrl Pts',(18.1272,89.9890859663486,2.34502050131559));
#71119=CARTESIAN_POINT('',(18.3,89.4652115046978,2.43724423497915));
#71120=CARTESIAN_POINT('Ctrl Pts',(18.3,89.4652115046978,2.43724423497915));
#71121=CARTESIAN_POINT('Ctrl Pts',(18.3,89.5961801946163,2.34502050131559));
#71122=CARTESIAN_POINT('Ctrl Pts',(18.3,89.9890859663486,2.34502050131559));
#71123=CARTESIAN_POINT('',(18.18,89.4652115046978,2.43724423497915));
#71124=CARTESIAN_POINT('',(18.3,89.4652115046978,2.43724423497915));
#71125=CARTESIAN_POINT('Ctrl Pts',(18.18,89.4652115046978,2.43724423497915));
#71126=CARTESIAN_POINT('Ctrl Pts',(18.18,89.5961801946163,2.34502050131559));
#71127=CARTESIAN_POINT('Ctrl Pts',(18.18,89.9890859663486,2.34502050131559));
#71128=CARTESIAN_POINT('Ctrl Pts',(18.3,89.3342428147793,2.66480210274458));
#71129=CARTESIAN_POINT('Ctrl Pts',(18.1272,89.3342428147793,2.66480210274458));
#71130=CARTESIAN_POINT('Ctrl Pts',(18.3,89.3342428147793,2.52946796864271));
#71131=CARTESIAN_POINT('Ctrl Pts',(18.1272,89.3342428147793,2.52946796864271));
#71132=CARTESIAN_POINT('Ctrl Pts',(18.3,89.4652115046978,2.43724423497915));
#71133=CARTESIAN_POINT('Ctrl Pts',(18.1272,89.4652115046978,2.43724423497915));
#71134=CARTESIAN_POINT('',(18.3,89.3342428147793,2.66480210274458));
#71135=CARTESIAN_POINT('Ctrl Pts',(18.3,89.3342428147793,2.66480210274458));
#71136=CARTESIAN_POINT('Ctrl Pts',(18.3,89.3342428147793,2.52946796864271));
#71137=CARTESIAN_POINT('Ctrl Pts',(18.3,89.4652115046978,2.43724423497915));
#71138=CARTESIAN_POINT('',(18.18,89.3342428147793,2.66480210274458));
#71139=CARTESIAN_POINT('',(18.3,89.3342428147793,2.66480210274458));
#71140=CARTESIAN_POINT('Ctrl Pts',(18.18,89.3342428147793,2.66480210274458));
#71141=CARTESIAN_POINT('Ctrl Pts',(18.18,89.3342428147793,2.52946796864271));
#71142=CARTESIAN_POINT('Ctrl Pts',(18.18,89.4652115046978,2.43724423497915));
#71143=CARTESIAN_POINT('Ctrl Pts',(18.3,89.4646658241749,2.89236011952162));
#71144=CARTESIAN_POINT('Ctrl Pts',(18.1272,89.4646658241749,2.89236011952162));
#71145=CARTESIAN_POINT('Ctrl Pts',(18.3,89.3342428147793,2.80013638585806));
#71146=CARTESIAN_POINT('Ctrl Pts',(18.1272,89.3342428147793,2.80013638585806));
#71147=CARTESIAN_POINT('Ctrl Pts',(18.3,89.3342428147793,2.66480210274458));
#71148=CARTESIAN_POINT('Ctrl Pts',(18.1272,89.3342428147793,2.66480210274458));
#71149=CARTESIAN_POINT('',(18.3,89.4646658241749,2.89236011952162));
#71150=CARTESIAN_POINT('Ctrl Pts',(18.3,89.4646658241749,2.89236011952162));
#71151=CARTESIAN_POINT('Ctrl Pts',(18.3,89.3342428147793,2.80013638585806));
#71152=CARTESIAN_POINT('Ctrl Pts',(18.3,89.3342428147793,2.66480210274458));
#71153=CARTESIAN_POINT('',(18.18,89.4646658241749,2.89236011952162));
#71154=CARTESIAN_POINT('',(18.3,89.4646658241749,2.89236011952162));
#71155=CARTESIAN_POINT('Ctrl Pts',(18.18,89.4646658241749,2.89236011952162));
#71156=CARTESIAN_POINT('Ctrl Pts',(18.18,89.3342428147793,2.80013638585806));
#71157=CARTESIAN_POINT('Ctrl Pts',(18.18,89.3342428147793,2.66480210274458));
#71158=CARTESIAN_POINT('Ctrl Pts',(18.3,89.9890859663486,2.98458385318518));
#71159=CARTESIAN_POINT('Ctrl Pts',(18.1272,89.9890859663486,2.98458385318518));
#71160=CARTESIAN_POINT('Ctrl Pts',(18.3,89.5950888335705,2.98458385318518));
#71161=CARTESIAN_POINT('Ctrl Pts',(18.1272,89.5950888335705,2.98458385318518));
#71162=CARTESIAN_POINT('Ctrl Pts',(18.3,89.4646658241749,2.89236011952162));
#71163=CARTESIAN_POINT('Ctrl Pts',(18.1272,89.4646658241749,2.89236011952162));
#71164=CARTESIAN_POINT('',(18.3,89.9890859663486,2.98458385318518));
#71165=CARTESIAN_POINT('Ctrl Pts',(18.3,89.9890859663486,2.98458385318518));
#71166=CARTESIAN_POINT('Ctrl Pts',(18.3,89.5950888335705,2.98458385318518));
#71167=CARTESIAN_POINT('Ctrl Pts',(18.3,89.4646658241749,2.89236011952162));
#71168=CARTESIAN_POINT('',(18.18,89.9890859663486,2.98458385318518));
#71169=CARTESIAN_POINT('',(18.3,89.9890859663486,2.98458385318518));
#71170=CARTESIAN_POINT('Ctrl Pts',(18.18,89.9890859663486,2.98458385318518));
#71171=CARTESIAN_POINT('Ctrl Pts',(18.18,89.5950888335705,2.98458385318518));
#71172=CARTESIAN_POINT('Ctrl Pts',(18.18,89.4646658241749,2.89236011952162));
#71173=CARTESIAN_POINT('Ctrl Pts',(18.3,90.5293315887451,2.88308325260878));
#71174=CARTESIAN_POINT('Ctrl Pts',(18.1272,90.5293315887451,2.88308325260878));
#71175=CARTESIAN_POINT('Ctrl Pts',(18.3,90.3830830991268,2.98458385318518));
#71176=CARTESIAN_POINT('Ctrl Pts',(18.1272,90.3830830991268,2.98458385318518));
#71177=CARTESIAN_POINT('Ctrl Pts',(18.3,89.9890859663486,2.98458385318518));
#71178=CARTESIAN_POINT('Ctrl Pts',(18.1272,89.9890859663486,2.98458385318518));
#71179=CARTESIAN_POINT('Ctrl Pts',(18.3,90.5293315887451,2.88308325260878));
#71180=CARTESIAN_POINT('Ctrl Pts',(18.3,90.3830830991268,2.98458385318518));
#71181=CARTESIAN_POINT('Ctrl Pts',(18.3,89.9890859663486,2.98458385318518));
#71182=CARTESIAN_POINT('Ctrl Pts',(18.18,90.5293315887451,2.88308325260878));
#71183=CARTESIAN_POINT('Ctrl Pts',(18.18,90.3830830991268,2.98458385318518));
#71184=CARTESIAN_POINT('Ctrl Pts',(18.18,89.9890859663486,2.98458385318518));
#71185=CARTESIAN_POINT('Ctrl Pts',(18.3,89.1727148234844,2.66480210274458));
#71186=CARTESIAN_POINT('Ctrl Pts',(18.1272,89.1727148234844,2.66480210274458));
#71187=CARTESIAN_POINT('Ctrl Pts',(18.3,89.1727148234844,2.89618003219366));
#71188=CARTESIAN_POINT('Ctrl Pts',(18.1272,89.1727148234844,2.89618003219366));
#71189=CARTESIAN_POINT('Ctrl Pts',(18.3,89.3386085569858,3.02824008315802));
#71190=CARTESIAN_POINT('Ctrl Pts',(18.1272,89.3386085569858,3.02824008315802));
#71191=CARTESIAN_POINT('',(18.3,89.1727148234844,2.66480210274458));
#71192=CARTESIAN_POINT('',(18.3,89.3386085569858,3.02824008315802));
#71193=CARTESIAN_POINT('Ctrl Pts',(18.3,89.1727148234844,2.66480210274458));
#71194=CARTESIAN_POINT('Ctrl Pts',(18.3,89.1727148234844,2.89618003219366));
#71195=CARTESIAN_POINT('Ctrl Pts',(18.3,89.3386085569858,3.02824008315802));
#71196=CARTESIAN_POINT('',(18.18,89.1727148234844,2.66480210274458));
#71197=CARTESIAN_POINT('',(18.3,89.1727148234844,2.66480210274458));
#71198=CARTESIAN_POINT('',(18.18,89.3386085569858,3.02824008315802));
#71199=CARTESIAN_POINT('Ctrl Pts',(18.18,89.1727148234844,2.66480210274458));
#71200=CARTESIAN_POINT('Ctrl Pts',(18.18,89.1727148234844,2.89618003219366));
#71201=CARTESIAN_POINT('Ctrl Pts',(18.18,89.3386085569858,3.02824008315802));
#71202=CARTESIAN_POINT('',(18.3,89.3386085569858,3.02824008315802));
#71203=CARTESIAN_POINT('Ctrl Pts',(18.3,89.2671214282513,2.37394276112318));
#71204=CARTESIAN_POINT('Ctrl Pts',(18.1272,89.2671214282513,2.37394276112318));
#71205=CARTESIAN_POINT('Ctrl Pts',(18.3,89.1727148234844,2.489085970819));
#71206=CARTESIAN_POINT('Ctrl Pts',(18.1272,89.1727148234844,2.489085970819));
#71207=CARTESIAN_POINT('Ctrl Pts',(18.3,89.1727148234844,2.66480210274458));
#71208=CARTESIAN_POINT('Ctrl Pts',(18.1272,89.1727148234844,2.66480210274458));
#71209=CARTESIAN_POINT('',(18.3,89.2671214282513,2.37394276112318));
#71210=CARTESIAN_POINT('Ctrl Pts',(18.3,89.2671214282513,2.37394276112318));
#71211=CARTESIAN_POINT('Ctrl Pts',(18.3,89.1727148234844,2.489085970819));
#71212=CARTESIAN_POINT('Ctrl Pts',(18.3,89.1727148234844,2.66480210274458));
#71213=CARTESIAN_POINT('',(18.18,89.2671214282513,2.37394276112318));
#71214=CARTESIAN_POINT('',(18.3,89.2671214282513,2.37394276112318));
#71215=CARTESIAN_POINT('Ctrl Pts',(18.18,89.2671214282513,2.37394276112318));
#71216=CARTESIAN_POINT('Ctrl Pts',(18.18,89.1727148234844,2.489085970819));
#71217=CARTESIAN_POINT('Ctrl Pts',(18.18,89.1727148234844,2.66480210274458));
#71218=CARTESIAN_POINT('Ctrl Pts',(18.3,89.5345156133175,2.20095503181219));
#71219=CARTESIAN_POINT('Ctrl Pts',(18.1272,89.5345156133175,2.20095503181219));
#71220=CARTESIAN_POINT('Ctrl Pts',(18.3,89.3615280330181,2.25879940241575));
#71221=CARTESIAN_POINT('Ctrl Pts',(18.1272,89.3615280330181,2.25879940241575));
#71222=CARTESIAN_POINT('Ctrl Pts',(18.3,89.2671214282513,2.37394276112318));
#71223=CARTESIAN_POINT('Ctrl Pts',(18.1272,89.2671214282513,2.37394276112318));
#71224=CARTESIAN_POINT('',(18.3,89.5345156133175,2.20095503181219));
#71225=CARTESIAN_POINT('Ctrl Pts',(18.3,89.5345156133175,2.20095503181219));
#71226=CARTESIAN_POINT('Ctrl Pts',(18.3,89.3615280330181,2.25879940241575));
#71227=CARTESIAN_POINT('Ctrl Pts',(18.3,89.2671214282513,2.37394276112318));
#71228=CARTESIAN_POINT('',(18.18,89.5345156133175,2.20095503181219));
#71229=CARTESIAN_POINT('',(18.3,89.5345156133175,2.20095503181219));
#71230=CARTESIAN_POINT('Ctrl Pts',(18.18,89.5345156133175,2.20095503181219));
#71231=CARTESIAN_POINT('Ctrl Pts',(18.18,89.3615280330181,2.25879940241575));
#71232=CARTESIAN_POINT('Ctrl Pts',(18.18,89.2671214282513,2.37394276112318));
#71233=CARTESIAN_POINT('Ctrl Pts',(18.3,89.9890859663486,2.14311051219702));
#71234=CARTESIAN_POINT('Ctrl Pts',(18.1272,89.9890859663486,2.14311051219702));
#71235=CARTESIAN_POINT('Ctrl Pts',(18.3,89.7075034916401,2.14311051219702));
#71236=CARTESIAN_POINT('Ctrl Pts',(18.1272,89.7075034916401,2.14311051219702));
#71237=CARTESIAN_POINT('Ctrl Pts',(18.3,89.5345156133175,2.20095503181219));
#71238=CARTESIAN_POINT('Ctrl Pts',(18.1272,89.5345156133175,2.20095503181219));
#71239=CARTESIAN_POINT('',(18.3,89.9890859663486,2.14311051219702));
#71240=CARTESIAN_POINT('Ctrl Pts',(18.3,89.9890859663486,2.14311051219702));
#71241=CARTESIAN_POINT('Ctrl Pts',(18.3,89.7075034916401,2.14311051219702));
#71242=CARTESIAN_POINT('Ctrl Pts',(18.3,89.5345156133175,2.20095503181219));
#71243=CARTESIAN_POINT('',(18.18,89.9890859663486,2.14311051219702));
#71244=CARTESIAN_POINT('',(18.3,89.9890859663486,2.14311051219702));
#71245=CARTESIAN_POINT('Ctrl Pts',(18.18,89.9890859663486,2.14311051219702));
#71246=CARTESIAN_POINT('Ctrl Pts',(18.18,89.7075034916401,2.14311051219702));
#71247=CARTESIAN_POINT('Ctrl Pts',(18.18,89.5345156133175,2.20095503181219));
#71248=CARTESIAN_POINT('Ctrl Pts',(18.3,90.3672577679157,2.17912691682577));
#71249=CARTESIAN_POINT('Ctrl Pts',(18.1272,90.3672577679157,2.17912691682577));
#71250=CARTESIAN_POINT('Ctrl Pts',(18.3,90.2270122110844,2.14311051219702));
#71251=CARTESIAN_POINT('Ctrl Pts',(18.1272,90.2270122110844,2.14311051219702));
#71252=CARTESIAN_POINT('Ctrl Pts',(18.3,89.9890859663486,2.14311051219702));
#71253=CARTESIAN_POINT('Ctrl Pts',(18.1272,89.9890859663486,2.14311051219702));
#71254=CARTESIAN_POINT('',(18.3,90.3672577679157,2.17912691682577));
#71255=CARTESIAN_POINT('Ctrl Pts',(18.3,90.3672577679157,2.17912691682577));
#71256=CARTESIAN_POINT('Ctrl Pts',(18.3,90.2270122110844,2.14311051219702));
#71257=CARTESIAN_POINT('Ctrl Pts',(18.3,89.9890859663486,2.14311051219702));
#71258=CARTESIAN_POINT('',(18.18,90.3672577679157,2.17912691682577));
#71259=CARTESIAN_POINT('',(18.3,90.3672577679157,2.17912691682577));
#71260=CARTESIAN_POINT('Ctrl Pts',(18.18,90.3672577679157,2.17912691682577));
#71261=CARTESIAN_POINT('Ctrl Pts',(18.18,90.2270122110844,2.14311051219702));
#71262=CARTESIAN_POINT('Ctrl Pts',(18.18,89.9890859663486,2.14311051219702));
#71263=CARTESIAN_POINT('Ctrl Pts',(18.3,90.605184161663,2.2784447953105));
#71264=CARTESIAN_POINT('Ctrl Pts',(18.1272,90.605184161663,2.2784447953105));
#71265=CARTESIAN_POINT('Ctrl Pts',(18.3,90.5075034737587,2.21514317244291));
#71266=CARTESIAN_POINT('Ctrl Pts',(18.1272,90.5075034737587,2.21514317244291));
#71267=CARTESIAN_POINT('Ctrl Pts',(18.3,90.3672577679157,2.17912691682577));
#71268=CARTESIAN_POINT('Ctrl Pts',(18.1272,90.3672577679157,2.17912691682577));
#71269=CARTESIAN_POINT('',(18.3,90.605184161663,2.2784447953105));
#71270=CARTESIAN_POINT('Ctrl Pts',(18.3,90.605184161663,2.2784447953105));
#71271=CARTESIAN_POINT('Ctrl Pts',(18.3,90.5075034737587,2.21514317244291));
#71272=CARTESIAN_POINT('Ctrl Pts',(18.3,90.3672577679157,2.17912691682577));
#71273=CARTESIAN_POINT('',(18.18,90.605184161663,2.2784447953105));
#71274=CARTESIAN_POINT('',(18.3,90.605184161663,2.2784447953105));
#71275=CARTESIAN_POINT('Ctrl Pts',(18.18,90.605184161663,2.2784447953105));
#71276=CARTESIAN_POINT('Ctrl Pts',(18.18,90.5075034737587,2.21514317244291));
#71277=CARTESIAN_POINT('Ctrl Pts',(18.18,90.3672577679157,2.17912691682577));
#71278=CARTESIAN_POINT('Ctrl Pts',(18.3,90.7547067344189,2.43888142555952));
#71279=CARTESIAN_POINT('Ctrl Pts',(18.1272,90.7547067344189,2.43888142555952));
#71280=CARTESIAN_POINT('Ctrl Pts',(18.3,90.702864998579,2.34174626916647));
#71281=CARTESIAN_POINT('Ctrl Pts',(18.1272,90.702864998579,2.34174626916647));
#71282=CARTESIAN_POINT('Ctrl Pts',(18.3,90.605184161663,2.2784447953105));
#71283=CARTESIAN_POINT('Ctrl Pts',(18.1272,90.605184161663,2.2784447953105));
#71284=CARTESIAN_POINT('',(18.3,90.7547067344189,2.43888142555952));
#71285=CARTESIAN_POINT('Ctrl Pts',(18.3,90.7547067344189,2.43888142555952));
#71286=CARTESIAN_POINT('Ctrl Pts',(18.3,90.702864998579,2.34174626916647));
#71287=CARTESIAN_POINT('Ctrl Pts',(18.3,90.605184161663,2.2784447953105));
#71288=CARTESIAN_POINT('',(18.18,90.7547067344189,2.43888142555952));
#71289=CARTESIAN_POINT('',(18.3,90.7547067344189,2.43888142555952));
#71290=CARTESIAN_POINT('Ctrl Pts',(18.18,90.7547067344189,2.43888142555952));
#71291=CARTESIAN_POINT('Ctrl Pts',(18.18,90.702864998579,2.34174626916647));
#71292=CARTESIAN_POINT('Ctrl Pts',(18.18,90.605184161663,2.2784447953105));
#71293=CARTESIAN_POINT('Ctrl Pts',(18.3,90.8065484702587,2.66480210274458));
#71294=CARTESIAN_POINT('Ctrl Pts',(18.1272,90.8065484702587,2.66480210274458));
#71295=CARTESIAN_POINT('Ctrl Pts',(18.3,90.8065484702587,2.53601643294096));
#71296=CARTESIAN_POINT('Ctrl Pts',(18.1272,90.8065484702587,2.53601643294096));
#71297=CARTESIAN_POINT('Ctrl Pts',(18.3,90.7547067344189,2.43888142555952));
#71298=CARTESIAN_POINT('Ctrl Pts',(18.1272,90.7547067344189,2.43888142555952));
#71299=CARTESIAN_POINT('',(18.3,90.8065484702587,2.66480210274458));
#71300=CARTESIAN_POINT('Ctrl Pts',(18.3,90.8065484702587,2.66480210274458));
#71301=CARTESIAN_POINT('Ctrl Pts',(18.3,90.8065484702587,2.53601643294096));
#71302=CARTESIAN_POINT('Ctrl Pts',(18.3,90.7547067344189,2.43888142555952));
#71303=CARTESIAN_POINT('',(18.18,90.8065484702587,2.66480210274458));
#71304=CARTESIAN_POINT('',(18.3,90.8065484702587,2.66480210274458));
#71305=CARTESIAN_POINT('Ctrl Pts',(18.18,90.8065484702587,2.66480210274458));
#71306=CARTESIAN_POINT('Ctrl Pts',(18.18,90.8065484702587,2.53601643294096));
#71307=CARTESIAN_POINT('Ctrl Pts',(18.18,90.7547067344189,2.43888142555952));
#71308=CARTESIAN_POINT('Ctrl Pts',(18.3,90.7126876950264,2.95457023233175));
#71309=CARTESIAN_POINT('Ctrl Pts',(18.1272,90.7126876950264,2.95457023233175));
#71310=CARTESIAN_POINT('Ctrl Pts',(18.3,90.8065484702587,2.83942702263594));
#71311=CARTESIAN_POINT('Ctrl Pts',(18.1272,90.8065484702587,2.83942702263594));
#71312=CARTESIAN_POINT('Ctrl Pts',(18.3,90.8065484702587,2.66480210274458));
#71313=CARTESIAN_POINT('Ctrl Pts',(18.1272,90.8065484702587,2.66480210274458));
#71314=CARTESIAN_POINT('',(18.3,90.7126876950264,2.95457023233175));
#71315=CARTESIAN_POINT('Ctrl Pts',(18.3,90.7126876950264,2.95457023233175));
#71316=CARTESIAN_POINT('Ctrl Pts',(18.3,90.8065484702587,2.83942702263594));
#71317=CARTESIAN_POINT('Ctrl Pts',(18.3,90.8065484702587,2.66480210274458));
#71318=CARTESIAN_POINT('',(18.18,90.7126876950264,2.95457023233175));
#71319=CARTESIAN_POINT('',(18.3,90.7126876950264,2.95457023233175));
#71320=CARTESIAN_POINT('Ctrl Pts',(18.18,90.7126876950264,2.95457023233175));
#71321=CARTESIAN_POINT('Ctrl Pts',(18.18,90.8065484702587,2.83942702263594));
#71322=CARTESIAN_POINT('Ctrl Pts',(18.18,90.8065484702587,2.66480210274458));
#71323=CARTESIAN_POINT('Ctrl Pts',(18.3,90.4458390414715,3.12810364216566));
#71324=CARTESIAN_POINT('Ctrl Pts',(18.1272,90.4458390414715,3.12810364216566));
#71325=CARTESIAN_POINT('Ctrl Pts',(18.3,90.6188267707825,3.06971344202757));
#71326=CARTESIAN_POINT('Ctrl Pts',(18.1272,90.6188267707825,3.06971344202757));
#71327=CARTESIAN_POINT('Ctrl Pts',(18.3,90.7126876950264,2.95457023233175));
#71328=CARTESIAN_POINT('Ctrl Pts',(18.1272,90.7126876950264,2.95457023233175));
#71329=CARTESIAN_POINT('',(18.3,90.4458390414715,3.12810364216566));
#71330=CARTESIAN_POINT('Ctrl Pts',(18.3,90.4458390414715,3.12810364216566));
#71331=CARTESIAN_POINT('Ctrl Pts',(18.3,90.6188267707825,3.06971344202757));
#71332=CARTESIAN_POINT('Ctrl Pts',(18.3,90.7126876950264,2.95457023233175));
#71333=CARTESIAN_POINT('',(18.18,90.4458390414715,3.12810364216566));
#71334=CARTESIAN_POINT('',(18.3,90.4458390414715,3.12810364216566));
#71335=CARTESIAN_POINT('Ctrl Pts',(18.18,90.4458390414715,3.12810364216566));
#71336=CARTESIAN_POINT('Ctrl Pts',(18.18,90.6188267707825,3.06971344202757));
#71337=CARTESIAN_POINT('Ctrl Pts',(18.18,90.7126876950264,2.95457023233175));
#71338=CARTESIAN_POINT('Ctrl Pts',(18.3,89.9890859663486,3.18649384230375));
#71339=CARTESIAN_POINT('Ctrl Pts',(18.1272,89.9890859663486,3.18649384230375));
#71340=CARTESIAN_POINT('Ctrl Pts',(18.3,90.2728513121605,3.18649384230375));
#71341=CARTESIAN_POINT('Ctrl Pts',(18.1272,90.2728513121605,3.18649384230375));
#71342=CARTESIAN_POINT('Ctrl Pts',(18.3,90.4458390414715,3.12810364216566));
#71343=CARTESIAN_POINT('Ctrl Pts',(18.1272,90.4458390414715,3.12810364216566));
#71344=CARTESIAN_POINT('',(18.3,89.9890859663486,3.18649384230375));
#71345=CARTESIAN_POINT('Ctrl Pts',(18.3,89.9890859663486,3.18649384230375));
#71346=CARTESIAN_POINT('Ctrl Pts',(18.3,90.2728513121605,3.18649384230375));
#71347=CARTESIAN_POINT('Ctrl Pts',(18.3,90.4458390414715,3.12810364216566));
#71348=CARTESIAN_POINT('',(18.18,89.9890859663486,3.18649384230375));
#71349=CARTESIAN_POINT('',(18.3,89.9890859663486,3.18649384230375));
#71350=CARTESIAN_POINT('Ctrl Pts',(18.18,89.9890859663486,3.18649384230375));
#71351=CARTESIAN_POINT('Ctrl Pts',(18.18,90.2728513121605,3.18649384230375));
#71352=CARTESIAN_POINT('Ctrl Pts',(18.18,90.4458390414715,3.12810364216566));
#71353=CARTESIAN_POINT('Ctrl Pts',(18.3,89.3386085569858,3.02824008315802));
#71354=CARTESIAN_POINT('Ctrl Pts',(18.1272,89.3386085569858,3.02824008315802));
#71355=CARTESIAN_POINT('Ctrl Pts',(18.3,89.5383356750011,3.18649384230375));
#71356=CARTESIAN_POINT('Ctrl Pts',(18.1272,89.5383356750011,3.18649384230375));
#71357=CARTESIAN_POINT('Ctrl Pts',(18.3,89.9890859663486,3.18649384230375));
#71358=CARTESIAN_POINT('Ctrl Pts',(18.1272,89.9890859663486,3.18649384230375));
#71359=CARTESIAN_POINT('Ctrl Pts',(18.3,89.3386085569858,3.02824008315802));
#71360=CARTESIAN_POINT('Ctrl Pts',(18.3,89.5383356750011,3.18649384230375));
#71361=CARTESIAN_POINT('Ctrl Pts',(18.3,89.9890859663486,3.18649384230375));
#71362=CARTESIAN_POINT('Ctrl Pts',(18.18,89.3386085569858,3.02824008315802));
#71363=CARTESIAN_POINT('Ctrl Pts',(18.18,89.5383356750011,3.18649384230375));
#71364=CARTESIAN_POINT('Ctrl Pts',(18.18,89.9890859663486,3.18649384230375));
#71365=CARTESIAN_POINT('Origin',(18.18,89.9896316468716,3.29999995455146));
#71366=CARTESIAN_POINT('Ctrl Pts',(18.3,89.4952251255512,4.09890851974487));
#71367=CARTESIAN_POINT('Ctrl Pts',(18.1272,89.4952251255512,4.09890851974487));
#71368=CARTESIAN_POINT('Ctrl Pts',(18.3,89.4422920286655,4.14911313951015));
#71369=CARTESIAN_POINT('Ctrl Pts',(18.1272,89.4422920286655,4.14911313951015));
#71370=CARTESIAN_POINT('Ctrl Pts',(18.3,89.3888132512569,4.18185527473688));
#71371=CARTESIAN_POINT('Ctrl Pts',(18.1272,89.3888132512569,4.18185527473688));
#71372=CARTESIAN_POINT('',(18.3,89.4952251255512,4.09890851974487));
#71373=CARTESIAN_POINT('',(18.3,89.3888132512569,4.18185527473688));
#71374=CARTESIAN_POINT('Ctrl Pts',(18.3,89.4952251255512,4.09890851974487));
#71375=CARTESIAN_POINT('Ctrl Pts',(18.3,89.4422920286655,4.14911313951015));
#71376=CARTESIAN_POINT('Ctrl Pts',(18.3,89.3888132512569,4.18185527473688));
#71377=CARTESIAN_POINT('',(18.18,89.4952251255512,4.09890851974487));
#71378=CARTESIAN_POINT('',(18.3,89.4952251255512,4.09890851974487));
#71379=CARTESIAN_POINT('',(18.18,89.3888132512569,4.18185527473688));
#71380=CARTESIAN_POINT('Ctrl Pts',(18.18,89.4952251255512,4.09890851974487));
#71381=CARTESIAN_POINT('Ctrl Pts',(18.18,89.4422920286655,4.14911313951015));
#71382=CARTESIAN_POINT('Ctrl Pts',(18.18,89.3888132512569,4.18185527473688));
#71383=CARTESIAN_POINT('',(18.3,89.3888132512569,4.18185527473688));
#71384=CARTESIAN_POINT('Ctrl Pts',(18.3,89.6965892851353,3.87189629524946));
#71385=CARTESIAN_POINT('Ctrl Pts',(18.1272,89.6965892851353,3.87189629524946));
#71386=CARTESIAN_POINT('Ctrl Pts',(18.3,89.5481582224369,4.04870386272669));
#71387=CARTESIAN_POINT('Ctrl Pts',(18.1272,89.5481582224369,4.04870386272669));
#71388=CARTESIAN_POINT('Ctrl Pts',(18.3,89.4952251255512,4.09890851974487));
#71389=CARTESIAN_POINT('Ctrl Pts',(18.1272,89.4952251255512,4.09890851974487));
#71390=CARTESIAN_POINT('',(18.3,89.6965892851353,3.87189629524946));
#71391=CARTESIAN_POINT('Ctrl Pts',(18.3,89.6965892851353,3.87189629524946));
#71392=CARTESIAN_POINT('Ctrl Pts',(18.3,89.5481582224369,4.04870386272669));
#71393=CARTESIAN_POINT('Ctrl Pts',(18.3,89.4952251255512,4.09890851974487));
#71394=CARTESIAN_POINT('',(18.18,89.6965892851353,3.87189629524946));
#71395=CARTESIAN_POINT('',(18.3,89.6965892851353,3.87189629524946));
#71396=CARTESIAN_POINT('Ctrl Pts',(18.18,89.6965892851353,3.87189629524946));
#71397=CARTESIAN_POINT('Ctrl Pts',(18.18,89.5481582224369,4.04870386272669));
#71398=CARTESIAN_POINT('Ctrl Pts',(18.18,89.4952251255512,4.09890851974487));
#71399=CARTESIAN_POINT('Ctrl Pts',(18.3,89.978172057867,3.5690313860774));
#71400=CARTESIAN_POINT('Ctrl Pts',(18.1272,89.978172057867,3.5690313860774));
#71401=CARTESIAN_POINT('Ctrl Pts',(18.3,89.8755799472332,3.66016360968351));
#71402=CARTESIAN_POINT('Ctrl Pts',(18.1272,89.8755799472332,3.66016360968351));
#71403=CARTESIAN_POINT('Ctrl Pts',(18.3,89.6965892851353,3.87189629524946));
#71404=CARTESIAN_POINT('Ctrl Pts',(18.1272,89.6965892851353,3.87189629524946));
#71405=CARTESIAN_POINT('',(18.3,89.978172057867,3.5690313860774));
#71406=CARTESIAN_POINT('Ctrl Pts',(18.3,89.978172057867,3.5690313860774));
#71407=CARTESIAN_POINT('Ctrl Pts',(18.3,89.8755799472332,3.66016360968351));
#71408=CARTESIAN_POINT('Ctrl Pts',(18.3,89.6965892851353,3.87189629524946));
#71409=CARTESIAN_POINT('',(18.18,89.978172057867,3.5690313860774));
#71410=CARTESIAN_POINT('',(18.3,89.978172057867,3.5690313860774));
#71411=CARTESIAN_POINT('Ctrl Pts',(18.18,89.978172057867,3.5690313860774));
#71412=CARTESIAN_POINT('Ctrl Pts',(18.18,89.8755799472332,3.66016360968351));
#71413=CARTESIAN_POINT('Ctrl Pts',(18.18,89.6965892851353,3.87189629524946));
#71414=CARTESIAN_POINT('Ctrl Pts',(18.3,90.1735334336758,3.4386083766818));
#71415=CARTESIAN_POINT('Ctrl Pts',(18.1272,90.1735334336758,3.4386083766818));
#71416=CARTESIAN_POINT('Ctrl Pts',(18.3,90.0807640194893,3.47789901345968));
#71417=CARTESIAN_POINT('Ctrl Pts',(18.1272,90.0807640194893,3.47789901345968));
#71418=CARTESIAN_POINT('Ctrl Pts',(18.3,89.978172057867,3.5690313860774));
#71419=CARTESIAN_POINT('Ctrl Pts',(18.1272,89.978172057867,3.5690313860774));
#71420=CARTESIAN_POINT('',(18.3,90.1735334336758,3.4386083766818));
#71421=CARTESIAN_POINT('Ctrl Pts',(18.3,90.1735334336758,3.4386083766818));
#71422=CARTESIAN_POINT('Ctrl Pts',(18.3,90.0807640194893,3.47789901345968));
#71423=CARTESIAN_POINT('Ctrl Pts',(18.3,89.978172057867,3.5690313860774));
#71424=CARTESIAN_POINT('',(18.18,90.1735334336758,3.4386083766818));
#71425=CARTESIAN_POINT('',(18.3,90.1735334336758,3.4386083766818));
#71426=CARTESIAN_POINT('Ctrl Pts',(18.18,90.1735334336758,3.4386083766818));
#71427=CARTESIAN_POINT('Ctrl Pts',(18.18,90.0807640194893,3.47789901345968));
#71428=CARTESIAN_POINT('Ctrl Pts',(18.18,89.978172057867,3.5690313860774));
#71429=CARTESIAN_POINT('Ctrl Pts',(18.3,90.3623466432094,3.39931788891554));
#71430=CARTESIAN_POINT('Ctrl Pts',(18.1272,90.3623466432094,3.39931788891554));
#71431=CARTESIAN_POINT('Ctrl Pts',(18.3,90.2663029968738,3.39931788891554));
#71432=CARTESIAN_POINT('Ctrl Pts',(18.1272,90.2663029968738,3.39931788891554));
#71433=CARTESIAN_POINT('Ctrl Pts',(18.3,90.1735334336758,3.4386083766818));
#71434=CARTESIAN_POINT('Ctrl Pts',(18.1272,90.1735334336758,3.4386083766818));
#71435=CARTESIAN_POINT('',(18.3,90.3623466432094,3.39931788891554));
#71436=CARTESIAN_POINT('Ctrl Pts',(18.3,90.3623466432094,3.39931788891554));
#71437=CARTESIAN_POINT('Ctrl Pts',(18.3,90.2663029968738,3.39931788891554));
#71438=CARTESIAN_POINT('Ctrl Pts',(18.3,90.1735334336758,3.4386083766818));
#71439=CARTESIAN_POINT('',(18.18,90.3623466432094,3.39931788891554));
#71440=CARTESIAN_POINT('',(18.3,90.3623466432094,3.39931788891554));
#71441=CARTESIAN_POINT('Ctrl Pts',(18.18,90.3623466432094,3.39931788891554));
#71442=CARTESIAN_POINT('Ctrl Pts',(18.18,90.2663029968738,3.39931788891554));
#71443=CARTESIAN_POINT('Ctrl Pts',(18.18,90.1735334336758,3.4386083766818));
#71444=CARTESIAN_POINT('Ctrl Pts',(18.3,90.6788541615009,3.53356066197157));
#71445=CARTESIAN_POINT('Ctrl Pts',(18.1272,90.6788541615009,3.53356066197157));
#71446=CARTESIAN_POINT('Ctrl Pts',(18.3,90.5511597037315,3.39931788891554));
#71447=CARTESIAN_POINT('Ctrl Pts',(18.1272,90.5511597037315,3.39931788891554));
#71448=CARTESIAN_POINT('Ctrl Pts',(18.3,90.3623466432094,3.39931788891554));
#71449=CARTESIAN_POINT('Ctrl Pts',(18.1272,90.3623466432094,3.39931788891554));
#71450=CARTESIAN_POINT('',(18.3,90.6788541615009,3.53356066197157));
#71451=CARTESIAN_POINT('Ctrl Pts',(18.3,90.6788541615009,3.53356066197157));
#71452=CARTESIAN_POINT('Ctrl Pts',(18.3,90.5511597037315,3.39931788891554));
#71453=CARTESIAN_POINT('Ctrl Pts',(18.3,90.3623466432094,3.39931788891554));
#71454=CARTESIAN_POINT('',(18.18,90.6788541615009,3.53356066197157));
#71455=CARTESIAN_POINT('',(18.3,90.6788541615009,3.53356066197157));
#71456=CARTESIAN_POINT('Ctrl Pts',(18.18,90.6788541615009,3.53356066197157));
#71457=CARTESIAN_POINT('Ctrl Pts',(18.18,90.5511597037315,3.39931788891554));
#71458=CARTESIAN_POINT('Ctrl Pts',(18.18,90.3623466432094,3.39931788891554));
#71459=CARTESIAN_POINT('Ctrl Pts',(18.3,90.8065484702587,3.89809000343084));
#71460=CARTESIAN_POINT('Ctrl Pts',(18.1272,90.8065484702587,3.89809000343084));
#71461=CARTESIAN_POINT('Ctrl Pts',(18.3,90.8065484702587,3.6678034350276));
#71462=CARTESIAN_POINT('Ctrl Pts',(18.1272,90.8065484702587,3.6678034350276));
#71463=CARTESIAN_POINT('Ctrl Pts',(18.3,90.6788541615009,3.53356066197157));
#71464=CARTESIAN_POINT('Ctrl Pts',(18.1272,90.6788541615009,3.53356066197157));
#71465=CARTESIAN_POINT('',(18.3,90.8065484702587,3.89809000343084));
#71466=CARTESIAN_POINT('Ctrl Pts',(18.3,90.8065484702587,3.89809000343084));
#71467=CARTESIAN_POINT('Ctrl Pts',(18.3,90.8065484702587,3.6678034350276));
#71468=CARTESIAN_POINT('Ctrl Pts',(18.3,90.6788541615009,3.53356066197157));
#71469=CARTESIAN_POINT('',(18.18,90.8065484702587,3.89809000343084));
#71470=CARTESIAN_POINT('',(18.3,90.8065484702587,3.89809000343084));
#71471=CARTESIAN_POINT('Ctrl Pts',(18.18,90.8065484702587,3.89809000343084));
#71472=CARTESIAN_POINT('Ctrl Pts',(18.18,90.8065484702587,3.6678034350276));
#71473=CARTESIAN_POINT('Ctrl Pts',(18.18,90.6788541615009,3.53356066197157));
#71474=CARTESIAN_POINT('Ctrl Pts',(18.3,90.6881310284138,4.26152787208557));
#71475=CARTESIAN_POINT('Ctrl Pts',(18.1272,90.6881310284138,4.26152787208557));
#71476=CARTESIAN_POINT('Ctrl Pts',(18.3,90.8065484702587,4.12619362622499));
#71477=CARTESIAN_POINT('Ctrl Pts',(18.1272,90.8065484702587,4.12619362622499));
#71478=CARTESIAN_POINT('Ctrl Pts',(18.3,90.8065484702587,3.89809000343084));
#71479=CARTESIAN_POINT('Ctrl Pts',(18.1272,90.8065484702587,3.89809000343084));
#71480=CARTESIAN_POINT('',(18.3,90.6881310284138,4.26152787208557));
#71481=CARTESIAN_POINT('Ctrl Pts',(18.3,90.6881310284138,4.26152787208557));
#71482=CARTESIAN_POINT('Ctrl Pts',(18.3,90.8065484702587,4.12619362622499));
#71483=CARTESIAN_POINT('Ctrl Pts',(18.3,90.8065484702587,3.89809000343084));
#71484=CARTESIAN_POINT('',(18.18,90.6881310284138,4.26152787208557));
#71485=CARTESIAN_POINT('',(18.3,90.6881310284138,4.26152787208557));
#71486=CARTESIAN_POINT('Ctrl Pts',(18.18,90.6881310284138,4.26152787208557));
#71487=CARTESIAN_POINT('Ctrl Pts',(18.18,90.8065484702587,4.12619362622499));
#71488=CARTESIAN_POINT('Ctrl Pts',(18.18,90.8065484702587,3.89809000343084));
#71489=CARTESIAN_POINT('Ctrl Pts',(18.3,90.3437926113605,4.41759881600738));
#71490=CARTESIAN_POINT('Ctrl Pts',(18.1272,90.3437926113605,4.41759881600738));
#71491=CARTESIAN_POINT('Ctrl Pts',(18.3,90.5697135865688,4.39686211794615));
#71492=CARTESIAN_POINT('Ctrl Pts',(18.1272,90.5697135865688,4.39686211794615));
#71493=CARTESIAN_POINT('Ctrl Pts',(18.3,90.6881310284138,4.26152787208557));
#71494=CARTESIAN_POINT('Ctrl Pts',(18.1272,90.6881310284138,4.26152787208557));
#71495=CARTESIAN_POINT('',(18.3,90.3437926113605,4.41759881600738));
#71496=CARTESIAN_POINT('Ctrl Pts',(18.3,90.3437926113605,4.41759881600738));
#71497=CARTESIAN_POINT('Ctrl Pts',(18.3,90.5697135865688,4.39686211794615));
#71498=CARTESIAN_POINT('Ctrl Pts',(18.3,90.6881310284138,4.26152787208557));
#71499=CARTESIAN_POINT('',(18.18,90.3437926113605,4.41759881600738));
#71500=CARTESIAN_POINT('',(18.3,90.3437926113605,4.41759881600738));
#71501=CARTESIAN_POINT('Ctrl Pts',(18.18,90.3437926113605,4.41759881600738));
#71502=CARTESIAN_POINT('Ctrl Pts',(18.18,90.5697135865688,4.39686211794615));
#71503=CARTESIAN_POINT('Ctrl Pts',(18.18,90.6881310284138,4.26152787208557));
#71504=CARTESIAN_POINT('Origin',(18.3,90.3230560064316,4.21568888276815));
#71505=CARTESIAN_POINT('',(18.3,90.3230560064316,4.21568888276815));
#71506=CARTESIAN_POINT('',(18.3,90.2822558942559,3.8184228908779));
#71507=CARTESIAN_POINT('',(18.18,90.3230560064316,4.21568888276815));
#71508=CARTESIAN_POINT('',(18.3,90.3230560064316,4.21568888276815));
#71509=CARTESIAN_POINT('',(18.18,90.3230560064316,4.21568888276815));
#71510=CARTESIAN_POINT('Ctrl Pts',(18.3,90.5587995290756,4.12946785837412));
#71511=CARTESIAN_POINT('Ctrl Pts',(18.1272,90.5587995290756,4.12946785837412));
#71512=CARTESIAN_POINT('Ctrl Pts',(18.3,90.4736699402332,4.21459744721651));
#71513=CARTESIAN_POINT('Ctrl Pts',(18.1272,90.4736699402332,4.21459744721651));
#71514=CARTESIAN_POINT('Ctrl Pts',(18.3,90.3230560064316,4.21568888276815));
#71515=CARTESIAN_POINT('Ctrl Pts',(18.1272,90.3230560064316,4.21568888276815));
#71516=CARTESIAN_POINT('',(18.3,90.5587995290756,4.12946785837412));
#71517=CARTESIAN_POINT('Ctrl Pts',(18.3,90.5587995290756,4.12946785837412));
#71518=CARTESIAN_POINT('Ctrl Pts',(18.3,90.4736699402332,4.21459744721651));
#71519=CARTESIAN_POINT('Ctrl Pts',(18.3,90.3230560064316,4.21568888276815));
#71520=CARTESIAN_POINT('',(18.18,90.5587995290756,4.12946785837412));
#71521=CARTESIAN_POINT('',(18.3,90.5587995290756,4.12946785837412));
#71522=CARTESIAN_POINT('Ctrl Pts',(18.18,90.5587995290756,4.12946785837412));
#71523=CARTESIAN_POINT('Ctrl Pts',(18.18,90.4736699402332,4.21459744721651));
#71524=CARTESIAN_POINT('Ctrl Pts',(18.18,90.3230560064316,4.21568888276815));
#71525=CARTESIAN_POINT('Ctrl Pts',(18.3,90.643929117918,3.9024555966258));
#71526=CARTESIAN_POINT('Ctrl Pts',(18.1272,90.643929117918,3.9024555966258));
#71527=CARTESIAN_POINT('Ctrl Pts',(18.3,90.643929117918,4.04433826953173));
#71528=CARTESIAN_POINT('Ctrl Pts',(18.1272,90.643929117918,4.04433826953173));
#71529=CARTESIAN_POINT('Ctrl Pts',(18.3,90.5587995290756,4.12946785837412));
#71530=CARTESIAN_POINT('Ctrl Pts',(18.1272,90.5587995290756,4.12946785837412));
#71531=CARTESIAN_POINT('',(18.3,90.643929117918,3.9024555966258));
#71532=CARTESIAN_POINT('Ctrl Pts',(18.3,90.643929117918,3.9024555966258));
#71533=CARTESIAN_POINT('Ctrl Pts',(18.3,90.643929117918,4.04433826953173));
#71534=CARTESIAN_POINT('Ctrl Pts',(18.3,90.5587995290756,4.12946785837412));
#71535=CARTESIAN_POINT('',(18.18,90.643929117918,3.9024555966258));
#71536=CARTESIAN_POINT('',(18.3,90.643929117918,3.9024555966258));
#71537=CARTESIAN_POINT('Ctrl Pts',(18.18,90.643929117918,3.9024555966258));
#71538=CARTESIAN_POINT('Ctrl Pts',(18.18,90.643929117918,4.04433826953173));
#71539=CARTESIAN_POINT('Ctrl Pts',(18.18,90.5587995290756,4.12946785837412));
#71540=CARTESIAN_POINT('Ctrl Pts',(18.3,90.5637108027935,3.68472027629614));
#71541=CARTESIAN_POINT('Ctrl Pts',(18.1272,90.5637108027935,3.68472027629614));
#71542=CARTESIAN_POINT('Ctrl Pts',(18.3,90.643929117918,3.76821282356977));
#71543=CARTESIAN_POINT('Ctrl Pts',(18.1272,90.643929117918,3.76821282356977));
#71544=CARTESIAN_POINT('Ctrl Pts',(18.3,90.643929117918,3.9024555966258));
#71545=CARTESIAN_POINT('Ctrl Pts',(18.1272,90.643929117918,3.9024555966258));
#71546=CARTESIAN_POINT('',(18.3,90.5637108027935,3.68472027629614));
#71547=CARTESIAN_POINT('Ctrl Pts',(18.3,90.5637108027935,3.68472027629614));
#71548=CARTESIAN_POINT('Ctrl Pts',(18.3,90.643929117918,3.76821282356977));
#71549=CARTESIAN_POINT('Ctrl Pts',(18.3,90.643929117918,3.9024555966258));
#71550=CARTESIAN_POINT('',(18.18,90.5637108027935,3.68472027629614));
#71551=CARTESIAN_POINT('',(18.3,90.5637108027935,3.68472027629614));
#71552=CARTESIAN_POINT('Ctrl Pts',(18.18,90.5637108027935,3.68472027629614));
#71553=CARTESIAN_POINT('Ctrl Pts',(18.18,90.643929117918,3.76821282356977));
#71554=CARTESIAN_POINT('Ctrl Pts',(18.18,90.643929117918,3.9024555966258));
#71555=CARTESIAN_POINT('Ctrl Pts',(18.3,90.3667122364044,3.6012277290225));
#71556=CARTESIAN_POINT('Ctrl Pts',(18.1272,90.3667122364044,3.6012277290225));
#71557=CARTESIAN_POINT('Ctrl Pts',(18.3,90.4834926366806,3.6012277290225));
#71558=CARTESIAN_POINT('Ctrl Pts',(18.1272,90.4834926366806,3.6012277290225));
#71559=CARTESIAN_POINT('Ctrl Pts',(18.3,90.5637108027935,3.68472027629614));
#71560=CARTESIAN_POINT('Ctrl Pts',(18.1272,90.5637108027935,3.68472027629614));
#71561=CARTESIAN_POINT('',(18.3,90.3667122364044,3.6012277290225));
#71562=CARTESIAN_POINT('Ctrl Pts',(18.3,90.3667122364044,3.6012277290225));
#71563=CARTESIAN_POINT('Ctrl Pts',(18.3,90.4834926366806,3.6012277290225));
#71564=CARTESIAN_POINT('Ctrl Pts',(18.3,90.5637108027935,3.68472027629614));
#71565=CARTESIAN_POINT('',(18.18,90.3667122364044,3.6012277290225));
#71566=CARTESIAN_POINT('',(18.3,90.3667122364044,3.6012277290225));
#71567=CARTESIAN_POINT('Ctrl Pts',(18.18,90.3667122364044,3.6012277290225));
#71568=CARTESIAN_POINT('Ctrl Pts',(18.18,90.4834926366806,3.6012277290225));
#71569=CARTESIAN_POINT('Ctrl Pts',(18.18,90.5637108027935,3.68472027629614));
#71570=CARTESIAN_POINT('Ctrl Pts',(18.3,90.1304228842258,3.69290578216314));
#71571=CARTESIAN_POINT('Ctrl Pts',(18.1272,90.1304228842258,3.69290578216314));
#71572=CARTESIAN_POINT('Ctrl Pts',(18.3,90.255388790369,3.6012277290225));
#71573=CARTESIAN_POINT('Ctrl Pts',(18.1272,90.255388790369,3.6012277290225));
#71574=CARTESIAN_POINT('Ctrl Pts',(18.3,90.3667122364044,3.6012277290225));
#71575=CARTESIAN_POINT('Ctrl Pts',(18.1272,90.3667122364044,3.6012277290225));
#71576=CARTESIAN_POINT('',(18.3,90.1304228842258,3.69290578216314));
#71577=CARTESIAN_POINT('Ctrl Pts',(18.3,90.1304228842258,3.69290578216314));
#71578=CARTESIAN_POINT('Ctrl Pts',(18.3,90.255388790369,3.6012277290225));
#71579=CARTESIAN_POINT('Ctrl Pts',(18.3,90.3667122364044,3.6012277290225));
#71580=CARTESIAN_POINT('',(18.18,90.1304228842258,3.69290578216314));
#71581=CARTESIAN_POINT('',(18.3,90.1304228842258,3.69290578216314));
#71582=CARTESIAN_POINT('Ctrl Pts',(18.18,90.1304228842258,3.69290578216314));
#71583=CARTESIAN_POINT('Ctrl Pts',(18.18,90.255388790369,3.6012277290225));
#71584=CARTESIAN_POINT('Ctrl Pts',(18.18,90.3667122364044,3.6012277290225));
#71585=CARTESIAN_POINT('Ctrl Pts',(18.3,89.791541570425,4.04542966783047));
#71586=CARTESIAN_POINT('Ctrl Pts',(18.1272,89.791541570425,4.04542966783047));
#71587=CARTESIAN_POINT('Ctrl Pts',(18.3,90.0054569780826,3.78458383530378));
#71588=CARTESIAN_POINT('Ctrl Pts',(18.1272,90.0054569780826,3.78458383530378));
#71589=CARTESIAN_POINT('Ctrl Pts',(18.3,90.1304228842258,3.69290578216314));
#71590=CARTESIAN_POINT('Ctrl Pts',(18.1272,90.1304228842258,3.69290578216314));
#71591=CARTESIAN_POINT('',(18.3,89.791541570425,4.04542966783047));
#71592=CARTESIAN_POINT('Ctrl Pts',(18.3,89.791541570425,4.04542966783047));
#71593=CARTESIAN_POINT('Ctrl Pts',(18.3,90.0054569780826,3.78458383530378));
#71594=CARTESIAN_POINT('Ctrl Pts',(18.3,90.1304228842258,3.69290578216314));
#71595=CARTESIAN_POINT('',(18.18,89.791541570425,4.04542966783047));
#71596=CARTESIAN_POINT('',(18.3,89.791541570425,4.04542966783047));
#71597=CARTESIAN_POINT('Ctrl Pts',(18.18,89.791541570425,4.04542966783047));
#71598=CARTESIAN_POINT('Ctrl Pts',(18.18,90.0054569780826,3.78458383530378));
#71599=CARTESIAN_POINT('Ctrl Pts',(18.18,90.1304228842258,3.69290578216314));
#71600=CARTESIAN_POINT('Ctrl Pts',(18.3,89.5492495834827,4.30245558768511));
#71601=CARTESIAN_POINT('Ctrl Pts',(18.1272,89.5492495834827,4.30245558768511));
#71602=CARTESIAN_POINT('Ctrl Pts',(18.3,89.6540247142315,4.21350604891777));
#71603=CARTESIAN_POINT('Ctrl Pts',(18.1272,89.6540247142315,4.21350604891777));
#71604=CARTESIAN_POINT('Ctrl Pts',(18.3,89.791541570425,4.04542966783047));
#71605=CARTESIAN_POINT('Ctrl Pts',(18.1272,89.791541570425,4.04542966783047));
#71606=CARTESIAN_POINT('',(18.3,89.5492495834827,4.30245558768511));
#71607=CARTESIAN_POINT('Ctrl Pts',(18.3,89.5492495834827,4.30245558768511));
#71608=CARTESIAN_POINT('Ctrl Pts',(18.3,89.6540247142315,4.21350604891777));
#71609=CARTESIAN_POINT('Ctrl Pts',(18.3,89.791541570425,4.04542966783047));
#71610=CARTESIAN_POINT('',(18.18,89.5492495834827,4.30245558768511));
#71611=CARTESIAN_POINT('',(18.3,89.5492495834827,4.30245558768511));
#71612=CARTESIAN_POINT('Ctrl Pts',(18.18,89.5492495834827,4.30245558768511));
#71613=CARTESIAN_POINT('Ctrl Pts',(18.18,89.6540247142315,4.21350604891777));
#71614=CARTESIAN_POINT('Ctrl Pts',(18.18,89.791541570425,4.04542966783047));
#71615=CARTESIAN_POINT('Ctrl Pts',(18.3,89.3364258348942,4.43178708702326));
#71616=CARTESIAN_POINT('Ctrl Pts',(18.1272,89.3364258348942,4.43178708702326));
#71617=CARTESIAN_POINT('Ctrl Pts',(18.3,89.4444747507572,4.39140508919954));
#71618=CARTESIAN_POINT('Ctrl Pts',(18.1272,89.4444747507572,4.39140508919954));
#71619=CARTESIAN_POINT('Ctrl Pts',(18.3,89.5492495834827,4.30245558768511));
#71620=CARTESIAN_POINT('Ctrl Pts',(18.1272,89.5492495834827,4.30245558768511));
#71621=CARTESIAN_POINT('',(18.3,89.3364258348942,4.43178708702326));
#71622=CARTESIAN_POINT('Ctrl Pts',(18.3,89.3364258348942,4.43178708702326));
#71623=CARTESIAN_POINT('Ctrl Pts',(18.3,89.4444747507572,4.39140508919954));
#71624=CARTESIAN_POINT('Ctrl Pts',(18.3,89.5492495834827,4.30245558768511));
#71625=CARTESIAN_POINT('',(18.18,89.3364258348942,4.43178708702326));
#71626=CARTESIAN_POINT('',(18.3,89.3364258348942,4.43178708702326));
#71627=CARTESIAN_POINT('Ctrl Pts',(18.18,89.3364258348942,4.43178708702326));
#71628=CARTESIAN_POINT('Ctrl Pts',(18.18,89.4444747507572,4.39140508919954));
#71629=CARTESIAN_POINT('Ctrl Pts',(18.18,89.5492495834827,4.30245558768511));
#71630=CARTESIAN_POINT('Ctrl Pts',(18.3,89.2000000417232,4.45470658168197));
#71631=CARTESIAN_POINT('Ctrl Pts',(18.1272,89.2000000417232,4.45470658168197));
#71632=CARTESIAN_POINT('Ctrl Pts',(18.3,89.2709414899349,4.4568893969059));
#71633=CARTESIAN_POINT('Ctrl Pts',(18.1272,89.2709414899349,4.4568893969059));
#71634=CARTESIAN_POINT('Ctrl Pts',(18.3,89.3364258348942,4.43178708702326));
#71635=CARTESIAN_POINT('Ctrl Pts',(18.1272,89.3364258348942,4.43178708702326));
#71636=CARTESIAN_POINT('',(18.3,89.2000000417232,4.45470658168197));
#71637=CARTESIAN_POINT('Ctrl Pts',(18.3,89.2000000417232,4.45470658168197));
#71638=CARTESIAN_POINT('Ctrl Pts',(18.3,89.2709414899349,4.4568893969059));
#71639=CARTESIAN_POINT('Ctrl Pts',(18.3,89.3364258348942,4.43178708702326));
#71640=CARTESIAN_POINT('',(18.18,89.2000000417232,4.45470658168197));
#71641=CARTESIAN_POINT('',(18.3,89.2000000417232,4.45470658168197));
#71642=CARTESIAN_POINT('Ctrl Pts',(18.18,89.2000000417232,4.45470658168197));
#71643=CARTESIAN_POINT('Ctrl Pts',(18.18,89.2709414899349,4.4568893969059));
#71644=CARTESIAN_POINT('Ctrl Pts',(18.18,89.3364258348942,4.43178708702326));
#71645=CARTESIAN_POINT('Origin',(18.3,89.2000000417232,3.39713501781225));
#71646=CARTESIAN_POINT('',(18.3,89.2000000417232,3.39713501781225));
#71647=CARTESIAN_POINT('',(18.3,89.2000000417232,4.44856750890613));
#71648=CARTESIAN_POINT('',(18.18,89.2000000417232,3.39713501781225));
#71649=CARTESIAN_POINT('',(18.3,89.2000000417232,3.39713501781225));
#71650=CARTESIAN_POINT('',(18.18,89.2000000417232,3.39713501781225));
#71651=CARTESIAN_POINT('Origin',(18.3,89.3888132512569,3.39713501781225));
#71652=CARTESIAN_POINT('',(18.3,89.3888132512569,3.39713501781225));
#71653=CARTESIAN_POINT('',(18.3,79.6944066256285,3.39713501781225));
#71654=CARTESIAN_POINT('',(18.18,89.3888132512569,3.39713501781225));
#71655=CARTESIAN_POINT('',(18.3,89.3888132512569,3.39713501781225));
#71656=CARTESIAN_POINT('',(18.18,89.3888132512569,3.39713501781225));
#71657=CARTESIAN_POINT('Origin',(18.3,89.3888132512569,4.18185527473688));
#71658=CARTESIAN_POINT('',(18.3,89.3888132512569,4.84092763736844));
#71659=CARTESIAN_POINT('',(18.18,89.3888132512569,4.18185527473688));
#71660=CARTESIAN_POINT('Origin',(18.18,89.9896316468716,3.29999995455146));
#71661=CARTESIAN_POINT('Origin',(18.3,70.,5.5));
#71662=CARTESIAN_POINT('Ctrl Pts',(18.3,80.643929117918,2.7559345126152));
#71663=CARTESIAN_POINT('Ctrl Pts',(18.1272,80.643929117918,2.7559345126152));
#71664=CARTESIAN_POINT('Ctrl Pts',(18.3,80.643929117918,2.89126879572868));
#71665=CARTESIAN_POINT('Ctrl Pts',(18.1272,80.643929117918,2.89126879572868));
#71666=CARTESIAN_POINT('Ctrl Pts',(18.3,80.5293315887451,2.97203279137611));
#71667=CARTESIAN_POINT('Ctrl Pts',(18.1272,80.5293315887451,2.97203279137611));
#71668=CARTESIAN_POINT('',(18.3,80.643929117918,2.7559345126152));
#71669=CARTESIAN_POINT('',(18.3,80.5293315887451,2.97203279137611));
#71670=CARTESIAN_POINT('Ctrl Pts',(18.3,80.643929117918,2.7559345126152));
#71671=CARTESIAN_POINT('Ctrl Pts',(18.3,80.643929117918,2.89126879572868));
#71672=CARTESIAN_POINT('Ctrl Pts',(18.3,80.5293315887451,2.97203279137611));
#71673=CARTESIAN_POINT('',(18.18,80.643929117918,2.7559345126152));
#71674=CARTESIAN_POINT('',(18.3,80.643929117918,2.7559345126152));
#71675=CARTESIAN_POINT('',(18.18,80.5293315887451,2.97203279137611));
#71676=CARTESIAN_POINT('Ctrl Pts',(18.18,80.643929117918,2.7559345126152));
#71677=CARTESIAN_POINT('Ctrl Pts',(18.18,80.643929117918,2.89126879572868));
#71678=CARTESIAN_POINT('Ctrl Pts',(18.18,80.5293315887451,2.97203279137611));
#71679=CARTESIAN_POINT('',(18.3,80.5293315887451,2.97203279137611));
#71680=CARTESIAN_POINT('Ctrl Pts',(18.3,80.5140519380569,2.52619377374649));
#71681=CARTESIAN_POINT('Ctrl Pts',(18.1272,80.5140519380569,2.52619377374649));
#71682=CARTESIAN_POINT('Ctrl Pts',(18.3,80.643929117918,2.61841750741005));
#71683=CARTESIAN_POINT('Ctrl Pts',(18.1272,80.643929117918,2.61841750741005));
#71684=CARTESIAN_POINT('Ctrl Pts',(18.3,80.643929117918,2.7559345126152));
#71685=CARTESIAN_POINT('Ctrl Pts',(18.1272,80.643929117918,2.7559345126152));
#71686=CARTESIAN_POINT('',(18.3,80.5140519380569,2.52619377374649));
#71687=CARTESIAN_POINT('Ctrl Pts',(18.3,80.5140519380569,2.52619377374649));
#71688=CARTESIAN_POINT('Ctrl Pts',(18.3,80.643929117918,2.61841750741005));
#71689=CARTESIAN_POINT('Ctrl Pts',(18.3,80.643929117918,2.7559345126152));
#71690=CARTESIAN_POINT('',(18.18,80.5140519380569,2.52619377374649));
#71691=CARTESIAN_POINT('',(18.3,80.5140519380569,2.52619377374649));
#71692=CARTESIAN_POINT('Ctrl Pts',(18.18,80.5140519380569,2.52619377374649));
#71693=CARTESIAN_POINT('Ctrl Pts',(18.18,80.643929117918,2.61841750741005));
#71694=CARTESIAN_POINT('Ctrl Pts',(18.18,80.643929117918,2.7559345126152));
#71695=CARTESIAN_POINT('Ctrl Pts',(18.3,79.9890859663486,2.43397004008293));
#71696=CARTESIAN_POINT('Ctrl Pts',(18.1272,79.9890859663486,2.43397004008293));
#71697=CARTESIAN_POINT('Ctrl Pts',(18.3,80.3841746091843,2.43397004008293));
#71698=CARTESIAN_POINT('Ctrl Pts',(18.1272,80.3841746091843,2.43397004008293));
#71699=CARTESIAN_POINT('Ctrl Pts',(18.3,80.5140519380569,2.52619377374649));
#71700=CARTESIAN_POINT('Ctrl Pts',(18.1272,80.5140519380569,2.52619377374649));
#71701=CARTESIAN_POINT('',(18.3,79.9890859663486,2.43397004008293));
#71702=CARTESIAN_POINT('Ctrl Pts',(18.3,79.9890859663486,2.43397004008293));
#71703=CARTESIAN_POINT('Ctrl Pts',(18.3,80.3841746091843,2.43397004008293));
#71704=CARTESIAN_POINT('Ctrl Pts',(18.3,80.5140519380569,2.52619377374649));
#71705=CARTESIAN_POINT('',(18.18,79.9890859663486,2.43397004008293));
#71706=CARTESIAN_POINT('',(18.3,79.9890859663486,2.43397004008293));
#71707=CARTESIAN_POINT('Ctrl Pts',(18.18,79.9890859663486,2.43397004008293));
#71708=CARTESIAN_POINT('Ctrl Pts',(18.18,80.3841746091843,2.43397004008293));
#71709=CARTESIAN_POINT('Ctrl Pts',(18.18,80.5140519380569,2.52619377374649));
#71710=CARTESIAN_POINT('Ctrl Pts',(18.3,79.4652115046978,2.52619377374649));
#71711=CARTESIAN_POINT('Ctrl Pts',(18.1272,79.4652115046978,2.52619377374649));
#71712=CARTESIAN_POINT('Ctrl Pts',(18.3,79.5961801946163,2.43397004008293));
#71713=CARTESIAN_POINT('Ctrl Pts',(18.1272,79.5961801946163,2.43397004008293));
#71714=CARTESIAN_POINT('Ctrl Pts',(18.3,79.9890859663486,2.43397004008293));
#71715=CARTESIAN_POINT('Ctrl Pts',(18.1272,79.9890859663486,2.43397004008293));
#71716=CARTESIAN_POINT('',(18.3,79.4652115046978,2.52619377374649));
#71717=CARTESIAN_POINT('Ctrl Pts',(18.3,79.4652115046978,2.52619377374649));
#71718=CARTESIAN_POINT('Ctrl Pts',(18.3,79.5961801946163,2.43397004008293));
#71719=CARTESIAN_POINT('Ctrl Pts',(18.3,79.9890859663486,2.43397004008293));
#71720=CARTESIAN_POINT('',(18.18,79.4652115046978,2.52619377374649));
#71721=CARTESIAN_POINT('',(18.3,79.4652115046978,2.52619377374649));
#71722=CARTESIAN_POINT('Ctrl Pts',(18.18,79.4652115046978,2.52619377374649));
#71723=CARTESIAN_POINT('Ctrl Pts',(18.18,79.5961801946163,2.43397004008293));
#71724=CARTESIAN_POINT('Ctrl Pts',(18.18,79.9890859663486,2.43397004008293));
#71725=CARTESIAN_POINT('Ctrl Pts',(18.3,79.3342428147793,2.75375164151192));
#71726=CARTESIAN_POINT('Ctrl Pts',(18.1272,79.3342428147793,2.75375164151192));
#71727=CARTESIAN_POINT('Ctrl Pts',(18.3,79.3342428147793,2.61841750741005));
#71728=CARTESIAN_POINT('Ctrl Pts',(18.1272,79.3342428147793,2.61841750741005));
#71729=CARTESIAN_POINT('Ctrl Pts',(18.3,79.4652115046978,2.52619377374649));
#71730=CARTESIAN_POINT('Ctrl Pts',(18.1272,79.4652115046978,2.52619377374649));
#71731=CARTESIAN_POINT('',(18.3,79.3342428147793,2.75375164151192));
#71732=CARTESIAN_POINT('Ctrl Pts',(18.3,79.3342428147793,2.75375164151192));
#71733=CARTESIAN_POINT('Ctrl Pts',(18.3,79.3342428147793,2.61841750741005));
#71734=CARTESIAN_POINT('Ctrl Pts',(18.3,79.4652115046978,2.52619377374649));
#71735=CARTESIAN_POINT('',(18.18,79.3342428147793,2.75375164151192));
#71736=CARTESIAN_POINT('',(18.3,79.3342428147793,2.75375164151192));
#71737=CARTESIAN_POINT('Ctrl Pts',(18.18,79.3342428147793,2.75375164151192));
#71738=CARTESIAN_POINT('Ctrl Pts',(18.18,79.3342428147793,2.61841750741005));
#71739=CARTESIAN_POINT('Ctrl Pts',(18.18,79.4652115046978,2.52619377374649));
#71740=CARTESIAN_POINT('Ctrl Pts',(18.3,79.4646658241749,2.98130965828896));
#71741=CARTESIAN_POINT('Ctrl Pts',(18.1272,79.4646658241749,2.98130965828896));
#71742=CARTESIAN_POINT('Ctrl Pts',(18.3,79.3342428147793,2.8890859246254));
#71743=CARTESIAN_POINT('Ctrl Pts',(18.1272,79.3342428147793,2.8890859246254));
#71744=CARTESIAN_POINT('Ctrl Pts',(18.3,79.3342428147793,2.75375164151192));
#71745=CARTESIAN_POINT('Ctrl Pts',(18.1272,79.3342428147793,2.75375164151192));
#71746=CARTESIAN_POINT('',(18.3,79.4646658241749,2.98130965828896));
#71747=CARTESIAN_POINT('Ctrl Pts',(18.3,79.4646658241749,2.98130965828896));
#71748=CARTESIAN_POINT('Ctrl Pts',(18.3,79.3342428147793,2.8890859246254));
#71749=CARTESIAN_POINT('Ctrl Pts',(18.3,79.3342428147793,2.75375164151192));
#71750=CARTESIAN_POINT('',(18.18,79.4646658241749,2.98130965828896));
#71751=CARTESIAN_POINT('',(18.3,79.4646658241749,2.98130965828896));
#71752=CARTESIAN_POINT('Ctrl Pts',(18.18,79.4646658241749,2.98130965828896));
#71753=CARTESIAN_POINT('Ctrl Pts',(18.18,79.3342428147793,2.8890859246254));
#71754=CARTESIAN_POINT('Ctrl Pts',(18.18,79.3342428147793,2.75375164151192));
#71755=CARTESIAN_POINT('Ctrl Pts',(18.3,79.9890859663486,3.07353339195251));
#71756=CARTESIAN_POINT('Ctrl Pts',(18.1272,79.9890859663486,3.07353339195251));
#71757=CARTESIAN_POINT('Ctrl Pts',(18.3,79.5950888335705,3.07353339195251));
#71758=CARTESIAN_POINT('Ctrl Pts',(18.1272,79.5950888335705,3.07353339195251));
#71759=CARTESIAN_POINT('Ctrl Pts',(18.3,79.4646658241749,2.98130965828896));
#71760=CARTESIAN_POINT('Ctrl Pts',(18.1272,79.4646658241749,2.98130965828896));
#71761=CARTESIAN_POINT('',(18.3,79.9890859663486,3.07353339195251));
#71762=CARTESIAN_POINT('Ctrl Pts',(18.3,79.9890859663486,3.07353339195251));
#71763=CARTESIAN_POINT('Ctrl Pts',(18.3,79.5950888335705,3.07353339195251));
#71764=CARTESIAN_POINT('Ctrl Pts',(18.3,79.4646658241749,2.98130965828896));
#71765=CARTESIAN_POINT('',(18.18,79.9890859663486,3.07353339195251));
#71766=CARTESIAN_POINT('',(18.3,79.9890859663486,3.07353339195251));
#71767=CARTESIAN_POINT('Ctrl Pts',(18.18,79.9890859663486,3.07353339195251));
#71768=CARTESIAN_POINT('Ctrl Pts',(18.18,79.5950888335705,3.07353339195251));
#71769=CARTESIAN_POINT('Ctrl Pts',(18.18,79.4646658241749,2.98130965828896));
#71770=CARTESIAN_POINT('Ctrl Pts',(18.3,80.5293315887451,2.97203279137611));
#71771=CARTESIAN_POINT('Ctrl Pts',(18.1272,80.5293315887451,2.97203279137611));
#71772=CARTESIAN_POINT('Ctrl Pts',(18.3,80.3830830991268,3.07353339195251));
#71773=CARTESIAN_POINT('Ctrl Pts',(18.1272,80.3830830991268,3.07353339195251));
#71774=CARTESIAN_POINT('Ctrl Pts',(18.3,79.9890859663486,3.07353339195251));
#71775=CARTESIAN_POINT('Ctrl Pts',(18.1272,79.9890859663486,3.07353339195251));
#71776=CARTESIAN_POINT('Ctrl Pts',(18.3,80.5293315887451,2.97203279137611));
#71777=CARTESIAN_POINT('Ctrl Pts',(18.3,80.3830830991268,3.07353339195251));
#71778=CARTESIAN_POINT('Ctrl Pts',(18.3,79.9890859663486,3.07353339195251));
#71779=CARTESIAN_POINT('Ctrl Pts',(18.18,80.5293315887451,2.97203279137611));
#71780=CARTESIAN_POINT('Ctrl Pts',(18.18,80.3830830991268,3.07353339195251));
#71781=CARTESIAN_POINT('Ctrl Pts',(18.18,79.9890859663486,3.07353339195251));
#71782=CARTESIAN_POINT('Ctrl Pts',(18.3,79.1727148234844,2.75375164151192));
#71783=CARTESIAN_POINT('Ctrl Pts',(18.1272,79.1727148234844,2.75375164151192));
#71784=CARTESIAN_POINT('Ctrl Pts',(18.3,79.1727148234844,2.985129570961));
#71785=CARTESIAN_POINT('Ctrl Pts',(18.1272,79.1727148234844,2.985129570961));
#71786=CARTESIAN_POINT('Ctrl Pts',(18.3,79.3386085569858,3.11718962192535));
#71787=CARTESIAN_POINT('Ctrl Pts',(18.1272,79.3386085569858,3.11718962192535));
#71788=CARTESIAN_POINT('',(18.3,79.1727148234844,2.75375164151192));
#71789=CARTESIAN_POINT('',(18.3,79.3386085569858,3.11718962192535));
#71790=CARTESIAN_POINT('Ctrl Pts',(18.3,79.1727148234844,2.75375164151192));
#71791=CARTESIAN_POINT('Ctrl Pts',(18.3,79.1727148234844,2.985129570961));
#71792=CARTESIAN_POINT('Ctrl Pts',(18.3,79.3386085569858,3.11718962192535));
#71793=CARTESIAN_POINT('',(18.18,79.1727148234844,2.75375164151192));
#71794=CARTESIAN_POINT('',(18.3,79.1727148234844,2.75375164151192));
#71795=CARTESIAN_POINT('',(18.18,79.3386085569858,3.11718962192535));
#71796=CARTESIAN_POINT('Ctrl Pts',(18.18,79.1727148234844,2.75375164151192));
#71797=CARTESIAN_POINT('Ctrl Pts',(18.18,79.1727148234844,2.985129570961));
#71798=CARTESIAN_POINT('Ctrl Pts',(18.18,79.3386085569858,3.11718962192535));
#71799=CARTESIAN_POINT('',(18.3,79.3386085569858,3.11718962192535));
#71800=CARTESIAN_POINT('Ctrl Pts',(18.3,79.2671214282513,2.46289229989052));
#71801=CARTESIAN_POINT('Ctrl Pts',(18.1272,79.2671214282513,2.46289229989052));
#71802=CARTESIAN_POINT('Ctrl Pts',(18.3,79.1727148234844,2.57803550958633));
#71803=CARTESIAN_POINT('Ctrl Pts',(18.1272,79.1727148234844,2.57803550958633));
#71804=CARTESIAN_POINT('Ctrl Pts',(18.3,79.1727148234844,2.75375164151192));
#71805=CARTESIAN_POINT('Ctrl Pts',(18.1272,79.1727148234844,2.75375164151192));
#71806=CARTESIAN_POINT('',(18.3,79.2671214282513,2.46289229989052));
#71807=CARTESIAN_POINT('Ctrl Pts',(18.3,79.2671214282513,2.46289229989052));
#71808=CARTESIAN_POINT('Ctrl Pts',(18.3,79.1727148234844,2.57803550958633));
#71809=CARTESIAN_POINT('Ctrl Pts',(18.3,79.1727148234844,2.75375164151192));
#71810=CARTESIAN_POINT('',(18.18,79.2671214282513,2.46289229989052));
#71811=CARTESIAN_POINT('',(18.3,79.2671214282513,2.46289229989052));
#71812=CARTESIAN_POINT('Ctrl Pts',(18.18,79.2671214282513,2.46289229989052));
#71813=CARTESIAN_POINT('Ctrl Pts',(18.18,79.1727148234844,2.57803550958633));
#71814=CARTESIAN_POINT('Ctrl Pts',(18.18,79.1727148234844,2.75375164151192));
#71815=CARTESIAN_POINT('Ctrl Pts',(18.3,79.5345156133175,2.28990457057953));
#71816=CARTESIAN_POINT('Ctrl Pts',(18.1272,79.5345156133175,2.28990457057953));
#71817=CARTESIAN_POINT('Ctrl Pts',(18.3,79.3615280330181,2.34774894118309));
#71818=CARTESIAN_POINT('Ctrl Pts',(18.1272,79.3615280330181,2.34774894118309));
#71819=CARTESIAN_POINT('Ctrl Pts',(18.3,79.2671214282513,2.46289229989052));
#71820=CARTESIAN_POINT('Ctrl Pts',(18.1272,79.2671214282513,2.46289229989052));
#71821=CARTESIAN_POINT('',(18.3,79.5345156133175,2.28990457057953));
#71822=CARTESIAN_POINT('Ctrl Pts',(18.3,79.5345156133175,2.28990457057953));
#71823=CARTESIAN_POINT('Ctrl Pts',(18.3,79.3615280330181,2.34774894118309));
#71824=CARTESIAN_POINT('Ctrl Pts',(18.3,79.2671214282513,2.46289229989052));
#71825=CARTESIAN_POINT('',(18.18,79.5345156133175,2.28990457057953));
#71826=CARTESIAN_POINT('',(18.3,79.5345156133175,2.28990457057953));
#71827=CARTESIAN_POINT('Ctrl Pts',(18.18,79.5345156133175,2.28990457057953));
#71828=CARTESIAN_POINT('Ctrl Pts',(18.18,79.3615280330181,2.34774894118309));
#71829=CARTESIAN_POINT('Ctrl Pts',(18.18,79.2671214282513,2.46289229989052));
#71830=CARTESIAN_POINT('Ctrl Pts',(18.3,79.9890859663486,2.23206005096436));
#71831=CARTESIAN_POINT('Ctrl Pts',(18.1272,79.9890859663486,2.23206005096436));
#71832=CARTESIAN_POINT('Ctrl Pts',(18.3,79.7075034916401,2.23206005096436));
#71833=CARTESIAN_POINT('Ctrl Pts',(18.1272,79.7075034916401,2.23206005096436));
#71834=CARTESIAN_POINT('Ctrl Pts',(18.3,79.5345156133175,2.28990457057953));
#71835=CARTESIAN_POINT('Ctrl Pts',(18.1272,79.5345156133175,2.28990457057953));
#71836=CARTESIAN_POINT('',(18.3,79.9890859663486,2.23206005096436));
#71837=CARTESIAN_POINT('Ctrl Pts',(18.3,79.9890859663486,2.23206005096436));
#71838=CARTESIAN_POINT('Ctrl Pts',(18.3,79.7075034916401,2.23206005096436));
#71839=CARTESIAN_POINT('Ctrl Pts',(18.3,79.5345156133175,2.28990457057953));
#71840=CARTESIAN_POINT('',(18.18,79.9890859663486,2.23206005096436));
#71841=CARTESIAN_POINT('',(18.3,79.9890859663486,2.23206005096436));
#71842=CARTESIAN_POINT('Ctrl Pts',(18.18,79.9890859663486,2.23206005096436));
#71843=CARTESIAN_POINT('Ctrl Pts',(18.18,79.7075034916401,2.23206005096436));
#71844=CARTESIAN_POINT('Ctrl Pts',(18.18,79.5345156133175,2.28990457057953));
#71845=CARTESIAN_POINT('Ctrl Pts',(18.3,80.3672577679157,2.26807645559311));
#71846=CARTESIAN_POINT('Ctrl Pts',(18.1272,80.3672577679157,2.26807645559311));
#71847=CARTESIAN_POINT('Ctrl Pts',(18.3,80.2270122110844,2.23206005096436));
#71848=CARTESIAN_POINT('Ctrl Pts',(18.1272,80.2270122110844,2.23206005096436));
#71849=CARTESIAN_POINT('Ctrl Pts',(18.3,79.9890859663486,2.23206005096436));
#71850=CARTESIAN_POINT('Ctrl Pts',(18.1272,79.9890859663486,2.23206005096436));
#71851=CARTESIAN_POINT('',(18.3,80.3672577679157,2.26807645559311));
#71852=CARTESIAN_POINT('Ctrl Pts',(18.3,80.3672577679157,2.26807645559311));
#71853=CARTESIAN_POINT('Ctrl Pts',(18.3,80.2270122110844,2.23206005096436));
#71854=CARTESIAN_POINT('Ctrl Pts',(18.3,79.9890859663486,2.23206005096436));
#71855=CARTESIAN_POINT('',(18.18,80.3672577679157,2.26807645559311));
#71856=CARTESIAN_POINT('',(18.3,80.3672577679157,2.26807645559311));
#71857=CARTESIAN_POINT('Ctrl Pts',(18.18,80.3672577679157,2.26807645559311));
#71858=CARTESIAN_POINT('Ctrl Pts',(18.18,80.2270122110844,2.23206005096436));
#71859=CARTESIAN_POINT('Ctrl Pts',(18.18,79.9890859663486,2.23206005096436));
#71860=CARTESIAN_POINT('Ctrl Pts',(18.3,80.605184161663,2.36739433407783));
#71861=CARTESIAN_POINT('Ctrl Pts',(18.1272,80.605184161663,2.36739433407783));
#71862=CARTESIAN_POINT('Ctrl Pts',(18.3,80.5075034737587,2.30409256219864));
#71863=CARTESIAN_POINT('Ctrl Pts',(18.1272,80.5075034737587,2.30409256219864));
#71864=CARTESIAN_POINT('Ctrl Pts',(18.3,80.3672577679157,2.26807645559311));
#71865=CARTESIAN_POINT('Ctrl Pts',(18.1272,80.3672577679157,2.26807645559311));
#71866=CARTESIAN_POINT('',(18.3,80.605184161663,2.36739433407783));
#71867=CARTESIAN_POINT('Ctrl Pts',(18.3,80.605184161663,2.36739433407783));
#71868=CARTESIAN_POINT('Ctrl Pts',(18.3,80.5075034737587,2.30409256219864));
#71869=CARTESIAN_POINT('Ctrl Pts',(18.3,80.3672577679157,2.26807645559311));
#71870=CARTESIAN_POINT('',(18.18,80.605184161663,2.36739433407783));
#71871=CARTESIAN_POINT('',(18.3,80.605184161663,2.36739433407783));
#71872=CARTESIAN_POINT('Ctrl Pts',(18.18,80.605184161663,2.36739433407783));
#71873=CARTESIAN_POINT('Ctrl Pts',(18.18,80.5075034737587,2.30409256219864));
#71874=CARTESIAN_POINT('Ctrl Pts',(18.18,80.3672577679157,2.26807645559311));
#71875=CARTESIAN_POINT('Ctrl Pts',(18.3,80.7547067344189,2.52783096432686));
#71876=CARTESIAN_POINT('Ctrl Pts',(18.1272,80.7547067344189,2.52783096432686));
#71877=CARTESIAN_POINT('Ctrl Pts',(18.3,80.702864998579,2.43069580793381));
#71878=CARTESIAN_POINT('Ctrl Pts',(18.1272,80.702864998579,2.43069580793381));
#71879=CARTESIAN_POINT('Ctrl Pts',(18.3,80.605184161663,2.36739433407783));
#71880=CARTESIAN_POINT('Ctrl Pts',(18.1272,80.605184161663,2.36739433407783));
#71881=CARTESIAN_POINT('',(18.3,80.7547067344189,2.52783096432686));
#71882=CARTESIAN_POINT('Ctrl Pts',(18.3,80.7547067344189,2.52783096432686));
#71883=CARTESIAN_POINT('Ctrl Pts',(18.3,80.702864998579,2.43069580793381));
#71884=CARTESIAN_POINT('Ctrl Pts',(18.3,80.605184161663,2.36739433407783));
#71885=CARTESIAN_POINT('',(18.18,80.7547067344189,2.52783096432686));
#71886=CARTESIAN_POINT('',(18.3,80.7547067344189,2.52783096432686));
#71887=CARTESIAN_POINT('Ctrl Pts',(18.18,80.7547067344189,2.52783096432686));
#71888=CARTESIAN_POINT('Ctrl Pts',(18.18,80.702864998579,2.43069580793381));
#71889=CARTESIAN_POINT('Ctrl Pts',(18.18,80.605184161663,2.36739433407783));
#71890=CARTESIAN_POINT('Ctrl Pts',(18.3,80.8065484702587,2.75375164151192));
#71891=CARTESIAN_POINT('Ctrl Pts',(18.1272,80.8065484702587,2.75375164151192));
#71892=CARTESIAN_POINT('Ctrl Pts',(18.3,80.8065484702587,2.6249659717083));
#71893=CARTESIAN_POINT('Ctrl Pts',(18.1272,80.8065484702587,2.6249659717083));
#71894=CARTESIAN_POINT('Ctrl Pts',(18.3,80.7547067344189,2.52783096432686));
#71895=CARTESIAN_POINT('Ctrl Pts',(18.1272,80.7547067344189,2.52783096432686));
#71896=CARTESIAN_POINT('',(18.3,80.8065484702587,2.75375164151192));
#71897=CARTESIAN_POINT('Ctrl Pts',(18.3,80.8065484702587,2.75375164151192));
#71898=CARTESIAN_POINT('Ctrl Pts',(18.3,80.8065484702587,2.6249659717083));
#71899=CARTESIAN_POINT('Ctrl Pts',(18.3,80.7547067344189,2.52783096432686));
#71900=CARTESIAN_POINT('',(18.18,80.8065484702587,2.75375164151192));
#71901=CARTESIAN_POINT('',(18.3,80.8065484702587,2.75375164151192));
#71902=CARTESIAN_POINT('Ctrl Pts',(18.18,80.8065484702587,2.75375164151192));
#71903=CARTESIAN_POINT('Ctrl Pts',(18.18,80.8065484702587,2.6249659717083));
#71904=CARTESIAN_POINT('Ctrl Pts',(18.18,80.7547067344189,2.52783096432686));
#71905=CARTESIAN_POINT('Ctrl Pts',(18.3,80.7126876950264,3.04351977109909));
#71906=CARTESIAN_POINT('Ctrl Pts',(18.1272,80.7126876950264,3.04351977109909));
#71907=CARTESIAN_POINT('Ctrl Pts',(18.3,80.8065484702587,2.92837656140327));
#71908=CARTESIAN_POINT('Ctrl Pts',(18.1272,80.8065484702587,2.92837656140327));
#71909=CARTESIAN_POINT('Ctrl Pts',(18.3,80.8065484702587,2.75375164151192));
#71910=CARTESIAN_POINT('Ctrl Pts',(18.1272,80.8065484702587,2.75375164151192));
#71911=CARTESIAN_POINT('',(18.3,80.7126876950264,3.04351977109909));
#71912=CARTESIAN_POINT('Ctrl Pts',(18.3,80.7126876950264,3.04351977109909));
#71913=CARTESIAN_POINT('Ctrl Pts',(18.3,80.8065484702587,2.92837656140327));
#71914=CARTESIAN_POINT('Ctrl Pts',(18.3,80.8065484702587,2.75375164151192));
#71915=CARTESIAN_POINT('',(18.18,80.7126876950264,3.04351977109909));
#71916=CARTESIAN_POINT('',(18.3,80.7126876950264,3.04351977109909));
#71917=CARTESIAN_POINT('Ctrl Pts',(18.18,80.7126876950264,3.04351977109909));
#71918=CARTESIAN_POINT('Ctrl Pts',(18.18,80.8065484702587,2.92837656140327));
#71919=CARTESIAN_POINT('Ctrl Pts',(18.18,80.8065484702587,2.75375164151192));
#71920=CARTESIAN_POINT('Ctrl Pts',(18.3,80.4458390414715,3.217053180933));
#71921=CARTESIAN_POINT('Ctrl Pts',(18.1272,80.4458390414715,3.217053180933));
#71922=CARTESIAN_POINT('Ctrl Pts',(18.3,80.6188267707825,3.15866298079491));
#71923=CARTESIAN_POINT('Ctrl Pts',(18.1272,80.6188267707825,3.15866298079491));
#71924=CARTESIAN_POINT('Ctrl Pts',(18.3,80.7126876950264,3.04351977109909));
#71925=CARTESIAN_POINT('Ctrl Pts',(18.1272,80.7126876950264,3.04351977109909));
#71926=CARTESIAN_POINT('',(18.3,80.4458390414715,3.217053180933));
#71927=CARTESIAN_POINT('Ctrl Pts',(18.3,80.4458390414715,3.217053180933));
#71928=CARTESIAN_POINT('Ctrl Pts',(18.3,80.6188267707825,3.15866298079491));
#71929=CARTESIAN_POINT('Ctrl Pts',(18.3,80.7126876950264,3.04351977109909));
#71930=CARTESIAN_POINT('',(18.18,80.4458390414715,3.217053180933));
#71931=CARTESIAN_POINT('',(18.3,80.4458390414715,3.217053180933));
#71932=CARTESIAN_POINT('Ctrl Pts',(18.18,80.4458390414715,3.217053180933));
#71933=CARTESIAN_POINT('Ctrl Pts',(18.18,80.6188267707825,3.15866298079491));
#71934=CARTESIAN_POINT('Ctrl Pts',(18.18,80.7126876950264,3.04351977109909));
#71935=CARTESIAN_POINT('Ctrl Pts',(18.3,79.9890859663486,3.27544338107109));
#71936=CARTESIAN_POINT('Ctrl Pts',(18.1272,79.9890859663486,3.27544338107109));
#71937=CARTESIAN_POINT('Ctrl Pts',(18.3,80.2728513121605,3.27544338107109));
#71938=CARTESIAN_POINT('Ctrl Pts',(18.1272,80.2728513121605,3.27544338107109));
#71939=CARTESIAN_POINT('Ctrl Pts',(18.3,80.4458390414715,3.217053180933));
#71940=CARTESIAN_POINT('Ctrl Pts',(18.1272,80.4458390414715,3.217053180933));
#71941=CARTESIAN_POINT('',(18.3,79.9890859663486,3.27544338107109));
#71942=CARTESIAN_POINT('Ctrl Pts',(18.3,79.9890859663486,3.27544338107109));
#71943=CARTESIAN_POINT('Ctrl Pts',(18.3,80.2728513121605,3.27544338107109));
#71944=CARTESIAN_POINT('Ctrl Pts',(18.3,80.4458390414715,3.217053180933));
#71945=CARTESIAN_POINT('',(18.18,79.9890859663486,3.27544338107109));
#71946=CARTESIAN_POINT('',(18.3,79.9890859663486,3.27544338107109));
#71947=CARTESIAN_POINT('Ctrl Pts',(18.18,79.9890859663486,3.27544338107109));
#71948=CARTESIAN_POINT('Ctrl Pts',(18.18,80.2728513121605,3.27544338107109));
#71949=CARTESIAN_POINT('Ctrl Pts',(18.18,80.4458390414715,3.217053180933));
#71950=CARTESIAN_POINT('Ctrl Pts',(18.3,79.3386085569858,3.11718962192535));
#71951=CARTESIAN_POINT('Ctrl Pts',(18.1272,79.3386085569858,3.11718962192535));
#71952=CARTESIAN_POINT('Ctrl Pts',(18.3,79.5383356750011,3.27544338107109));
#71953=CARTESIAN_POINT('Ctrl Pts',(18.1272,79.5383356750011,3.27544338107109));
#71954=CARTESIAN_POINT('Ctrl Pts',(18.3,79.9890859663486,3.27544338107109));
#71955=CARTESIAN_POINT('Ctrl Pts',(18.1272,79.9890859663486,3.27544338107109));
#71956=CARTESIAN_POINT('Ctrl Pts',(18.3,79.3386085569858,3.11718962192535));
#71957=CARTESIAN_POINT('Ctrl Pts',(18.3,79.5383356750011,3.27544338107109));
#71958=CARTESIAN_POINT('Ctrl Pts',(18.3,79.9890859663486,3.27544338107109));
#71959=CARTESIAN_POINT('Ctrl Pts',(18.18,79.3386085569858,3.11718962192535));
#71960=CARTESIAN_POINT('Ctrl Pts',(18.18,79.5383356750011,3.27544338107109));
#71961=CARTESIAN_POINT('Ctrl Pts',(18.18,79.9890859663486,3.27544338107109));
#71962=CARTESIAN_POINT('Origin',(18.18,79.9896316468716,3.29999997317791));
#71963=CARTESIAN_POINT('Origin',(18.3,80.8065484702587,3.90518411099911));
#71964=CARTESIAN_POINT('',(18.3,80.8065484702587,3.90518411099911));
#71965=CARTESIAN_POINT('',(18.3,80.8065484702587,3.77858108878136));
#71966=CARTESIAN_POINT('',(18.3,80.8065484702587,4.70259205549955));
#71967=CARTESIAN_POINT('',(18.18,80.8065484702587,3.90518411099911));
#71968=CARTESIAN_POINT('',(18.3,80.8065484702587,3.90518411099911));
#71969=CARTESIAN_POINT('',(18.18,80.8065484702587,3.77858108878136));
#71970=CARTESIAN_POINT('',(18.18,80.8065484702587,3.90518411099911));
#71971=CARTESIAN_POINT('',(18.3,80.8065484702587,3.77858108878136));
#71972=CARTESIAN_POINT('Ctrl Pts',(18.3,80.5926330626011,4.07980895638466));
#71973=CARTESIAN_POINT('Ctrl Pts',(18.1272,80.5926330626011,4.07980895638466));
#71974=CARTESIAN_POINT('Ctrl Pts',(18.3,80.702864998579,3.95648016631603));
#71975=CARTESIAN_POINT('Ctrl Pts',(18.1272,80.702864998579,3.95648016631603));
#71976=CARTESIAN_POINT('Ctrl Pts',(18.3,80.8065484702587,3.90518411099911));
#71977=CARTESIAN_POINT('Ctrl Pts',(18.1272,80.8065484702587,3.90518411099911));
#71978=CARTESIAN_POINT('',(18.3,80.5926330626011,4.07980895638466));
#71979=CARTESIAN_POINT('Ctrl Pts',(18.3,80.5926330626011,4.07980895638466));
#71980=CARTESIAN_POINT('Ctrl Pts',(18.3,80.702864998579,3.95648016631603));
#71981=CARTESIAN_POINT('Ctrl Pts',(18.3,80.8065484702587,3.90518411099911));
#71982=CARTESIAN_POINT('',(18.18,80.5926330626011,4.07980895638466));
#71983=CARTESIAN_POINT('',(18.3,80.5926330626011,4.07980895638466));
#71984=CARTESIAN_POINT('Ctrl Pts',(18.18,80.5926330626011,4.07980895638466));
#71985=CARTESIAN_POINT('Ctrl Pts',(18.18,80.702864998579,3.95648016631603));
#71986=CARTESIAN_POINT('Ctrl Pts',(18.18,80.8065484702587,3.90518411099911));
#71987=CARTESIAN_POINT('Ctrl Pts',(18.3,80.4049113631248,4.36793989539146));
#71988=CARTESIAN_POINT('Ctrl Pts',(18.1272,80.4049113631248,4.36793989539146));
#71989=CARTESIAN_POINT('Ctrl Pts',(18.3,80.4824011266231,4.20313774645328));
#71990=CARTESIAN_POINT('Ctrl Pts',(18.1272,80.4824011266231,4.20313774645328));
#71991=CARTESIAN_POINT('Ctrl Pts',(18.3,80.5926330626011,4.07980895638466));
#71992=CARTESIAN_POINT('Ctrl Pts',(18.1272,80.5926330626011,4.07980895638466));
#71993=CARTESIAN_POINT('',(18.3,80.4049113631248,4.36793989539146));
#71994=CARTESIAN_POINT('Ctrl Pts',(18.3,80.4049113631248,4.36793989539146));
#71995=CARTESIAN_POINT('Ctrl Pts',(18.3,80.4824011266231,4.20313774645328));
#71996=CARTESIAN_POINT('Ctrl Pts',(18.3,80.5926330626011,4.07980895638466));
#71997=CARTESIAN_POINT('',(18.18,80.4049113631248,4.36793989539146));
#71998=CARTESIAN_POINT('',(18.3,80.4049113631248,4.36793989539146));
#71999=CARTESIAN_POINT('Ctrl Pts',(18.18,80.4049113631248,4.36793989539146));
#72000=CARTESIAN_POINT('Ctrl Pts',(18.18,80.4824011266231,4.20313774645328));
#72001=CARTESIAN_POINT('Ctrl Pts',(18.18,80.5926330626011,4.07980895638466));
#72002=CARTESIAN_POINT('Origin',(18.3,80.2150069415569,4.36793989539146));
#72003=CARTESIAN_POINT('',(18.3,80.2150069415569,4.36793989539146));
#72004=CARTESIAN_POINT('',(18.3,75.1075034707785,4.36793989539146));
#72005=CARTESIAN_POINT('',(18.18,80.2150069415569,4.36793989539146));
#72006=CARTESIAN_POINT('',(18.3,80.2150069415569,4.36793989539146));
#72007=CARTESIAN_POINT('',(18.18,80.2150069415569,4.36793989539146));
#72008=CARTESIAN_POINT('Ctrl Pts',(18.3,80.3165075421333,4.16111863255501));
#72009=CARTESIAN_POINT('Ctrl Pts',(18.1272,80.3165075421333,4.16111863255501));
#72010=CARTESIAN_POINT('Ctrl Pts',(18.3,80.2488404750824,4.27626184225082));
#72011=CARTESIAN_POINT('Ctrl Pts',(18.1272,80.2488404750824,4.27626184225082));
#72012=CARTESIAN_POINT('Ctrl Pts',(18.3,80.2150069415569,4.36793989539146));
#72013=CARTESIAN_POINT('Ctrl Pts',(18.1272,80.2150069415569,4.36793989539146));
#72014=CARTESIAN_POINT('',(18.3,80.3165075421333,4.16111863255501));
#72015=CARTESIAN_POINT('Ctrl Pts',(18.3,80.3165075421333,4.16111863255501));
#72016=CARTESIAN_POINT('Ctrl Pts',(18.3,80.2488404750824,4.27626184225082));
#72017=CARTESIAN_POINT('Ctrl Pts',(18.3,80.2150069415569,4.36793989539146));
#72018=CARTESIAN_POINT('',(18.18,80.3165075421333,4.16111863255501));
#72019=CARTESIAN_POINT('',(18.3,80.3165075421333,4.16111863255501));
#72020=CARTESIAN_POINT('Ctrl Pts',(18.18,80.3165075421333,4.16111863255501));
#72021=CARTESIAN_POINT('Ctrl Pts',(18.18,80.2488404750824,4.27626184225082));
#72022=CARTESIAN_POINT('Ctrl Pts',(18.18,80.2150069415569,4.36793989539146));
#72023=CARTESIAN_POINT('Ctrl Pts',(18.3,80.4518418252468,3.97503404915333));
#72024=CARTESIAN_POINT('Ctrl Pts',(18.1272,80.4518418252468,3.97503404915333));
#72025=CARTESIAN_POINT('Ctrl Pts',(18.3,80.3841747581959,4.04597542285919));
#72026=CARTESIAN_POINT('Ctrl Pts',(18.1272,80.3841747581959,4.04597542285919));
#72027=CARTESIAN_POINT('Ctrl Pts',(18.3,80.3165075421333,4.16111863255501));
#72028=CARTESIAN_POINT('Ctrl Pts',(18.1272,80.3165075421333,4.16111863255501));
#72029=CARTESIAN_POINT('',(18.3,80.4518418252468,3.97503404915333));
#72030=CARTESIAN_POINT('Ctrl Pts',(18.3,80.4518418252468,3.97503404915333));
#72031=CARTESIAN_POINT('Ctrl Pts',(18.3,80.3841747581959,4.04597542285919));
#72032=CARTESIAN_POINT('Ctrl Pts',(18.3,80.3165075421333,4.16111863255501));
#72033=CARTESIAN_POINT('',(18.18,80.4518418252468,3.97503404915333));
#72034=CARTESIAN_POINT('',(18.3,80.4518418252468,3.97503404915333));
#72035=CARTESIAN_POINT('Ctrl Pts',(18.18,80.4518418252468,3.97503404915333));
#72036=CARTESIAN_POINT('Ctrl Pts',(18.18,80.3841747581959,4.04597542285919));
#72037=CARTESIAN_POINT('Ctrl Pts',(18.18,80.3165075421333,4.16111863255501));
#72038=CARTESIAN_POINT('Origin',(18.3,79.2000000417232,3.97503404915333));
#72039=CARTESIAN_POINT('',(18.3,79.2000000417232,3.97503404915333));
#72040=CARTESIAN_POINT('',(18.3,74.6000000208616,3.97503404915333));
#72041=CARTESIAN_POINT('',(18.18,79.2000000417232,3.97503404915333));
#72042=CARTESIAN_POINT('',(18.3,79.2000000417232,3.97503404915333));
#72043=CARTESIAN_POINT('',(18.18,79.2000000417232,3.97503404915333));
#72044=CARTESIAN_POINT('Origin',(18.3,79.2000000417232,3.77858108878136));
#72045=CARTESIAN_POINT('',(18.3,79.2000000417232,3.77858108878136));
#72046=CARTESIAN_POINT('',(18.3,79.2000000417232,4.63929054439068));
#72047=CARTESIAN_POINT('',(18.18,79.2000000417232,3.77858108878136));
#72048=CARTESIAN_POINT('',(18.3,79.2000000417232,3.77858108878136));
#72049=CARTESIAN_POINT('',(18.18,79.2000000417232,3.77858108878136));
#72050=CARTESIAN_POINT('Origin',(18.3,80.8065484702587,3.77858108878136));
#72051=CARTESIAN_POINT('',(18.3,75.4032742351294,3.77858108878136));
#72052=CARTESIAN_POINT('',(18.18,80.8065484702587,3.77858108878136));
#72053=CARTESIAN_POINT('Origin',(18.18,79.9896316468716,3.29999997317791));
#72054=CARTESIAN_POINT('Origin',(18.3,70.,5.5));
#72055=CARTESIAN_POINT('Ctrl Pts',(18.3,70.6439290940762,3.30218293741345));
#72056=CARTESIAN_POINT('Ctrl Pts',(18.1272,70.6439290940762,3.30218293741345));
#72057=CARTESIAN_POINT('Ctrl Pts',(18.3,70.6439290940762,3.43751707151532));
#72058=CARTESIAN_POINT('Ctrl Pts',(18.1272,70.6439290940762,3.43751707151532));
#72059=CARTESIAN_POINT('Ctrl Pts',(18.3,70.5293315649033,3.51828106716275));
#72060=CARTESIAN_POINT('Ctrl Pts',(18.1272,70.5293315649033,3.51828106716275));
#72061=CARTESIAN_POINT('',(18.3,70.6439290940762,3.30218293741345));
#72062=CARTESIAN_POINT('',(18.3,70.5293315649033,3.51828106716275));
#72063=CARTESIAN_POINT('Ctrl Pts',(18.3,70.6439290940762,3.30218293741345));
#72064=CARTESIAN_POINT('Ctrl Pts',(18.3,70.6439290940762,3.43751707151532));
#72065=CARTESIAN_POINT('Ctrl Pts',(18.3,70.5293315649033,3.51828106716275));
#72066=CARTESIAN_POINT('',(18.18,70.6439290940762,3.30218293741345));
#72067=CARTESIAN_POINT('',(18.3,70.6439290940762,3.30218293741345));
#72068=CARTESIAN_POINT('',(18.18,70.5293315649033,3.51828106716275));
#72069=CARTESIAN_POINT('Ctrl Pts',(18.18,70.6439290940762,3.30218293741345));
#72070=CARTESIAN_POINT('Ctrl Pts',(18.18,70.6439290940762,3.43751707151532));
#72071=CARTESIAN_POINT('Ctrl Pts',(18.18,70.5293315649033,3.51828106716275));
#72072=CARTESIAN_POINT('',(18.3,70.5293315649033,3.51828106716275));
#72073=CARTESIAN_POINT('Ctrl Pts',(18.3,70.5140519142151,3.07244219854474));
#72074=CARTESIAN_POINT('Ctrl Pts',(18.1272,70.5140519142151,3.07244219854474));
#72075=CARTESIAN_POINT('Ctrl Pts',(18.3,70.6439290940762,3.16466578319669));
#72076=CARTESIAN_POINT('Ctrl Pts',(18.1272,70.6439290940762,3.16466578319669));
#72077=CARTESIAN_POINT('Ctrl Pts',(18.3,70.6439290940762,3.30218293741345));
#72078=CARTESIAN_POINT('Ctrl Pts',(18.1272,70.6439290940762,3.30218293741345));
#72079=CARTESIAN_POINT('',(18.3,70.5140519142151,3.07244219854474));
#72080=CARTESIAN_POINT('Ctrl Pts',(18.3,70.5140519142151,3.07244219854474));
#72081=CARTESIAN_POINT('Ctrl Pts',(18.3,70.6439290940762,3.16466578319669));
#72082=CARTESIAN_POINT('Ctrl Pts',(18.3,70.6439290940762,3.30218293741345));
#72083=CARTESIAN_POINT('',(18.18,70.5140519142151,3.07244219854474));
#72084=CARTESIAN_POINT('',(18.3,70.5140519142151,3.07244219854474));
#72085=CARTESIAN_POINT('Ctrl Pts',(18.18,70.5140519142151,3.07244219854474));
#72086=CARTESIAN_POINT('Ctrl Pts',(18.18,70.6439290940762,3.16466578319669));
#72087=CARTESIAN_POINT('Ctrl Pts',(18.18,70.6439290940762,3.30218293741345));
#72088=CARTESIAN_POINT('Ctrl Pts',(18.3,69.9890859425068,2.98021831586957));
#72089=CARTESIAN_POINT('Ctrl Pts',(18.1272,69.9890859425068,2.98021831586957));
#72090=CARTESIAN_POINT('Ctrl Pts',(18.3,70.3841745853424,2.98021831586957));
#72091=CARTESIAN_POINT('Ctrl Pts',(18.1272,70.3841745853424,2.98021831586957));
#72092=CARTESIAN_POINT('Ctrl Pts',(18.3,70.5140519142151,3.07244219854474));
#72093=CARTESIAN_POINT('Ctrl Pts',(18.1272,70.5140519142151,3.07244219854474));
#72094=CARTESIAN_POINT('',(18.3,69.9890859425068,2.98021831586957));
#72095=CARTESIAN_POINT('Ctrl Pts',(18.3,69.9890859425068,2.98021831586957));
#72096=CARTESIAN_POINT('Ctrl Pts',(18.3,70.3841745853424,2.98021831586957));
#72097=CARTESIAN_POINT('Ctrl Pts',(18.3,70.5140519142151,3.07244219854474));
#72098=CARTESIAN_POINT('',(18.18,69.9890859425068,2.98021831586957));
#72099=CARTESIAN_POINT('',(18.3,69.9890859425068,2.98021831586957));
#72100=CARTESIAN_POINT('Ctrl Pts',(18.18,69.9890859425068,2.98021831586957));
#72101=CARTESIAN_POINT('Ctrl Pts',(18.18,70.3841745853424,2.98021831586957));
#72102=CARTESIAN_POINT('Ctrl Pts',(18.18,70.5140519142151,3.07244219854474));
#72103=CARTESIAN_POINT('Ctrl Pts',(18.3,69.4652114808559,3.07244219854474));
#72104=CARTESIAN_POINT('Ctrl Pts',(18.1272,69.4652114808559,3.07244219854474));
#72105=CARTESIAN_POINT('Ctrl Pts',(18.3,69.5961800217628,2.98021831586957));
#72106=CARTESIAN_POINT('Ctrl Pts',(18.1272,69.5961800217628,2.98021831586957));
#72107=CARTESIAN_POINT('Ctrl Pts',(18.3,69.9890859425068,2.98021831586957));
#72108=CARTESIAN_POINT('Ctrl Pts',(18.1272,69.9890859425068,2.98021831586957));
#72109=CARTESIAN_POINT('',(18.3,69.4652114808559,3.07244219854474));
#72110=CARTESIAN_POINT('Ctrl Pts',(18.3,69.4652114808559,3.07244219854474));
#72111=CARTESIAN_POINT('Ctrl Pts',(18.3,69.5961800217628,2.98021831586957));
#72112=CARTESIAN_POINT('Ctrl Pts',(18.3,69.9890859425068,2.98021831586957));
#72113=CARTESIAN_POINT('',(18.18,69.4652114808559,3.07244219854474));
#72114=CARTESIAN_POINT('',(18.3,69.4652114808559,3.07244219854474));
#72115=CARTESIAN_POINT('Ctrl Pts',(18.18,69.4652114808559,3.07244219854474));
#72116=CARTESIAN_POINT('Ctrl Pts',(18.18,69.5961800217628,2.98021831586957));
#72117=CARTESIAN_POINT('Ctrl Pts',(18.18,69.9890859425068,2.98021831586957));
#72118=CARTESIAN_POINT('Ctrl Pts',(18.3,69.3342427909374,3.30000006631017));
#72119=CARTESIAN_POINT('Ctrl Pts',(18.1272,69.3342427909374,3.30000006631017));
#72120=CARTESIAN_POINT('Ctrl Pts',(18.3,69.3342427909374,3.16466578319669));
#72121=CARTESIAN_POINT('Ctrl Pts',(18.1272,69.3342427909374,3.16466578319669));
#72122=CARTESIAN_POINT('Ctrl Pts',(18.3,69.4652114808559,3.07244219854474));
#72123=CARTESIAN_POINT('Ctrl Pts',(18.1272,69.4652114808559,3.07244219854474));
#72124=CARTESIAN_POINT('',(18.3,69.3342427909374,3.30000006631017));
#72125=CARTESIAN_POINT('Ctrl Pts',(18.3,69.3342427909374,3.30000006631017));
#72126=CARTESIAN_POINT('Ctrl Pts',(18.3,69.3342427909374,3.16466578319669));
#72127=CARTESIAN_POINT('Ctrl Pts',(18.3,69.4652114808559,3.07244219854474));
#72128=CARTESIAN_POINT('',(18.18,69.3342427909374,3.30000006631017));
#72129=CARTESIAN_POINT('',(18.3,69.3342427909374,3.30000006631017));
#72130=CARTESIAN_POINT('Ctrl Pts',(18.18,69.3342427909374,3.30000006631017));
#72131=CARTESIAN_POINT('Ctrl Pts',(18.18,69.3342427909374,3.16466578319669));
#72132=CARTESIAN_POINT('Ctrl Pts',(18.18,69.4652114808559,3.07244219854474));
#72133=CARTESIAN_POINT('Ctrl Pts',(18.3,69.464665800333,3.5275580085814));
#72134=CARTESIAN_POINT('Ctrl Pts',(18.1272,69.464665800333,3.5275580085814));
#72135=CARTESIAN_POINT('Ctrl Pts',(18.3,69.3342427909374,3.43533434942365));
#72136=CARTESIAN_POINT('Ctrl Pts',(18.1272,69.3342427909374,3.43533434942365));
#72137=CARTESIAN_POINT('Ctrl Pts',(18.3,69.3342427909374,3.30000006631017));
#72138=CARTESIAN_POINT('Ctrl Pts',(18.1272,69.3342427909374,3.30000006631017));
#72139=CARTESIAN_POINT('',(18.3,69.464665800333,3.5275580085814));
#72140=CARTESIAN_POINT('Ctrl Pts',(18.3,69.464665800333,3.5275580085814));
#72141=CARTESIAN_POINT('Ctrl Pts',(18.3,69.3342427909374,3.43533434942365));
#72142=CARTESIAN_POINT('Ctrl Pts',(18.3,69.3342427909374,3.30000006631017));
#72143=CARTESIAN_POINT('',(18.18,69.464665800333,3.5275580085814));
#72144=CARTESIAN_POINT('',(18.3,69.464665800333,3.5275580085814));
#72145=CARTESIAN_POINT('Ctrl Pts',(18.18,69.464665800333,3.5275580085814));
#72146=CARTESIAN_POINT('Ctrl Pts',(18.18,69.3342427909374,3.43533434942365));
#72147=CARTESIAN_POINT('Ctrl Pts',(18.18,69.3342427909374,3.30000006631017));
#72148=CARTESIAN_POINT('Ctrl Pts',(18.3,69.9890859425068,3.61978174224496));
#72149=CARTESIAN_POINT('Ctrl Pts',(18.1272,69.9890859425068,3.61978174224496));
#72150=CARTESIAN_POINT('Ctrl Pts',(18.3,69.595088660717,3.61978174224496));
#72151=CARTESIAN_POINT('Ctrl Pts',(18.1272,69.595088660717,3.61978174224496));
#72152=CARTESIAN_POINT('Ctrl Pts',(18.3,69.464665800333,3.5275580085814));
#72153=CARTESIAN_POINT('Ctrl Pts',(18.1272,69.464665800333,3.5275580085814));
#72154=CARTESIAN_POINT('',(18.3,69.9890859425068,3.61978174224496));
#72155=CARTESIAN_POINT('Ctrl Pts',(18.3,69.9890859425068,3.61978174224496));
#72156=CARTESIAN_POINT('Ctrl Pts',(18.3,69.595088660717,3.61978174224496));
#72157=CARTESIAN_POINT('Ctrl Pts',(18.3,69.464665800333,3.5275580085814));
#72158=CARTESIAN_POINT('',(18.18,69.9890859425068,3.61978174224496));
#72159=CARTESIAN_POINT('',(18.3,69.9890859425068,3.61978174224496));
#72160=CARTESIAN_POINT('Ctrl Pts',(18.18,69.9890859425068,3.61978174224496));
#72161=CARTESIAN_POINT('Ctrl Pts',(18.18,69.595088660717,3.61978174224496));
#72162=CARTESIAN_POINT('Ctrl Pts',(18.18,69.464665800333,3.5275580085814));
#72163=CARTESIAN_POINT('Ctrl Pts',(18.3,70.5293315649033,3.51828106716275));
#72164=CARTESIAN_POINT('Ctrl Pts',(18.1272,70.5293315649033,3.51828106716275));
#72165=CARTESIAN_POINT('Ctrl Pts',(18.3,70.383083075285,3.61978174224496));
#72166=CARTESIAN_POINT('Ctrl Pts',(18.1272,70.383083075285,3.61978174224496));
#72167=CARTESIAN_POINT('Ctrl Pts',(18.3,69.9890859425068,3.61978174224496));
#72168=CARTESIAN_POINT('Ctrl Pts',(18.1272,69.9890859425068,3.61978174224496));
#72169=CARTESIAN_POINT('Ctrl Pts',(18.3,70.5293315649033,3.51828106716275));
#72170=CARTESIAN_POINT('Ctrl Pts',(18.3,70.383083075285,3.61978174224496));
#72171=CARTESIAN_POINT('Ctrl Pts',(18.3,69.9890859425068,3.61978174224496));
#72172=CARTESIAN_POINT('Ctrl Pts',(18.18,70.5293315649033,3.51828106716275));
#72173=CARTESIAN_POINT('Ctrl Pts',(18.18,70.383083075285,3.61978174224496));
#72174=CARTESIAN_POINT('Ctrl Pts',(18.18,69.9890859425068,3.61978174224496));
#72175=CARTESIAN_POINT('Ctrl Pts',(18.3,69.1727147996426,3.30000006631017));
#72176=CARTESIAN_POINT('Ctrl Pts',(18.1272,69.1727147996426,3.30000006631017));
#72177=CARTESIAN_POINT('Ctrl Pts',(18.3,69.1727147996426,3.53137792125344));
#72178=CARTESIAN_POINT('Ctrl Pts',(18.1272,69.1727147996426,3.53137792125344));
#72179=CARTESIAN_POINT('Ctrl Pts',(18.3,69.338608533144,3.6634379722178));
#72180=CARTESIAN_POINT('Ctrl Pts',(18.1272,69.338608533144,3.6634379722178));
#72181=CARTESIAN_POINT('',(18.3,69.1727147996426,3.30000006631017));
#72182=CARTESIAN_POINT('',(18.3,69.338608533144,3.6634379722178));
#72183=CARTESIAN_POINT('Ctrl Pts',(18.3,69.1727147996426,3.30000006631017));
#72184=CARTESIAN_POINT('Ctrl Pts',(18.3,69.1727147996426,3.53137792125344));
#72185=CARTESIAN_POINT('Ctrl Pts',(18.3,69.338608533144,3.6634379722178));
#72186=CARTESIAN_POINT('',(18.18,69.1727147996426,3.30000006631017));
#72187=CARTESIAN_POINT('',(18.3,69.1727147996426,3.30000006631017));
#72188=CARTESIAN_POINT('',(18.18,69.338608533144,3.6634379722178));
#72189=CARTESIAN_POINT('Ctrl Pts',(18.18,69.1727147996426,3.30000006631017));
#72190=CARTESIAN_POINT('Ctrl Pts',(18.18,69.1727147996426,3.53137792125344));
#72191=CARTESIAN_POINT('Ctrl Pts',(18.18,69.338608533144,3.6634379722178));
#72192=CARTESIAN_POINT('',(18.3,69.338608533144,3.6634379722178));
#72193=CARTESIAN_POINT('Ctrl Pts',(18.3,69.2671214044094,3.00914057567716));
#72194=CARTESIAN_POINT('Ctrl Pts',(18.1272,69.2671214044094,3.00914057567716));
#72195=CARTESIAN_POINT('Ctrl Pts',(18.3,69.1727147996426,3.12428393438458));
#72196=CARTESIAN_POINT('Ctrl Pts',(18.1272,69.1727147996426,3.12428393438458));
#72197=CARTESIAN_POINT('Ctrl Pts',(18.3,69.1727147996426,3.30000006631017));
#72198=CARTESIAN_POINT('Ctrl Pts',(18.1272,69.1727147996426,3.30000006631017));
#72199=CARTESIAN_POINT('',(18.3,69.2671214044094,3.00914057567716));
#72200=CARTESIAN_POINT('Ctrl Pts',(18.3,69.2671214044094,3.00914057567716));
#72201=CARTESIAN_POINT('Ctrl Pts',(18.3,69.1727147996426,3.12428393438458));
#72202=CARTESIAN_POINT('Ctrl Pts',(18.3,69.1727147996426,3.30000006631017));
#72203=CARTESIAN_POINT('',(18.18,69.2671214044094,3.00914057567716));
#72204=CARTESIAN_POINT('',(18.3,69.2671214044094,3.00914057567716));
#72205=CARTESIAN_POINT('Ctrl Pts',(18.18,69.2671214044094,3.00914057567716));
#72206=CARTESIAN_POINT('Ctrl Pts',(18.18,69.1727147996426,3.12428393438458));
#72207=CARTESIAN_POINT('Ctrl Pts',(18.18,69.1727147996426,3.30000006631017));
#72208=CARTESIAN_POINT('Ctrl Pts',(18.3,69.5345155894756,2.83615299537778));
#72209=CARTESIAN_POINT('Ctrl Pts',(18.1272,69.5345155894756,2.83615299537778));
#72210=CARTESIAN_POINT('Ctrl Pts',(18.3,69.3615280091763,2.89399736598134));
#72211=CARTESIAN_POINT('Ctrl Pts',(18.1272,69.3615280091763,2.89399736598134));
#72212=CARTESIAN_POINT('Ctrl Pts',(18.3,69.2671214044094,3.00914057567716));
#72213=CARTESIAN_POINT('Ctrl Pts',(18.1272,69.2671214044094,3.00914057567716));
#72214=CARTESIAN_POINT('',(18.3,69.5345155894756,2.83615299537778));
#72215=CARTESIAN_POINT('Ctrl Pts',(18.3,69.5345155894756,2.83615299537778));
#72216=CARTESIAN_POINT('Ctrl Pts',(18.3,69.3615280091763,2.89399736598134));
#72217=CARTESIAN_POINT('Ctrl Pts',(18.3,69.2671214044094,3.00914057567716));
#72218=CARTESIAN_POINT('',(18.18,69.5345155894756,2.83615299537778));
#72219=CARTESIAN_POINT('',(18.3,69.5345155894756,2.83615299537778));
#72220=CARTESIAN_POINT('Ctrl Pts',(18.18,69.5345155894756,2.83615299537778));
#72221=CARTESIAN_POINT('Ctrl Pts',(18.18,69.3615280091763,2.89399736598134));
#72222=CARTESIAN_POINT('Ctrl Pts',(18.18,69.2671214044094,3.00914057567716));
#72223=CARTESIAN_POINT('Ctrl Pts',(18.3,69.9890859425068,2.77830847576261));
#72224=CARTESIAN_POINT('Ctrl Pts',(18.1272,69.9890859425068,2.77830847576261));
#72225=CARTESIAN_POINT('Ctrl Pts',(18.3,69.7075034677982,2.77830847576261));
#72226=CARTESIAN_POINT('Ctrl Pts',(18.1272,69.7075034677982,2.77830847576261));
#72227=CARTESIAN_POINT('Ctrl Pts',(18.3,69.5345155894756,2.83615299537778));
#72228=CARTESIAN_POINT('Ctrl Pts',(18.1272,69.5345155894756,2.83615299537778));
#72229=CARTESIAN_POINT('',(18.3,69.9890859425068,2.77830847576261));
#72230=CARTESIAN_POINT('Ctrl Pts',(18.3,69.9890859425068,2.77830847576261));
#72231=CARTESIAN_POINT('Ctrl Pts',(18.3,69.7075034677982,2.77830847576261));
#72232=CARTESIAN_POINT('Ctrl Pts',(18.3,69.5345155894756,2.83615299537778));
#72233=CARTESIAN_POINT('',(18.18,69.9890859425068,2.77830847576261));
#72234=CARTESIAN_POINT('',(18.3,69.9890859425068,2.77830847576261));
#72235=CARTESIAN_POINT('Ctrl Pts',(18.18,69.9890859425068,2.77830847576261));
#72236=CARTESIAN_POINT('Ctrl Pts',(18.18,69.7075034677982,2.77830847576261));
#72237=CARTESIAN_POINT('Ctrl Pts',(18.18,69.5345155894756,2.83615299537778));
#72238=CARTESIAN_POINT('Ctrl Pts',(18.3,70.3672577440739,2.81432488039136));
#72239=CARTESIAN_POINT('Ctrl Pts',(18.1272,70.3672577440739,2.81432488039136));
#72240=CARTESIAN_POINT('Ctrl Pts',(18.3,70.2270121872425,2.77830847576261));
#72241=CARTESIAN_POINT('Ctrl Pts',(18.1272,70.2270121872425,2.77830847576261));
#72242=CARTESIAN_POINT('Ctrl Pts',(18.3,69.9890859425068,2.77830847576261));
#72243=CARTESIAN_POINT('Ctrl Pts',(18.1272,69.9890859425068,2.77830847576261));
#72244=CARTESIAN_POINT('',(18.3,70.3672577440739,2.81432488039136));
#72245=CARTESIAN_POINT('Ctrl Pts',(18.3,70.3672577440739,2.81432488039136));
#72246=CARTESIAN_POINT('Ctrl Pts',(18.3,70.2270121872425,2.77830847576261));
#72247=CARTESIAN_POINT('Ctrl Pts',(18.3,69.9890859425068,2.77830847576261));
#72248=CARTESIAN_POINT('',(18.18,70.3672577440739,2.81432488039136));
#72249=CARTESIAN_POINT('',(18.3,70.3672577440739,2.81432488039136));
#72250=CARTESIAN_POINT('Ctrl Pts',(18.18,70.3672577440739,2.81432488039136));
#72251=CARTESIAN_POINT('Ctrl Pts',(18.18,70.2270121872425,2.77830847576261));
#72252=CARTESIAN_POINT('Ctrl Pts',(18.18,69.9890859425068,2.77830847576261));
#72253=CARTESIAN_POINT('Ctrl Pts',(18.3,70.6051841378212,2.91364260986447));
#72254=CARTESIAN_POINT('Ctrl Pts',(18.1272,70.6051841378212,2.91364260986447));
#72255=CARTESIAN_POINT('Ctrl Pts',(18.3,70.5075034499168,2.8503411360085));
#72256=CARTESIAN_POINT('Ctrl Pts',(18.1272,70.5075034499168,2.8503411360085));
#72257=CARTESIAN_POINT('Ctrl Pts',(18.3,70.3672577440739,2.81432488039136));
#72258=CARTESIAN_POINT('Ctrl Pts',(18.1272,70.3672577440739,2.81432488039136));
#72259=CARTESIAN_POINT('',(18.3,70.6051841378212,2.91364260986447));
#72260=CARTESIAN_POINT('Ctrl Pts',(18.3,70.6051841378212,2.91364260986447));
#72261=CARTESIAN_POINT('Ctrl Pts',(18.3,70.5075034499168,2.8503411360085));
#72262=CARTESIAN_POINT('Ctrl Pts',(18.3,70.3672577440739,2.81432488039136));
#72263=CARTESIAN_POINT('',(18.18,70.6051841378212,2.91364260986447));
#72264=CARTESIAN_POINT('',(18.3,70.6051841378212,2.91364260986447));
#72265=CARTESIAN_POINT('Ctrl Pts',(18.18,70.6051841378212,2.91364260986447));
#72266=CARTESIAN_POINT('Ctrl Pts',(18.18,70.5075034499168,2.8503411360085));
#72267=CARTESIAN_POINT('Ctrl Pts',(18.18,70.3672577440739,2.81432488039136));
#72268=CARTESIAN_POINT('Ctrl Pts',(18.3,70.754706710577,3.0740792401135));
#72269=CARTESIAN_POINT('Ctrl Pts',(18.1272,70.754706710577,3.0740792401135));
#72270=CARTESIAN_POINT('Ctrl Pts',(18.3,70.7028649747372,2.97694423273206));
#72271=CARTESIAN_POINT('Ctrl Pts',(18.1272,70.7028649747372,2.97694423273206));
#72272=CARTESIAN_POINT('Ctrl Pts',(18.3,70.6051841378212,2.91364260986447));
#72273=CARTESIAN_POINT('Ctrl Pts',(18.1272,70.6051841378212,2.91364260986447));
#72274=CARTESIAN_POINT('',(18.3,70.754706710577,3.0740792401135));
#72275=CARTESIAN_POINT('Ctrl Pts',(18.3,70.754706710577,3.0740792401135));
#72276=CARTESIAN_POINT('Ctrl Pts',(18.3,70.7028649747372,2.97694423273206));
#72277=CARTESIAN_POINT('Ctrl Pts',(18.3,70.6051841378212,2.91364260986447));
#72278=CARTESIAN_POINT('',(18.18,70.754706710577,3.0740792401135));
#72279=CARTESIAN_POINT('',(18.3,70.754706710577,3.0740792401135));
#72280=CARTESIAN_POINT('Ctrl Pts',(18.18,70.754706710577,3.0740792401135));
#72281=CARTESIAN_POINT('Ctrl Pts',(18.18,70.7028649747372,2.97694423273206));
#72282=CARTESIAN_POINT('Ctrl Pts',(18.18,70.6051841378212,2.91364260986447));
#72283=CARTESIAN_POINT('Ctrl Pts',(18.3,70.8065484464169,3.30000006631017));
#72284=CARTESIAN_POINT('Ctrl Pts',(18.1272,70.8065484464169,3.30000006631017));
#72285=CARTESIAN_POINT('Ctrl Pts',(18.3,70.8065484464169,3.17121424749494));
#72286=CARTESIAN_POINT('Ctrl Pts',(18.1272,70.8065484464169,3.17121424749494));
#72287=CARTESIAN_POINT('Ctrl Pts',(18.3,70.754706710577,3.0740792401135));
#72288=CARTESIAN_POINT('Ctrl Pts',(18.1272,70.754706710577,3.0740792401135));
#72289=CARTESIAN_POINT('',(18.3,70.8065484464169,3.30000006631017));
#72290=CARTESIAN_POINT('Ctrl Pts',(18.3,70.8065484464169,3.30000006631017));
#72291=CARTESIAN_POINT('Ctrl Pts',(18.3,70.8065484464169,3.17121424749494));
#72292=CARTESIAN_POINT('Ctrl Pts',(18.3,70.754706710577,3.0740792401135));
#72293=CARTESIAN_POINT('',(18.18,70.8065484464169,3.30000006631017));
#72294=CARTESIAN_POINT('',(18.3,70.8065484464169,3.30000006631017));
#72295=CARTESIAN_POINT('Ctrl Pts',(18.18,70.8065484464169,3.30000006631017));
#72296=CARTESIAN_POINT('Ctrl Pts',(18.18,70.8065484464169,3.17121424749494));
#72297=CARTESIAN_POINT('Ctrl Pts',(18.18,70.754706710577,3.0740792401135));
#72298=CARTESIAN_POINT('Ctrl Pts',(18.3,70.7126876711845,3.58976812139153));
#72299=CARTESIAN_POINT('Ctrl Pts',(18.1272,70.7126876711845,3.58976812139153));
#72300=CARTESIAN_POINT('Ctrl Pts',(18.3,70.8065484464169,3.47462491169572));
#72301=CARTESIAN_POINT('Ctrl Pts',(18.1272,70.8065484464169,3.47462491169572));
#72302=CARTESIAN_POINT('Ctrl Pts',(18.3,70.8065484464169,3.30000006631017));
#72303=CARTESIAN_POINT('Ctrl Pts',(18.1272,70.8065484464169,3.30000006631017));
#72304=CARTESIAN_POINT('',(18.3,70.7126876711845,3.58976812139153));
#72305=CARTESIAN_POINT('Ctrl Pts',(18.3,70.7126876711845,3.58976812139153));
#72306=CARTESIAN_POINT('Ctrl Pts',(18.3,70.8065484464169,3.47462491169572));
#72307=CARTESIAN_POINT('Ctrl Pts',(18.3,70.8065484464169,3.30000006631017));
#72308=CARTESIAN_POINT('',(18.18,70.7126876711845,3.58976812139153));
#72309=CARTESIAN_POINT('',(18.3,70.7126876711845,3.58976812139153));
#72310=CARTESIAN_POINT('Ctrl Pts',(18.18,70.7126876711845,3.58976812139153));
#72311=CARTESIAN_POINT('Ctrl Pts',(18.18,70.8065484464169,3.47462491169572));
#72312=CARTESIAN_POINT('Ctrl Pts',(18.18,70.8065484464169,3.30000006631017));
#72313=CARTESIAN_POINT('Ctrl Pts',(18.3,70.4458389431238,3.76330153122544));
#72314=CARTESIAN_POINT('Ctrl Pts',(18.1272,70.4458389431238,3.76330153122544));
#72315=CARTESIAN_POINT('Ctrl Pts',(18.3,70.6188267469406,3.70491140559316));
#72316=CARTESIAN_POINT('Ctrl Pts',(18.1272,70.6188267469406,3.70491140559316));
#72317=CARTESIAN_POINT('Ctrl Pts',(18.3,70.7126876711845,3.58976812139153));
#72318=CARTESIAN_POINT('Ctrl Pts',(18.1272,70.7126876711845,3.58976812139153));
#72319=CARTESIAN_POINT('',(18.3,70.4458389431238,3.76330153122544));
#72320=CARTESIAN_POINT('Ctrl Pts',(18.3,70.4458389431238,3.76330153122544));
#72321=CARTESIAN_POINT('Ctrl Pts',(18.3,70.6188267469406,3.70491140559316));
#72322=CARTESIAN_POINT('Ctrl Pts',(18.3,70.7126876711845,3.58976812139153));
#72323=CARTESIAN_POINT('',(18.18,70.4458389431238,3.76330153122544));
#72324=CARTESIAN_POINT('',(18.3,70.4458389431238,3.76330153122544));
#72325=CARTESIAN_POINT('Ctrl Pts',(18.18,70.4458389431238,3.76330153122544));
#72326=CARTESIAN_POINT('Ctrl Pts',(18.18,70.6188267469406,3.70491140559316));
#72327=CARTESIAN_POINT('Ctrl Pts',(18.18,70.7126876711845,3.58976812139153));
#72328=CARTESIAN_POINT('Ctrl Pts',(18.3,69.9890859425068,3.82169173136353));
#72329=CARTESIAN_POINT('Ctrl Pts',(18.1272,69.9890859425068,3.82169173136353));
#72330=CARTESIAN_POINT('Ctrl Pts',(18.3,70.2728512883186,3.82169173136353));
#72331=CARTESIAN_POINT('Ctrl Pts',(18.1272,70.2728512883186,3.82169173136353));
#72332=CARTESIAN_POINT('Ctrl Pts',(18.3,70.4458389431238,3.76330153122544));
#72333=CARTESIAN_POINT('Ctrl Pts',(18.1272,70.4458389431238,3.76330153122544));
#72334=CARTESIAN_POINT('',(18.3,69.9890859425068,3.82169173136353));
#72335=CARTESIAN_POINT('Ctrl Pts',(18.3,69.9890859425068,3.82169173136353));
#72336=CARTESIAN_POINT('Ctrl Pts',(18.3,70.2728512883186,3.82169173136353));
#72337=CARTESIAN_POINT('Ctrl Pts',(18.3,70.4458389431238,3.76330153122544));
#72338=CARTESIAN_POINT('',(18.18,69.9890859425068,3.82169173136353));
#72339=CARTESIAN_POINT('',(18.3,69.9890859425068,3.82169173136353));
#72340=CARTESIAN_POINT('Ctrl Pts',(18.18,69.9890859425068,3.82169173136353));
#72341=CARTESIAN_POINT('Ctrl Pts',(18.18,70.2728512883186,3.82169173136353));
#72342=CARTESIAN_POINT('Ctrl Pts',(18.18,70.4458389431238,3.76330153122544));
#72343=CARTESIAN_POINT('Ctrl Pts',(18.3,69.338608533144,3.6634379722178));
#72344=CARTESIAN_POINT('Ctrl Pts',(18.1272,69.338608533144,3.6634379722178));
#72345=CARTESIAN_POINT('Ctrl Pts',(18.3,69.5383356511593,3.82169173136353));
#72346=CARTESIAN_POINT('Ctrl Pts',(18.1272,69.5383356511593,3.82169173136353));
#72347=CARTESIAN_POINT('Ctrl Pts',(18.3,69.9890859425068,3.82169173136353));
#72348=CARTESIAN_POINT('Ctrl Pts',(18.1272,69.9890859425068,3.82169173136353));
#72349=CARTESIAN_POINT('Ctrl Pts',(18.3,69.338608533144,3.6634379722178));
#72350=CARTESIAN_POINT('Ctrl Pts',(18.3,69.5383356511593,3.82169173136353));
#72351=CARTESIAN_POINT('Ctrl Pts',(18.3,69.9890859425068,3.82169173136353));
#72352=CARTESIAN_POINT('Ctrl Pts',(18.18,69.338608533144,3.6634379722178));
#72353=CARTESIAN_POINT('Ctrl Pts',(18.18,69.5383356511593,3.82169173136353));
#72354=CARTESIAN_POINT('Ctrl Pts',(18.18,69.9890859425068,3.82169173136353));
#72355=CARTESIAN_POINT('Origin',(18.18,69.9896316230297,3.30000010356307));
#72356=CARTESIAN_POINT('Origin',(18.3,70.,5.5));
#72357=CARTESIAN_POINT('Ctrl Pts',(18.3,60.643929117918,2.7559345126152));
#72358=CARTESIAN_POINT('Ctrl Pts',(18.1272,60.643929117918,2.7559345126152));
#72359=CARTESIAN_POINT('Ctrl Pts',(18.3,60.643929117918,2.89126879572868));
#72360=CARTESIAN_POINT('Ctrl Pts',(18.1272,60.643929117918,2.89126879572868));
#72361=CARTESIAN_POINT('Ctrl Pts',(18.3,60.5293315887451,2.97203279137611));
#72362=CARTESIAN_POINT('Ctrl Pts',(18.1272,60.5293315887451,2.97203279137611));
#72363=CARTESIAN_POINT('',(18.3,60.643929117918,2.7559345126152));
#72364=CARTESIAN_POINT('',(18.3,60.5293315887451,2.97203279137611));
#72365=CARTESIAN_POINT('Ctrl Pts',(18.3,60.643929117918,2.7559345126152));
#72366=CARTESIAN_POINT('Ctrl Pts',(18.3,60.643929117918,2.89126879572868));
#72367=CARTESIAN_POINT('Ctrl Pts',(18.3,60.5293315887451,2.97203279137611));
#72368=CARTESIAN_POINT('',(18.18,60.643929117918,2.7559345126152));
#72369=CARTESIAN_POINT('',(18.3,60.643929117918,2.7559345126152));
#72370=CARTESIAN_POINT('',(18.18,60.5293315887451,2.97203279137611));
#72371=CARTESIAN_POINT('Ctrl Pts',(18.18,60.643929117918,2.7559345126152));
#72372=CARTESIAN_POINT('Ctrl Pts',(18.18,60.643929117918,2.89126879572868));
#72373=CARTESIAN_POINT('Ctrl Pts',(18.18,60.5293315887451,2.97203279137611));
#72374=CARTESIAN_POINT('',(18.3,60.5293315887451,2.97203279137611));
#72375=CARTESIAN_POINT('Ctrl Pts',(18.3,60.5140519380569,2.52619377374649));
#72376=CARTESIAN_POINT('Ctrl Pts',(18.1272,60.5140519380569,2.52619377374649));
#72377=CARTESIAN_POINT('Ctrl Pts',(18.3,60.643929117918,2.61841750741005));
#72378=CARTESIAN_POINT('Ctrl Pts',(18.1272,60.643929117918,2.61841750741005));
#72379=CARTESIAN_POINT('Ctrl Pts',(18.3,60.643929117918,2.7559345126152));
#72380=CARTESIAN_POINT('Ctrl Pts',(18.1272,60.643929117918,2.7559345126152));
#72381=CARTESIAN_POINT('',(18.3,60.5140519380569,2.52619377374649));
#72382=CARTESIAN_POINT('Ctrl Pts',(18.3,60.5140519380569,2.52619377374649));
#72383=CARTESIAN_POINT('Ctrl Pts',(18.3,60.643929117918,2.61841750741005));
#72384=CARTESIAN_POINT('Ctrl Pts',(18.3,60.643929117918,2.7559345126152));
#72385=CARTESIAN_POINT('',(18.18,60.5140519380569,2.52619377374649));
#72386=CARTESIAN_POINT('',(18.3,60.5140519380569,2.52619377374649));
#72387=CARTESIAN_POINT('Ctrl Pts',(18.18,60.5140519380569,2.52619377374649));
#72388=CARTESIAN_POINT('Ctrl Pts',(18.18,60.643929117918,2.61841750741005));
#72389=CARTESIAN_POINT('Ctrl Pts',(18.18,60.643929117918,2.7559345126152));
#72390=CARTESIAN_POINT('Ctrl Pts',(18.3,59.9890859663486,2.43397004008293));
#72391=CARTESIAN_POINT('Ctrl Pts',(18.1272,59.9890859663486,2.43397004008293));
#72392=CARTESIAN_POINT('Ctrl Pts',(18.3,60.3841746091843,2.43397004008293));
#72393=CARTESIAN_POINT('Ctrl Pts',(18.1272,60.3841746091843,2.43397004008293));
#72394=CARTESIAN_POINT('Ctrl Pts',(18.3,60.5140519380569,2.52619377374649));
#72395=CARTESIAN_POINT('Ctrl Pts',(18.1272,60.5140519380569,2.52619377374649));
#72396=CARTESIAN_POINT('',(18.3,59.9890859663486,2.43397004008293));
#72397=CARTESIAN_POINT('Ctrl Pts',(18.3,59.9890859663486,2.43397004008293));
#72398=CARTESIAN_POINT('Ctrl Pts',(18.3,60.3841746091843,2.43397004008293));
#72399=CARTESIAN_POINT('Ctrl Pts',(18.3,60.5140519380569,2.52619377374649));
#72400=CARTESIAN_POINT('',(18.18,59.9890859663486,2.43397004008293));
#72401=CARTESIAN_POINT('',(18.3,59.9890859663486,2.43397004008293));
#72402=CARTESIAN_POINT('Ctrl Pts',(18.18,59.9890859663486,2.43397004008293));
#72403=CARTESIAN_POINT('Ctrl Pts',(18.18,60.3841746091843,2.43397004008293));
#72404=CARTESIAN_POINT('Ctrl Pts',(18.18,60.5140519380569,2.52619377374649));
#72405=CARTESIAN_POINT('Ctrl Pts',(18.3,59.4652115046978,2.52619377374649));
#72406=CARTESIAN_POINT('Ctrl Pts',(18.1272,59.4652115046978,2.52619377374649));
#72407=CARTESIAN_POINT('Ctrl Pts',(18.3,59.5961801946163,2.43397004008293));
#72408=CARTESIAN_POINT('Ctrl Pts',(18.1272,59.5961801946163,2.43397004008293));
#72409=CARTESIAN_POINT('Ctrl Pts',(18.3,59.9890859663486,2.43397004008293));
#72410=CARTESIAN_POINT('Ctrl Pts',(18.1272,59.9890859663486,2.43397004008293));
#72411=CARTESIAN_POINT('',(18.3,59.4652115046978,2.52619377374649));
#72412=CARTESIAN_POINT('Ctrl Pts',(18.3,59.4652115046978,2.52619377374649));
#72413=CARTESIAN_POINT('Ctrl Pts',(18.3,59.5961801946163,2.43397004008293));
#72414=CARTESIAN_POINT('Ctrl Pts',(18.3,59.9890859663486,2.43397004008293));
#72415=CARTESIAN_POINT('',(18.18,59.4652115046978,2.52619377374649));
#72416=CARTESIAN_POINT('',(18.3,59.4652115046978,2.52619377374649));
#72417=CARTESIAN_POINT('Ctrl Pts',(18.18,59.4652115046978,2.52619377374649));
#72418=CARTESIAN_POINT('Ctrl Pts',(18.18,59.5961801946163,2.43397004008293));
#72419=CARTESIAN_POINT('Ctrl Pts',(18.18,59.9890859663486,2.43397004008293));
#72420=CARTESIAN_POINT('Ctrl Pts',(18.3,59.3342428147793,2.75375164151192));
#72421=CARTESIAN_POINT('Ctrl Pts',(18.1272,59.3342428147793,2.75375164151192));
#72422=CARTESIAN_POINT('Ctrl Pts',(18.3,59.3342428147793,2.61841750741005));
#72423=CARTESIAN_POINT('Ctrl Pts',(18.1272,59.3342428147793,2.61841750741005));
#72424=CARTESIAN_POINT('Ctrl Pts',(18.3,59.4652115046978,2.52619377374649));
#72425=CARTESIAN_POINT('Ctrl Pts',(18.1272,59.4652115046978,2.52619377374649));
#72426=CARTESIAN_POINT('',(18.3,59.3342428147793,2.75375164151192));
#72427=CARTESIAN_POINT('Ctrl Pts',(18.3,59.3342428147793,2.75375164151192));
#72428=CARTESIAN_POINT('Ctrl Pts',(18.3,59.3342428147793,2.61841750741005));
#72429=CARTESIAN_POINT('Ctrl Pts',(18.3,59.4652115046978,2.52619377374649));
#72430=CARTESIAN_POINT('',(18.18,59.3342428147793,2.75375164151192));
#72431=CARTESIAN_POINT('',(18.3,59.3342428147793,2.75375164151192));
#72432=CARTESIAN_POINT('Ctrl Pts',(18.18,59.3342428147793,2.75375164151192));
#72433=CARTESIAN_POINT('Ctrl Pts',(18.18,59.3342428147793,2.61841750741005));
#72434=CARTESIAN_POINT('Ctrl Pts',(18.18,59.4652115046978,2.52619377374649));
#72435=CARTESIAN_POINT('Ctrl Pts',(18.3,59.4646658241749,2.98130965828896));
#72436=CARTESIAN_POINT('Ctrl Pts',(18.1272,59.4646658241749,2.98130965828896));
#72437=CARTESIAN_POINT('Ctrl Pts',(18.3,59.3342428147793,2.8890859246254));
#72438=CARTESIAN_POINT('Ctrl Pts',(18.1272,59.3342428147793,2.8890859246254));
#72439=CARTESIAN_POINT('Ctrl Pts',(18.3,59.3342428147793,2.75375164151192));
#72440=CARTESIAN_POINT('Ctrl Pts',(18.1272,59.3342428147793,2.75375164151192));
#72441=CARTESIAN_POINT('',(18.3,59.4646658241749,2.98130965828896));
#72442=CARTESIAN_POINT('Ctrl Pts',(18.3,59.4646658241749,2.98130965828896));
#72443=CARTESIAN_POINT('Ctrl Pts',(18.3,59.3342428147793,2.8890859246254));
#72444=CARTESIAN_POINT('Ctrl Pts',(18.3,59.3342428147793,2.75375164151192));
#72445=CARTESIAN_POINT('',(18.18,59.4646658241749,2.98130965828896));
#72446=CARTESIAN_POINT('',(18.3,59.4646658241749,2.98130965828896));
#72447=CARTESIAN_POINT('Ctrl Pts',(18.18,59.4646658241749,2.98130965828896));
#72448=CARTESIAN_POINT('Ctrl Pts',(18.18,59.3342428147793,2.8890859246254));
#72449=CARTESIAN_POINT('Ctrl Pts',(18.18,59.3342428147793,2.75375164151192));
#72450=CARTESIAN_POINT('Ctrl Pts',(18.3,59.9890859663486,3.07353339195251));
#72451=CARTESIAN_POINT('Ctrl Pts',(18.1272,59.9890859663486,3.07353339195251));
#72452=CARTESIAN_POINT('Ctrl Pts',(18.3,59.5950888335705,3.07353339195251));
#72453=CARTESIAN_POINT('Ctrl Pts',(18.1272,59.5950888335705,3.07353339195251));
#72454=CARTESIAN_POINT('Ctrl Pts',(18.3,59.4646658241749,2.98130965828896));
#72455=CARTESIAN_POINT('Ctrl Pts',(18.1272,59.4646658241749,2.98130965828896));
#72456=CARTESIAN_POINT('',(18.3,59.9890859663486,3.07353339195251));
#72457=CARTESIAN_POINT('Ctrl Pts',(18.3,59.9890859663486,3.07353339195251));
#72458=CARTESIAN_POINT('Ctrl Pts',(18.3,59.5950888335705,3.07353339195251));
#72459=CARTESIAN_POINT('Ctrl Pts',(18.3,59.4646658241749,2.98130965828896));
#72460=CARTESIAN_POINT('',(18.18,59.9890859663486,3.07353339195251));
#72461=CARTESIAN_POINT('',(18.3,59.9890859663486,3.07353339195251));
#72462=CARTESIAN_POINT('Ctrl Pts',(18.18,59.9890859663486,3.07353339195251));
#72463=CARTESIAN_POINT('Ctrl Pts',(18.18,59.5950888335705,3.07353339195251));
#72464=CARTESIAN_POINT('Ctrl Pts',(18.18,59.4646658241749,2.98130965828896));
#72465=CARTESIAN_POINT('Ctrl Pts',(18.3,60.5293315887451,2.97203279137611));
#72466=CARTESIAN_POINT('Ctrl Pts',(18.1272,60.5293315887451,2.97203279137611));
#72467=CARTESIAN_POINT('Ctrl Pts',(18.3,60.3830830991268,3.07353339195251));
#72468=CARTESIAN_POINT('Ctrl Pts',(18.1272,60.3830830991268,3.07353339195251));
#72469=CARTESIAN_POINT('Ctrl Pts',(18.3,59.9890859663486,3.07353339195251));
#72470=CARTESIAN_POINT('Ctrl Pts',(18.1272,59.9890859663486,3.07353339195251));
#72471=CARTESIAN_POINT('Ctrl Pts',(18.3,60.5293315887451,2.97203279137611));
#72472=CARTESIAN_POINT('Ctrl Pts',(18.3,60.3830830991268,3.07353339195251));
#72473=CARTESIAN_POINT('Ctrl Pts',(18.3,59.9890859663486,3.07353339195251));
#72474=CARTESIAN_POINT('Ctrl Pts',(18.18,60.5293315887451,2.97203279137611));
#72475=CARTESIAN_POINT('Ctrl Pts',(18.18,60.3830830991268,3.07353339195251));
#72476=CARTESIAN_POINT('Ctrl Pts',(18.18,59.9890859663486,3.07353339195251));
#72477=CARTESIAN_POINT('Ctrl Pts',(18.3,59.1727148234844,2.75375164151192));
#72478=CARTESIAN_POINT('Ctrl Pts',(18.1272,59.1727148234844,2.75375164151192));
#72479=CARTESIAN_POINT('Ctrl Pts',(18.3,59.1727148234844,2.985129570961));
#72480=CARTESIAN_POINT('Ctrl Pts',(18.1272,59.1727148234844,2.985129570961));
#72481=CARTESIAN_POINT('Ctrl Pts',(18.3,59.3386085569858,3.11718962192535));
#72482=CARTESIAN_POINT('Ctrl Pts',(18.1272,59.3386085569858,3.11718962192535));
#72483=CARTESIAN_POINT('',(18.3,59.1727148234844,2.75375164151192));
#72484=CARTESIAN_POINT('',(18.3,59.3386085569858,3.11718962192535));
#72485=CARTESIAN_POINT('Ctrl Pts',(18.3,59.1727148234844,2.75375164151192));
#72486=CARTESIAN_POINT('Ctrl Pts',(18.3,59.1727148234844,2.985129570961));
#72487=CARTESIAN_POINT('Ctrl Pts',(18.3,59.3386085569858,3.11718962192535));
#72488=CARTESIAN_POINT('',(18.18,59.1727148234844,2.75375164151192));
#72489=CARTESIAN_POINT('',(18.3,59.1727148234844,2.75375164151192));
#72490=CARTESIAN_POINT('',(18.18,59.3386085569858,3.11718962192535));
#72491=CARTESIAN_POINT('Ctrl Pts',(18.18,59.1727148234844,2.75375164151192));
#72492=CARTESIAN_POINT('Ctrl Pts',(18.18,59.1727148234844,2.985129570961));
#72493=CARTESIAN_POINT('Ctrl Pts',(18.18,59.3386085569858,3.11718962192535));
#72494=CARTESIAN_POINT('',(18.3,59.3386085569858,3.11718962192535));
#72495=CARTESIAN_POINT('Ctrl Pts',(18.3,59.2671214282513,2.46289229989052));
#72496=CARTESIAN_POINT('Ctrl Pts',(18.1272,59.2671214282513,2.46289229989052));
#72497=CARTESIAN_POINT('Ctrl Pts',(18.3,59.1727148234844,2.57803550958633));
#72498=CARTESIAN_POINT('Ctrl Pts',(18.1272,59.1727148234844,2.57803550958633));
#72499=CARTESIAN_POINT('Ctrl Pts',(18.3,59.1727148234844,2.75375164151192));
#72500=CARTESIAN_POINT('Ctrl Pts',(18.1272,59.1727148234844,2.75375164151192));
#72501=CARTESIAN_POINT('',(18.3,59.2671214282513,2.46289229989052));
#72502=CARTESIAN_POINT('Ctrl Pts',(18.3,59.2671214282513,2.46289229989052));
#72503=CARTESIAN_POINT('Ctrl Pts',(18.3,59.1727148234844,2.57803550958633));
#72504=CARTESIAN_POINT('Ctrl Pts',(18.3,59.1727148234844,2.75375164151192));
#72505=CARTESIAN_POINT('',(18.18,59.2671214282513,2.46289229989052));
#72506=CARTESIAN_POINT('',(18.3,59.2671214282513,2.46289229989052));
#72507=CARTESIAN_POINT('Ctrl Pts',(18.18,59.2671214282513,2.46289229989052));
#72508=CARTESIAN_POINT('Ctrl Pts',(18.18,59.1727148234844,2.57803550958633));
#72509=CARTESIAN_POINT('Ctrl Pts',(18.18,59.1727148234844,2.75375164151192));
#72510=CARTESIAN_POINT('Ctrl Pts',(18.3,59.5345156133175,2.28990457057953));
#72511=CARTESIAN_POINT('Ctrl Pts',(18.1272,59.5345156133175,2.28990457057953));
#72512=CARTESIAN_POINT('Ctrl Pts',(18.3,59.3615280330181,2.34774894118309));
#72513=CARTESIAN_POINT('Ctrl Pts',(18.1272,59.3615280330181,2.34774894118309));
#72514=CARTESIAN_POINT('Ctrl Pts',(18.3,59.2671214282513,2.46289229989052));
#72515=CARTESIAN_POINT('Ctrl Pts',(18.1272,59.2671214282513,2.46289229989052));
#72516=CARTESIAN_POINT('',(18.3,59.5345156133175,2.28990457057953));
#72517=CARTESIAN_POINT('Ctrl Pts',(18.3,59.5345156133175,2.28990457057953));
#72518=CARTESIAN_POINT('Ctrl Pts',(18.3,59.3615280330181,2.34774894118309));
#72519=CARTESIAN_POINT('Ctrl Pts',(18.3,59.2671214282513,2.46289229989052));
#72520=CARTESIAN_POINT('',(18.18,59.5345156133175,2.28990457057953));
#72521=CARTESIAN_POINT('',(18.3,59.5345156133175,2.28990457057953));
#72522=CARTESIAN_POINT('Ctrl Pts',(18.18,59.5345156133175,2.28990457057953));
#72523=CARTESIAN_POINT('Ctrl Pts',(18.18,59.3615280330181,2.34774894118309));
#72524=CARTESIAN_POINT('Ctrl Pts',(18.18,59.2671214282513,2.46289229989052));
#72525=CARTESIAN_POINT('Ctrl Pts',(18.3,59.9890859663486,2.23206005096436));
#72526=CARTESIAN_POINT('Ctrl Pts',(18.1272,59.9890859663486,2.23206005096436));
#72527=CARTESIAN_POINT('Ctrl Pts',(18.3,59.7075034916401,2.23206005096436));
#72528=CARTESIAN_POINT('Ctrl Pts',(18.1272,59.7075034916401,2.23206005096436));
#72529=CARTESIAN_POINT('Ctrl Pts',(18.3,59.5345156133175,2.28990457057953));
#72530=CARTESIAN_POINT('Ctrl Pts',(18.1272,59.5345156133175,2.28990457057953));
#72531=CARTESIAN_POINT('',(18.3,59.9890859663486,2.23206005096436));
#72532=CARTESIAN_POINT('Ctrl Pts',(18.3,59.9890859663486,2.23206005096436));
#72533=CARTESIAN_POINT('Ctrl Pts',(18.3,59.7075034916401,2.23206005096436));
#72534=CARTESIAN_POINT('Ctrl Pts',(18.3,59.5345156133175,2.28990457057953));
#72535=CARTESIAN_POINT('',(18.18,59.9890859663486,2.23206005096436));
#72536=CARTESIAN_POINT('',(18.3,59.9890859663486,2.23206005096436));
#72537=CARTESIAN_POINT('Ctrl Pts',(18.18,59.9890859663486,2.23206005096436));
#72538=CARTESIAN_POINT('Ctrl Pts',(18.18,59.7075034916401,2.23206005096436));
#72539=CARTESIAN_POINT('Ctrl Pts',(18.18,59.5345156133175,2.28990457057953));
#72540=CARTESIAN_POINT('Ctrl Pts',(18.3,60.3672577679157,2.26807645559311));
#72541=CARTESIAN_POINT('Ctrl Pts',(18.1272,60.3672577679157,2.26807645559311));
#72542=CARTESIAN_POINT('Ctrl Pts',(18.3,60.2270122110844,2.23206005096436));
#72543=CARTESIAN_POINT('Ctrl Pts',(18.1272,60.2270122110844,2.23206005096436));
#72544=CARTESIAN_POINT('Ctrl Pts',(18.3,59.9890859663486,2.23206005096436));
#72545=CARTESIAN_POINT('Ctrl Pts',(18.1272,59.9890859663486,2.23206005096436));
#72546=CARTESIAN_POINT('',(18.3,60.3672577679157,2.26807645559311));
#72547=CARTESIAN_POINT('Ctrl Pts',(18.3,60.3672577679157,2.26807645559311));
#72548=CARTESIAN_POINT('Ctrl Pts',(18.3,60.2270122110844,2.23206005096436));
#72549=CARTESIAN_POINT('Ctrl Pts',(18.3,59.9890859663486,2.23206005096436));
#72550=CARTESIAN_POINT('',(18.18,60.3672577679157,2.26807645559311));
#72551=CARTESIAN_POINT('',(18.3,60.3672577679157,2.26807645559311));
#72552=CARTESIAN_POINT('Ctrl Pts',(18.18,60.3672577679157,2.26807645559311));
#72553=CARTESIAN_POINT('Ctrl Pts',(18.18,60.2270122110844,2.23206005096436));
#72554=CARTESIAN_POINT('Ctrl Pts',(18.18,59.9890859663486,2.23206005096436));
#72555=CARTESIAN_POINT('Ctrl Pts',(18.3,60.605184161663,2.36739433407783));
#72556=CARTESIAN_POINT('Ctrl Pts',(18.1272,60.605184161663,2.36739433407783));
#72557=CARTESIAN_POINT('Ctrl Pts',(18.3,60.5075034737587,2.30409256219864));
#72558=CARTESIAN_POINT('Ctrl Pts',(18.1272,60.5075034737587,2.30409256219864));
#72559=CARTESIAN_POINT('Ctrl Pts',(18.3,60.3672577679157,2.26807645559311));
#72560=CARTESIAN_POINT('Ctrl Pts',(18.1272,60.3672577679157,2.26807645559311));
#72561=CARTESIAN_POINT('',(18.3,60.605184161663,2.36739433407783));
#72562=CARTESIAN_POINT('Ctrl Pts',(18.3,60.605184161663,2.36739433407783));
#72563=CARTESIAN_POINT('Ctrl Pts',(18.3,60.5075034737587,2.30409256219864));
#72564=CARTESIAN_POINT('Ctrl Pts',(18.3,60.3672577679157,2.26807645559311));
#72565=CARTESIAN_POINT('',(18.18,60.605184161663,2.36739433407783));
#72566=CARTESIAN_POINT('',(18.3,60.605184161663,2.36739433407783));
#72567=CARTESIAN_POINT('Ctrl Pts',(18.18,60.605184161663,2.36739433407783));
#72568=CARTESIAN_POINT('Ctrl Pts',(18.18,60.5075034737587,2.30409256219864));
#72569=CARTESIAN_POINT('Ctrl Pts',(18.18,60.3672577679157,2.26807645559311));
#72570=CARTESIAN_POINT('Ctrl Pts',(18.3,60.7547067344189,2.52783096432686));
#72571=CARTESIAN_POINT('Ctrl Pts',(18.1272,60.7547067344189,2.52783096432686));
#72572=CARTESIAN_POINT('Ctrl Pts',(18.3,60.702864998579,2.43069580793381));
#72573=CARTESIAN_POINT('Ctrl Pts',(18.1272,60.702864998579,2.43069580793381));
#72574=CARTESIAN_POINT('Ctrl Pts',(18.3,60.605184161663,2.36739433407783));
#72575=CARTESIAN_POINT('Ctrl Pts',(18.1272,60.605184161663,2.36739433407783));
#72576=CARTESIAN_POINT('',(18.3,60.7547067344189,2.52783096432686));
#72577=CARTESIAN_POINT('Ctrl Pts',(18.3,60.7547067344189,2.52783096432686));
#72578=CARTESIAN_POINT('Ctrl Pts',(18.3,60.702864998579,2.43069580793381));
#72579=CARTESIAN_POINT('Ctrl Pts',(18.3,60.605184161663,2.36739433407783));
#72580=CARTESIAN_POINT('',(18.18,60.7547067344189,2.52783096432686));
#72581=CARTESIAN_POINT('',(18.3,60.7547067344189,2.52783096432686));
#72582=CARTESIAN_POINT('Ctrl Pts',(18.18,60.7547067344189,2.52783096432686));
#72583=CARTESIAN_POINT('Ctrl Pts',(18.18,60.702864998579,2.43069580793381));
#72584=CARTESIAN_POINT('Ctrl Pts',(18.18,60.605184161663,2.36739433407783));
#72585=CARTESIAN_POINT('Ctrl Pts',(18.3,60.8065484702587,2.75375164151192));
#72586=CARTESIAN_POINT('Ctrl Pts',(18.1272,60.8065484702587,2.75375164151192));
#72587=CARTESIAN_POINT('Ctrl Pts',(18.3,60.8065484702587,2.6249659717083));
#72588=CARTESIAN_POINT('Ctrl Pts',(18.1272,60.8065484702587,2.6249659717083));
#72589=CARTESIAN_POINT('Ctrl Pts',(18.3,60.7547067344189,2.52783096432686));
#72590=CARTESIAN_POINT('Ctrl Pts',(18.1272,60.7547067344189,2.52783096432686));
#72591=CARTESIAN_POINT('',(18.3,60.8065484702587,2.75375164151192));
#72592=CARTESIAN_POINT('Ctrl Pts',(18.3,60.8065484702587,2.75375164151192));
#72593=CARTESIAN_POINT('Ctrl Pts',(18.3,60.8065484702587,2.6249659717083));
#72594=CARTESIAN_POINT('Ctrl Pts',(18.3,60.7547067344189,2.52783096432686));
#72595=CARTESIAN_POINT('',(18.18,60.8065484702587,2.75375164151192));
#72596=CARTESIAN_POINT('',(18.3,60.8065484702587,2.75375164151192));
#72597=CARTESIAN_POINT('Ctrl Pts',(18.18,60.8065484702587,2.75375164151192));
#72598=CARTESIAN_POINT('Ctrl Pts',(18.18,60.8065484702587,2.6249659717083));
#72599=CARTESIAN_POINT('Ctrl Pts',(18.18,60.7547067344189,2.52783096432686));
#72600=CARTESIAN_POINT('Ctrl Pts',(18.3,60.7126876950264,3.04351977109909));
#72601=CARTESIAN_POINT('Ctrl Pts',(18.1272,60.7126876950264,3.04351977109909));
#72602=CARTESIAN_POINT('Ctrl Pts',(18.3,60.8065484702587,2.92837656140327));
#72603=CARTESIAN_POINT('Ctrl Pts',(18.1272,60.8065484702587,2.92837656140327));
#72604=CARTESIAN_POINT('Ctrl Pts',(18.3,60.8065484702587,2.75375164151192));
#72605=CARTESIAN_POINT('Ctrl Pts',(18.1272,60.8065484702587,2.75375164151192));
#72606=CARTESIAN_POINT('',(18.3,60.7126876950264,3.04351977109909));
#72607=CARTESIAN_POINT('Ctrl Pts',(18.3,60.7126876950264,3.04351977109909));
#72608=CARTESIAN_POINT('Ctrl Pts',(18.3,60.8065484702587,2.92837656140327));
#72609=CARTESIAN_POINT('Ctrl Pts',(18.3,60.8065484702587,2.75375164151192));
#72610=CARTESIAN_POINT('',(18.18,60.7126876950264,3.04351977109909));
#72611=CARTESIAN_POINT('',(18.3,60.7126876950264,3.04351977109909));
#72612=CARTESIAN_POINT('Ctrl Pts',(18.18,60.7126876950264,3.04351977109909));
#72613=CARTESIAN_POINT('Ctrl Pts',(18.18,60.8065484702587,2.92837656140327));
#72614=CARTESIAN_POINT('Ctrl Pts',(18.18,60.8065484702587,2.75375164151192));
#72615=CARTESIAN_POINT('Ctrl Pts',(18.3,60.4458390414715,3.217053180933));
#72616=CARTESIAN_POINT('Ctrl Pts',(18.1272,60.4458390414715,3.217053180933));
#72617=CARTESIAN_POINT('Ctrl Pts',(18.3,60.6188267707825,3.15866298079491));
#72618=CARTESIAN_POINT('Ctrl Pts',(18.1272,60.6188267707825,3.15866298079491));
#72619=CARTESIAN_POINT('Ctrl Pts',(18.3,60.7126876950264,3.04351977109909));
#72620=CARTESIAN_POINT('Ctrl Pts',(18.1272,60.7126876950264,3.04351977109909));
#72621=CARTESIAN_POINT('',(18.3,60.4458390414715,3.217053180933));
#72622=CARTESIAN_POINT('Ctrl Pts',(18.3,60.4458390414715,3.217053180933));
#72623=CARTESIAN_POINT('Ctrl Pts',(18.3,60.6188267707825,3.15866298079491));
#72624=CARTESIAN_POINT('Ctrl Pts',(18.3,60.7126876950264,3.04351977109909));
#72625=CARTESIAN_POINT('',(18.18,60.4458390414715,3.217053180933));
#72626=CARTESIAN_POINT('',(18.3,60.4458390414715,3.217053180933));
#72627=CARTESIAN_POINT('Ctrl Pts',(18.18,60.4458390414715,3.217053180933));
#72628=CARTESIAN_POINT('Ctrl Pts',(18.18,60.6188267707825,3.15866298079491));
#72629=CARTESIAN_POINT('Ctrl Pts',(18.18,60.7126876950264,3.04351977109909));
#72630=CARTESIAN_POINT('Ctrl Pts',(18.3,59.9890859663486,3.27544338107109));
#72631=CARTESIAN_POINT('Ctrl Pts',(18.1272,59.9890859663486,3.27544338107109));
#72632=CARTESIAN_POINT('Ctrl Pts',(18.3,60.2728513121605,3.27544338107109));
#72633=CARTESIAN_POINT('Ctrl Pts',(18.1272,60.2728513121605,3.27544338107109));
#72634=CARTESIAN_POINT('Ctrl Pts',(18.3,60.4458390414715,3.217053180933));
#72635=CARTESIAN_POINT('Ctrl Pts',(18.1272,60.4458390414715,3.217053180933));
#72636=CARTESIAN_POINT('',(18.3,59.9890859663486,3.27544338107109));
#72637=CARTESIAN_POINT('Ctrl Pts',(18.3,59.9890859663486,3.27544338107109));
#72638=CARTESIAN_POINT('Ctrl Pts',(18.3,60.2728513121605,3.27544338107109));
#72639=CARTESIAN_POINT('Ctrl Pts',(18.3,60.4458390414715,3.217053180933));
#72640=CARTESIAN_POINT('',(18.18,59.9890859663486,3.27544338107109));
#72641=CARTESIAN_POINT('',(18.3,59.9890859663486,3.27544338107109));
#72642=CARTESIAN_POINT('Ctrl Pts',(18.18,59.9890859663486,3.27544338107109));
#72643=CARTESIAN_POINT('Ctrl Pts',(18.18,60.2728513121605,3.27544338107109));
#72644=CARTESIAN_POINT('Ctrl Pts',(18.18,60.4458390414715,3.217053180933));
#72645=CARTESIAN_POINT('Ctrl Pts',(18.3,59.3386085569858,3.11718962192535));
#72646=CARTESIAN_POINT('Ctrl Pts',(18.1272,59.3386085569858,3.11718962192535));
#72647=CARTESIAN_POINT('Ctrl Pts',(18.3,59.5383356750011,3.27544338107109));
#72648=CARTESIAN_POINT('Ctrl Pts',(18.1272,59.5383356750011,3.27544338107109));
#72649=CARTESIAN_POINT('Ctrl Pts',(18.3,59.9890859663486,3.27544338107109));
#72650=CARTESIAN_POINT('Ctrl Pts',(18.1272,59.9890859663486,3.27544338107109));
#72651=CARTESIAN_POINT('Ctrl Pts',(18.3,59.3386085569858,3.11718962192535));
#72652=CARTESIAN_POINT('Ctrl Pts',(18.3,59.5383356750011,3.27544338107109));
#72653=CARTESIAN_POINT('Ctrl Pts',(18.3,59.9890859663486,3.27544338107109));
#72654=CARTESIAN_POINT('Ctrl Pts',(18.18,59.3386085569858,3.11718962192535));
#72655=CARTESIAN_POINT('Ctrl Pts',(18.18,59.5383356750011,3.27544338107109));
#72656=CARTESIAN_POINT('Ctrl Pts',(18.18,59.9890859663486,3.27544338107109));
#72657=CARTESIAN_POINT('Origin',(18.18,59.9896316468716,3.29999997317791));
#72658=CARTESIAN_POINT('Origin',(18.3,60.8065484702587,3.90518411099911));
#72659=CARTESIAN_POINT('',(18.3,60.8065484702587,3.90518411099911));
#72660=CARTESIAN_POINT('',(18.3,60.8065484702587,3.77858108878136));
#72661=CARTESIAN_POINT('',(18.3,60.8065484702587,4.70259205549955));
#72662=CARTESIAN_POINT('',(18.18,60.8065484702587,3.90518411099911));
#72663=CARTESIAN_POINT('',(18.3,60.8065484702587,3.90518411099911));
#72664=CARTESIAN_POINT('',(18.18,60.8065484702587,3.77858108878136));
#72665=CARTESIAN_POINT('',(18.18,60.8065484702587,3.90518411099911));
#72666=CARTESIAN_POINT('',(18.3,60.8065484702587,3.77858108878136));
#72667=CARTESIAN_POINT('Ctrl Pts',(18.3,60.5926330626011,4.07980895638466));
#72668=CARTESIAN_POINT('Ctrl Pts',(18.1272,60.5926330626011,4.07980895638466));
#72669=CARTESIAN_POINT('Ctrl Pts',(18.3,60.702864998579,3.95648016631603));
#72670=CARTESIAN_POINT('Ctrl Pts',(18.1272,60.702864998579,3.95648016631603));
#72671=CARTESIAN_POINT('Ctrl Pts',(18.3,60.8065484702587,3.90518411099911));
#72672=CARTESIAN_POINT('Ctrl Pts',(18.1272,60.8065484702587,3.90518411099911));
#72673=CARTESIAN_POINT('',(18.3,60.5926330626011,4.07980895638466));
#72674=CARTESIAN_POINT('Ctrl Pts',(18.3,60.5926330626011,4.07980895638466));
#72675=CARTESIAN_POINT('Ctrl Pts',(18.3,60.702864998579,3.95648016631603));
#72676=CARTESIAN_POINT('Ctrl Pts',(18.3,60.8065484702587,3.90518411099911));
#72677=CARTESIAN_POINT('',(18.18,60.5926330626011,4.07980895638466));
#72678=CARTESIAN_POINT('',(18.3,60.5926330626011,4.07980895638466));
#72679=CARTESIAN_POINT('Ctrl Pts',(18.18,60.5926330626011,4.07980895638466));
#72680=CARTESIAN_POINT('Ctrl Pts',(18.18,60.702864998579,3.95648016631603));
#72681=CARTESIAN_POINT('Ctrl Pts',(18.18,60.8065484702587,3.90518411099911));
#72682=CARTESIAN_POINT('Ctrl Pts',(18.3,60.4049113631248,4.36793989539146));
#72683=CARTESIAN_POINT('Ctrl Pts',(18.1272,60.4049113631248,4.36793989539146));
#72684=CARTESIAN_POINT('Ctrl Pts',(18.3,60.4824011266231,4.20313774645328));
#72685=CARTESIAN_POINT('Ctrl Pts',(18.1272,60.4824011266231,4.20313774645328));
#72686=CARTESIAN_POINT('Ctrl Pts',(18.3,60.5926330626011,4.07980895638466));
#72687=CARTESIAN_POINT('Ctrl Pts',(18.1272,60.5926330626011,4.07980895638466));
#72688=CARTESIAN_POINT('',(18.3,60.4049113631248,4.36793989539146));
#72689=CARTESIAN_POINT('Ctrl Pts',(18.3,60.4049113631248,4.36793989539146));
#72690=CARTESIAN_POINT('Ctrl Pts',(18.3,60.4824011266231,4.20313774645328));
#72691=CARTESIAN_POINT('Ctrl Pts',(18.3,60.5926330626011,4.07980895638466));
#72692=CARTESIAN_POINT('',(18.18,60.4049113631248,4.36793989539146));
#72693=CARTESIAN_POINT('',(18.3,60.4049113631248,4.36793989539146));
#72694=CARTESIAN_POINT('Ctrl Pts',(18.18,60.4049113631248,4.36793989539146));
#72695=CARTESIAN_POINT('Ctrl Pts',(18.18,60.4824011266231,4.20313774645328));
#72696=CARTESIAN_POINT('Ctrl Pts',(18.18,60.5926330626011,4.07980895638466));
#72697=CARTESIAN_POINT('Origin',(18.3,60.2150069415569,4.36793989539146));
#72698=CARTESIAN_POINT('',(18.3,60.2150069415569,4.36793989539146));
#72699=CARTESIAN_POINT('',(18.3,65.1075034707785,4.36793989539146));
#72700=CARTESIAN_POINT('',(18.18,60.2150069415569,4.36793989539146));
#72701=CARTESIAN_POINT('',(18.3,60.2150069415569,4.36793989539146));
#72702=CARTESIAN_POINT('',(18.18,60.2150069415569,4.36793989539146));
#72703=CARTESIAN_POINT('Ctrl Pts',(18.3,60.3165075421333,4.16111863255501));
#72704=CARTESIAN_POINT('Ctrl Pts',(18.1272,60.3165075421333,4.16111863255501));
#72705=CARTESIAN_POINT('Ctrl Pts',(18.3,60.2488404750824,4.27626184225082));
#72706=CARTESIAN_POINT('Ctrl Pts',(18.1272,60.2488404750824,4.27626184225082));
#72707=CARTESIAN_POINT('Ctrl Pts',(18.3,60.2150069415569,4.36793989539146));
#72708=CARTESIAN_POINT('Ctrl Pts',(18.1272,60.2150069415569,4.36793989539146));
#72709=CARTESIAN_POINT('',(18.3,60.3165075421333,4.16111863255501));
#72710=CARTESIAN_POINT('Ctrl Pts',(18.3,60.3165075421333,4.16111863255501));
#72711=CARTESIAN_POINT('Ctrl Pts',(18.3,60.2488404750824,4.27626184225082));
#72712=CARTESIAN_POINT('Ctrl Pts',(18.3,60.2150069415569,4.36793989539146));
#72713=CARTESIAN_POINT('',(18.18,60.3165075421333,4.16111863255501));
#72714=CARTESIAN_POINT('',(18.3,60.3165075421333,4.16111863255501));
#72715=CARTESIAN_POINT('Ctrl Pts',(18.18,60.3165075421333,4.16111863255501));
#72716=CARTESIAN_POINT('Ctrl Pts',(18.18,60.2488404750824,4.27626184225082));
#72717=CARTESIAN_POINT('Ctrl Pts',(18.18,60.2150069415569,4.36793989539146));
#72718=CARTESIAN_POINT('Ctrl Pts',(18.3,60.4518418252468,3.97503404915333));
#72719=CARTESIAN_POINT('Ctrl Pts',(18.1272,60.4518418252468,3.97503404915333));
#72720=CARTESIAN_POINT('Ctrl Pts',(18.3,60.3841747581959,4.04597542285919));
#72721=CARTESIAN_POINT('Ctrl Pts',(18.1272,60.3841747581959,4.04597542285919));
#72722=CARTESIAN_POINT('Ctrl Pts',(18.3,60.3165075421333,4.16111863255501));
#72723=CARTESIAN_POINT('Ctrl Pts',(18.1272,60.3165075421333,4.16111863255501));
#72724=CARTESIAN_POINT('',(18.3,60.4518418252468,3.97503404915333));
#72725=CARTESIAN_POINT('Ctrl Pts',(18.3,60.4518418252468,3.97503404915333));
#72726=CARTESIAN_POINT('Ctrl Pts',(18.3,60.3841747581959,4.04597542285919));
#72727=CARTESIAN_POINT('Ctrl Pts',(18.3,60.3165075421333,4.16111863255501));
#72728=CARTESIAN_POINT('',(18.18,60.4518418252468,3.97503404915333));
#72729=CARTESIAN_POINT('',(18.3,60.4518418252468,3.97503404915333));
#72730=CARTESIAN_POINT('Ctrl Pts',(18.18,60.4518418252468,3.97503404915333));
#72731=CARTESIAN_POINT('Ctrl Pts',(18.18,60.3841747581959,4.04597542285919));
#72732=CARTESIAN_POINT('Ctrl Pts',(18.18,60.3165075421333,4.16111863255501));
#72733=CARTESIAN_POINT('Origin',(18.3,59.2000000417232,3.97503404915333));
#72734=CARTESIAN_POINT('',(18.3,59.2000000417232,3.97503404915333));
#72735=CARTESIAN_POINT('',(18.3,64.6000000208616,3.97503404915333));
#72736=CARTESIAN_POINT('',(18.18,59.2000000417232,3.97503404915333));
#72737=CARTESIAN_POINT('',(18.3,59.2000000417232,3.97503404915333));
#72738=CARTESIAN_POINT('',(18.18,59.2000000417232,3.97503404915333));
#72739=CARTESIAN_POINT('Origin',(18.3,59.2000000417232,3.77858108878136));
#72740=CARTESIAN_POINT('',(18.3,59.2000000417232,3.77858108878136));
#72741=CARTESIAN_POINT('',(18.3,59.2000000417232,4.63929054439068));
#72742=CARTESIAN_POINT('',(18.18,59.2000000417232,3.77858108878136));
#72743=CARTESIAN_POINT('',(18.3,59.2000000417232,3.77858108878136));
#72744=CARTESIAN_POINT('',(18.18,59.2000000417232,3.77858108878136));
#72745=CARTESIAN_POINT('Origin',(18.3,60.8065484702587,3.77858108878136));
#72746=CARTESIAN_POINT('',(18.3,65.4032742351294,3.77858108878136));
#72747=CARTESIAN_POINT('',(18.18,60.8065484702587,3.77858108878136));
#72748=CARTESIAN_POINT('Origin',(18.18,59.9896316468716,3.29999997317791));
#72749=CARTESIAN_POINT('Origin',(18.3,70.,5.5));
#72750=CARTESIAN_POINT('Ctrl Pts',(18.3,50.643929117918,2.66698497384787));
#72751=CARTESIAN_POINT('Ctrl Pts',(18.1272,50.643929117918,2.66698497384787));
#72752=CARTESIAN_POINT('Ctrl Pts',(18.3,50.643929117918,2.80231925696135));
#72753=CARTESIAN_POINT('Ctrl Pts',(18.1272,50.643929117918,2.80231925696135));
#72754=CARTESIAN_POINT('Ctrl Pts',(18.3,50.5293315887451,2.88308325260878));
#72755=CARTESIAN_POINT('Ctrl Pts',(18.1272,50.5293315887451,2.88308325260878));
#72756=CARTESIAN_POINT('',(18.3,50.643929117918,2.66698497384787));
#72757=CARTESIAN_POINT('',(18.3,50.5293315887451,2.88308325260878));
#72758=CARTESIAN_POINT('Ctrl Pts',(18.3,50.643929117918,2.66698497384787));
#72759=CARTESIAN_POINT('Ctrl Pts',(18.3,50.643929117918,2.80231925696135));
#72760=CARTESIAN_POINT('Ctrl Pts',(18.3,50.5293315887451,2.88308325260878));
#72761=CARTESIAN_POINT('',(18.18,50.643929117918,2.66698497384787));
#72762=CARTESIAN_POINT('',(18.3,50.643929117918,2.66698497384787));
#72763=CARTESIAN_POINT('',(18.18,50.5293315887451,2.88308325260878));
#72764=CARTESIAN_POINT('Ctrl Pts',(18.18,50.643929117918,2.66698497384787));
#72765=CARTESIAN_POINT('Ctrl Pts',(18.18,50.643929117918,2.80231925696135));
#72766=CARTESIAN_POINT('Ctrl Pts',(18.18,50.5293315887451,2.88308325260878));
#72767=CARTESIAN_POINT('',(18.3,50.5293315887451,2.88308325260878));
#72768=CARTESIAN_POINT('Ctrl Pts',(18.3,50.5140519380569,2.43724423497915));
#72769=CARTESIAN_POINT('Ctrl Pts',(18.1272,50.5140519380569,2.43724423497915));
#72770=CARTESIAN_POINT('Ctrl Pts',(18.3,50.643929117918,2.52946796864271));
#72771=CARTESIAN_POINT('Ctrl Pts',(18.1272,50.643929117918,2.52946796864271));
#72772=CARTESIAN_POINT('Ctrl Pts',(18.3,50.643929117918,2.66698497384787));
#72773=CARTESIAN_POINT('Ctrl Pts',(18.1272,50.643929117918,2.66698497384787));
#72774=CARTESIAN_POINT('',(18.3,50.5140519380569,2.43724423497915));
#72775=CARTESIAN_POINT('Ctrl Pts',(18.3,50.5140519380569,2.43724423497915));
#72776=CARTESIAN_POINT('Ctrl Pts',(18.3,50.643929117918,2.52946796864271));
#72777=CARTESIAN_POINT('Ctrl Pts',(18.3,50.643929117918,2.66698497384787));
#72778=CARTESIAN_POINT('',(18.18,50.5140519380569,2.43724423497915));
#72779=CARTESIAN_POINT('',(18.3,50.5140519380569,2.43724423497915));
#72780=CARTESIAN_POINT('Ctrl Pts',(18.18,50.5140519380569,2.43724423497915));
#72781=CARTESIAN_POINT('Ctrl Pts',(18.18,50.643929117918,2.52946796864271));
#72782=CARTESIAN_POINT('Ctrl Pts',(18.18,50.643929117918,2.66698497384787));
#72783=CARTESIAN_POINT('Ctrl Pts',(18.3,49.9890859663486,2.34502050131559));
#72784=CARTESIAN_POINT('Ctrl Pts',(18.1272,49.9890859663486,2.34502050131559));
#72785=CARTESIAN_POINT('Ctrl Pts',(18.3,50.3841746091843,2.34502050131559));
#72786=CARTESIAN_POINT('Ctrl Pts',(18.1272,50.3841746091843,2.34502050131559));
#72787=CARTESIAN_POINT('Ctrl Pts',(18.3,50.5140519380569,2.43724423497915));
#72788=CARTESIAN_POINT('Ctrl Pts',(18.1272,50.5140519380569,2.43724423497915));
#72789=CARTESIAN_POINT('',(18.3,49.9890859663486,2.34502050131559));
#72790=CARTESIAN_POINT('Ctrl Pts',(18.3,49.9890859663486,2.34502050131559));
#72791=CARTESIAN_POINT('Ctrl Pts',(18.3,50.3841746091843,2.34502050131559));
#72792=CARTESIAN_POINT('Ctrl Pts',(18.3,50.5140519380569,2.43724423497915));
#72793=CARTESIAN_POINT('',(18.18,49.9890859663486,2.34502050131559));
#72794=CARTESIAN_POINT('',(18.3,49.9890859663486,2.34502050131559));
#72795=CARTESIAN_POINT('Ctrl Pts',(18.18,49.9890859663486,2.34502050131559));
#72796=CARTESIAN_POINT('Ctrl Pts',(18.18,50.3841746091843,2.34502050131559));
#72797=CARTESIAN_POINT('Ctrl Pts',(18.18,50.5140519380569,2.43724423497915));
#72798=CARTESIAN_POINT('Ctrl Pts',(18.3,49.4652115046978,2.43724423497915));
#72799=CARTESIAN_POINT('Ctrl Pts',(18.1272,49.4652115046978,2.43724423497915));
#72800=CARTESIAN_POINT('Ctrl Pts',(18.3,49.5961801946163,2.34502050131559));
#72801=CARTESIAN_POINT('Ctrl Pts',(18.1272,49.5961801946163,2.34502050131559));
#72802=CARTESIAN_POINT('Ctrl Pts',(18.3,49.9890859663486,2.34502050131559));
#72803=CARTESIAN_POINT('Ctrl Pts',(18.1272,49.9890859663486,2.34502050131559));
#72804=CARTESIAN_POINT('',(18.3,49.4652115046978,2.43724423497915));
#72805=CARTESIAN_POINT('Ctrl Pts',(18.3,49.4652115046978,2.43724423497915));
#72806=CARTESIAN_POINT('Ctrl Pts',(18.3,49.5961801946163,2.34502050131559));
#72807=CARTESIAN_POINT('Ctrl Pts',(18.3,49.9890859663486,2.34502050131559));
#72808=CARTESIAN_POINT('',(18.18,49.4652115046978,2.43724423497915));
#72809=CARTESIAN_POINT('',(18.3,49.4652115046978,2.43724423497915));
#72810=CARTESIAN_POINT('Ctrl Pts',(18.18,49.4652115046978,2.43724423497915));
#72811=CARTESIAN_POINT('Ctrl Pts',(18.18,49.5961801946163,2.34502050131559));
#72812=CARTESIAN_POINT('Ctrl Pts',(18.18,49.9890859663486,2.34502050131559));
#72813=CARTESIAN_POINT('Ctrl Pts',(18.3,49.3342428147793,2.66480210274458));
#72814=CARTESIAN_POINT('Ctrl Pts',(18.1272,49.3342428147793,2.66480210274458));
#72815=CARTESIAN_POINT('Ctrl Pts',(18.3,49.3342428147793,2.52946796864271));
#72816=CARTESIAN_POINT('Ctrl Pts',(18.1272,49.3342428147793,2.52946796864271));
#72817=CARTESIAN_POINT('Ctrl Pts',(18.3,49.4652115046978,2.43724423497915));
#72818=CARTESIAN_POINT('Ctrl Pts',(18.1272,49.4652115046978,2.43724423497915));
#72819=CARTESIAN_POINT('',(18.3,49.3342428147793,2.66480210274458));
#72820=CARTESIAN_POINT('Ctrl Pts',(18.3,49.3342428147793,2.66480210274458));
#72821=CARTESIAN_POINT('Ctrl Pts',(18.3,49.3342428147793,2.52946796864271));
#72822=CARTESIAN_POINT('Ctrl Pts',(18.3,49.4652115046978,2.43724423497915));
#72823=CARTESIAN_POINT('',(18.18,49.3342428147793,2.66480210274458));
#72824=CARTESIAN_POINT('',(18.3,49.3342428147793,2.66480210274458));
#72825=CARTESIAN_POINT('Ctrl Pts',(18.18,49.3342428147793,2.66480210274458));
#72826=CARTESIAN_POINT('Ctrl Pts',(18.18,49.3342428147793,2.52946796864271));
#72827=CARTESIAN_POINT('Ctrl Pts',(18.18,49.4652115046978,2.43724423497915));
#72828=CARTESIAN_POINT('Ctrl Pts',(18.3,49.4646658241749,2.89236011952162));
#72829=CARTESIAN_POINT('Ctrl Pts',(18.1272,49.4646658241749,2.89236011952162));
#72830=CARTESIAN_POINT('Ctrl Pts',(18.3,49.3342428147793,2.80013638585806));
#72831=CARTESIAN_POINT('Ctrl Pts',(18.1272,49.3342428147793,2.80013638585806));
#72832=CARTESIAN_POINT('Ctrl Pts',(18.3,49.3342428147793,2.66480210274458));
#72833=CARTESIAN_POINT('Ctrl Pts',(18.1272,49.3342428147793,2.66480210274458));
#72834=CARTESIAN_POINT('',(18.3,49.4646658241749,2.89236011952162));
#72835=CARTESIAN_POINT('Ctrl Pts',(18.3,49.4646658241749,2.89236011952162));
#72836=CARTESIAN_POINT('Ctrl Pts',(18.3,49.3342428147793,2.80013638585806));
#72837=CARTESIAN_POINT('Ctrl Pts',(18.3,49.3342428147793,2.66480210274458));
#72838=CARTESIAN_POINT('',(18.18,49.4646658241749,2.89236011952162));
#72839=CARTESIAN_POINT('',(18.3,49.4646658241749,2.89236011952162));
#72840=CARTESIAN_POINT('Ctrl Pts',(18.18,49.4646658241749,2.89236011952162));
#72841=CARTESIAN_POINT('Ctrl Pts',(18.18,49.3342428147793,2.80013638585806));
#72842=CARTESIAN_POINT('Ctrl Pts',(18.18,49.3342428147793,2.66480210274458));
#72843=CARTESIAN_POINT('Ctrl Pts',(18.3,49.9890859663486,2.98458385318518));
#72844=CARTESIAN_POINT('Ctrl Pts',(18.1272,49.9890859663486,2.98458385318518));
#72845=CARTESIAN_POINT('Ctrl Pts',(18.3,49.5950888335705,2.98458385318518));
#72846=CARTESIAN_POINT('Ctrl Pts',(18.1272,49.5950888335705,2.98458385318518));
#72847=CARTESIAN_POINT('Ctrl Pts',(18.3,49.4646658241749,2.89236011952162));
#72848=CARTESIAN_POINT('Ctrl Pts',(18.1272,49.4646658241749,2.89236011952162));
#72849=CARTESIAN_POINT('',(18.3,49.9890859663486,2.98458385318518));
#72850=CARTESIAN_POINT('Ctrl Pts',(18.3,49.9890859663486,2.98458385318518));
#72851=CARTESIAN_POINT('Ctrl Pts',(18.3,49.5950888335705,2.98458385318518));
#72852=CARTESIAN_POINT('Ctrl Pts',(18.3,49.4646658241749,2.89236011952162));
#72853=CARTESIAN_POINT('',(18.18,49.9890859663486,2.98458385318518));
#72854=CARTESIAN_POINT('',(18.3,49.9890859663486,2.98458385318518));
#72855=CARTESIAN_POINT('Ctrl Pts',(18.18,49.9890859663486,2.98458385318518));
#72856=CARTESIAN_POINT('Ctrl Pts',(18.18,49.5950888335705,2.98458385318518));
#72857=CARTESIAN_POINT('Ctrl Pts',(18.18,49.4646658241749,2.89236011952162));
#72858=CARTESIAN_POINT('Ctrl Pts',(18.3,50.5293315887451,2.88308325260878));
#72859=CARTESIAN_POINT('Ctrl Pts',(18.1272,50.5293315887451,2.88308325260878));
#72860=CARTESIAN_POINT('Ctrl Pts',(18.3,50.3830830991268,2.98458385318518));
#72861=CARTESIAN_POINT('Ctrl Pts',(18.1272,50.3830830991268,2.98458385318518));
#72862=CARTESIAN_POINT('Ctrl Pts',(18.3,49.9890859663486,2.98458385318518));
#72863=CARTESIAN_POINT('Ctrl Pts',(18.1272,49.9890859663486,2.98458385318518));
#72864=CARTESIAN_POINT('Ctrl Pts',(18.3,50.5293315887451,2.88308325260878));
#72865=CARTESIAN_POINT('Ctrl Pts',(18.3,50.3830830991268,2.98458385318518));
#72866=CARTESIAN_POINT('Ctrl Pts',(18.3,49.9890859663486,2.98458385318518));
#72867=CARTESIAN_POINT('Ctrl Pts',(18.18,50.5293315887451,2.88308325260878));
#72868=CARTESIAN_POINT('Ctrl Pts',(18.18,50.3830830991268,2.98458385318518));
#72869=CARTESIAN_POINT('Ctrl Pts',(18.18,49.9890859663486,2.98458385318518));
#72870=CARTESIAN_POINT('Ctrl Pts',(18.3,49.1727148234844,2.66480210274458));
#72871=CARTESIAN_POINT('Ctrl Pts',(18.1272,49.1727148234844,2.66480210274458));
#72872=CARTESIAN_POINT('Ctrl Pts',(18.3,49.1727148234844,2.89618003219366));
#72873=CARTESIAN_POINT('Ctrl Pts',(18.1272,49.1727148234844,2.89618003219366));
#72874=CARTESIAN_POINT('Ctrl Pts',(18.3,49.3386085569858,3.02824008315802));
#72875=CARTESIAN_POINT('Ctrl Pts',(18.1272,49.3386085569858,3.02824008315802));
#72876=CARTESIAN_POINT('',(18.3,49.1727148234844,2.66480210274458));
#72877=CARTESIAN_POINT('',(18.3,49.3386085569858,3.02824008315802));
#72878=CARTESIAN_POINT('Ctrl Pts',(18.3,49.1727148234844,2.66480210274458));
#72879=CARTESIAN_POINT('Ctrl Pts',(18.3,49.1727148234844,2.89618003219366));
#72880=CARTESIAN_POINT('Ctrl Pts',(18.3,49.3386085569858,3.02824008315802));
#72881=CARTESIAN_POINT('',(18.18,49.1727148234844,2.66480210274458));
#72882=CARTESIAN_POINT('',(18.3,49.1727148234844,2.66480210274458));
#72883=CARTESIAN_POINT('',(18.18,49.3386085569858,3.02824008315802));
#72884=CARTESIAN_POINT('Ctrl Pts',(18.18,49.1727148234844,2.66480210274458));
#72885=CARTESIAN_POINT('Ctrl Pts',(18.18,49.1727148234844,2.89618003219366));
#72886=CARTESIAN_POINT('Ctrl Pts',(18.18,49.3386085569858,3.02824008315802));
#72887=CARTESIAN_POINT('',(18.3,49.3386085569858,3.02824008315802));
#72888=CARTESIAN_POINT('Ctrl Pts',(18.3,49.2671214282513,2.37394276112318));
#72889=CARTESIAN_POINT('Ctrl Pts',(18.1272,49.2671214282513,2.37394276112318));
#72890=CARTESIAN_POINT('Ctrl Pts',(18.3,49.1727148234844,2.489085970819));
#72891=CARTESIAN_POINT('Ctrl Pts',(18.1272,49.1727148234844,2.489085970819));
#72892=CARTESIAN_POINT('Ctrl Pts',(18.3,49.1727148234844,2.66480210274458));
#72893=CARTESIAN_POINT('Ctrl Pts',(18.1272,49.1727148234844,2.66480210274458));
#72894=CARTESIAN_POINT('',(18.3,49.2671214282513,2.37394276112318));
#72895=CARTESIAN_POINT('Ctrl Pts',(18.3,49.2671214282513,2.37394276112318));
#72896=CARTESIAN_POINT('Ctrl Pts',(18.3,49.1727148234844,2.489085970819));
#72897=CARTESIAN_POINT('Ctrl Pts',(18.3,49.1727148234844,2.66480210274458));
#72898=CARTESIAN_POINT('',(18.18,49.2671214282513,2.37394276112318));
#72899=CARTESIAN_POINT('',(18.3,49.2671214282513,2.37394276112318));
#72900=CARTESIAN_POINT('Ctrl Pts',(18.18,49.2671214282513,2.37394276112318));
#72901=CARTESIAN_POINT('Ctrl Pts',(18.18,49.1727148234844,2.489085970819));
#72902=CARTESIAN_POINT('Ctrl Pts',(18.18,49.1727148234844,2.66480210274458));
#72903=CARTESIAN_POINT('Ctrl Pts',(18.3,49.5345156133175,2.20095503181219));
#72904=CARTESIAN_POINT('Ctrl Pts',(18.1272,49.5345156133175,2.20095503181219));
#72905=CARTESIAN_POINT('Ctrl Pts',(18.3,49.3615280330181,2.25879940241575));
#72906=CARTESIAN_POINT('Ctrl Pts',(18.1272,49.3615280330181,2.25879940241575));
#72907=CARTESIAN_POINT('Ctrl Pts',(18.3,49.2671214282513,2.37394276112318));
#72908=CARTESIAN_POINT('Ctrl Pts',(18.1272,49.2671214282513,2.37394276112318));
#72909=CARTESIAN_POINT('',(18.3,49.5345156133175,2.20095503181219));
#72910=CARTESIAN_POINT('Ctrl Pts',(18.3,49.5345156133175,2.20095503181219));
#72911=CARTESIAN_POINT('Ctrl Pts',(18.3,49.3615280330181,2.25879940241575));
#72912=CARTESIAN_POINT('Ctrl Pts',(18.3,49.2671214282513,2.37394276112318));
#72913=CARTESIAN_POINT('',(18.18,49.5345156133175,2.20095503181219));
#72914=CARTESIAN_POINT('',(18.3,49.5345156133175,2.20095503181219));
#72915=CARTESIAN_POINT('Ctrl Pts',(18.18,49.5345156133175,2.20095503181219));
#72916=CARTESIAN_POINT('Ctrl Pts',(18.18,49.3615280330181,2.25879940241575));
#72917=CARTESIAN_POINT('Ctrl Pts',(18.18,49.2671214282513,2.37394276112318));
#72918=CARTESIAN_POINT('Ctrl Pts',(18.3,49.9890859663486,2.14311051219702));
#72919=CARTESIAN_POINT('Ctrl Pts',(18.1272,49.9890859663486,2.14311051219702));
#72920=CARTESIAN_POINT('Ctrl Pts',(18.3,49.7075034916401,2.14311051219702));
#72921=CARTESIAN_POINT('Ctrl Pts',(18.1272,49.7075034916401,2.14311051219702));
#72922=CARTESIAN_POINT('Ctrl Pts',(18.3,49.5345156133175,2.20095503181219));
#72923=CARTESIAN_POINT('Ctrl Pts',(18.1272,49.5345156133175,2.20095503181219));
#72924=CARTESIAN_POINT('',(18.3,49.9890859663486,2.14311051219702));
#72925=CARTESIAN_POINT('Ctrl Pts',(18.3,49.9890859663486,2.14311051219702));
#72926=CARTESIAN_POINT('Ctrl Pts',(18.3,49.7075034916401,2.14311051219702));
#72927=CARTESIAN_POINT('Ctrl Pts',(18.3,49.5345156133175,2.20095503181219));
#72928=CARTESIAN_POINT('',(18.18,49.9890859663486,2.14311051219702));
#72929=CARTESIAN_POINT('',(18.3,49.9890859663486,2.14311051219702));
#72930=CARTESIAN_POINT('Ctrl Pts',(18.18,49.9890859663486,2.14311051219702));
#72931=CARTESIAN_POINT('Ctrl Pts',(18.18,49.7075034916401,2.14311051219702));
#72932=CARTESIAN_POINT('Ctrl Pts',(18.18,49.5345156133175,2.20095503181219));
#72933=CARTESIAN_POINT('Ctrl Pts',(18.3,50.3672577679157,2.17912691682577));
#72934=CARTESIAN_POINT('Ctrl Pts',(18.1272,50.3672577679157,2.17912691682577));
#72935=CARTESIAN_POINT('Ctrl Pts',(18.3,50.2270122110844,2.14311051219702));
#72936=CARTESIAN_POINT('Ctrl Pts',(18.1272,50.2270122110844,2.14311051219702));
#72937=CARTESIAN_POINT('Ctrl Pts',(18.3,49.9890859663486,2.14311051219702));
#72938=CARTESIAN_POINT('Ctrl Pts',(18.1272,49.9890859663486,2.14311051219702));
#72939=CARTESIAN_POINT('',(18.3,50.3672577679157,2.17912691682577));
#72940=CARTESIAN_POINT('Ctrl Pts',(18.3,50.3672577679157,2.17912691682577));
#72941=CARTESIAN_POINT('Ctrl Pts',(18.3,50.2270122110844,2.14311051219702));
#72942=CARTESIAN_POINT('Ctrl Pts',(18.3,49.9890859663486,2.14311051219702));
#72943=CARTESIAN_POINT('',(18.18,50.3672577679157,2.17912691682577));
#72944=CARTESIAN_POINT('',(18.3,50.3672577679157,2.17912691682577));
#72945=CARTESIAN_POINT('Ctrl Pts',(18.18,50.3672577679157,2.17912691682577));
#72946=CARTESIAN_POINT('Ctrl Pts',(18.18,50.2270122110844,2.14311051219702));
#72947=CARTESIAN_POINT('Ctrl Pts',(18.18,49.9890859663486,2.14311051219702));
#72948=CARTESIAN_POINT('Ctrl Pts',(18.3,50.605184161663,2.2784447953105));
#72949=CARTESIAN_POINT('Ctrl Pts',(18.1272,50.605184161663,2.2784447953105));
#72950=CARTESIAN_POINT('Ctrl Pts',(18.3,50.5075034737587,2.21514317244291));
#72951=CARTESIAN_POINT('Ctrl Pts',(18.1272,50.5075034737587,2.21514317244291));
#72952=CARTESIAN_POINT('Ctrl Pts',(18.3,50.3672577679157,2.17912691682577));
#72953=CARTESIAN_POINT('Ctrl Pts',(18.1272,50.3672577679157,2.17912691682577));
#72954=CARTESIAN_POINT('',(18.3,50.605184161663,2.2784447953105));
#72955=CARTESIAN_POINT('Ctrl Pts',(18.3,50.605184161663,2.2784447953105));
#72956=CARTESIAN_POINT('Ctrl Pts',(18.3,50.5075034737587,2.21514317244291));
#72957=CARTESIAN_POINT('Ctrl Pts',(18.3,50.3672577679157,2.17912691682577));
#72958=CARTESIAN_POINT('',(18.18,50.605184161663,2.2784447953105));
#72959=CARTESIAN_POINT('',(18.3,50.605184161663,2.2784447953105));
#72960=CARTESIAN_POINT('Ctrl Pts',(18.18,50.605184161663,2.2784447953105));
#72961=CARTESIAN_POINT('Ctrl Pts',(18.18,50.5075034737587,2.21514317244291));
#72962=CARTESIAN_POINT('Ctrl Pts',(18.18,50.3672577679157,2.17912691682577));
#72963=CARTESIAN_POINT('Ctrl Pts',(18.3,50.7547067344189,2.43888142555952));
#72964=CARTESIAN_POINT('Ctrl Pts',(18.1272,50.7547067344189,2.43888142555952));
#72965=CARTESIAN_POINT('Ctrl Pts',(18.3,50.702864998579,2.34174626916647));
#72966=CARTESIAN_POINT('Ctrl Pts',(18.1272,50.702864998579,2.34174626916647));
#72967=CARTESIAN_POINT('Ctrl Pts',(18.3,50.605184161663,2.2784447953105));
#72968=CARTESIAN_POINT('Ctrl Pts',(18.1272,50.605184161663,2.2784447953105));
#72969=CARTESIAN_POINT('',(18.3,50.7547067344189,2.43888142555952));
#72970=CARTESIAN_POINT('Ctrl Pts',(18.3,50.7547067344189,2.43888142555952));
#72971=CARTESIAN_POINT('Ctrl Pts',(18.3,50.702864998579,2.34174626916647));
#72972=CARTESIAN_POINT('Ctrl Pts',(18.3,50.605184161663,2.2784447953105));
#72973=CARTESIAN_POINT('',(18.18,50.7547067344189,2.43888142555952));
#72974=CARTESIAN_POINT('',(18.3,50.7547067344189,2.43888142555952));
#72975=CARTESIAN_POINT('Ctrl Pts',(18.18,50.7547067344189,2.43888142555952));
#72976=CARTESIAN_POINT('Ctrl Pts',(18.18,50.702864998579,2.34174626916647));
#72977=CARTESIAN_POINT('Ctrl Pts',(18.18,50.605184161663,2.2784447953105));
#72978=CARTESIAN_POINT('Ctrl Pts',(18.3,50.8065484702587,2.66480210274458));
#72979=CARTESIAN_POINT('Ctrl Pts',(18.1272,50.8065484702587,2.66480210274458));
#72980=CARTESIAN_POINT('Ctrl Pts',(18.3,50.8065484702587,2.53601643294096));
#72981=CARTESIAN_POINT('Ctrl Pts',(18.1272,50.8065484702587,2.53601643294096));
#72982=CARTESIAN_POINT('Ctrl Pts',(18.3,50.7547067344189,2.43888142555952));
#72983=CARTESIAN_POINT('Ctrl Pts',(18.1272,50.7547067344189,2.43888142555952));
#72984=CARTESIAN_POINT('',(18.3,50.8065484702587,2.66480210274458));
#72985=CARTESIAN_POINT('Ctrl Pts',(18.3,50.8065484702587,2.66480210274458));
#72986=CARTESIAN_POINT('Ctrl Pts',(18.3,50.8065484702587,2.53601643294096));
#72987=CARTESIAN_POINT('Ctrl Pts',(18.3,50.7547067344189,2.43888142555952));
#72988=CARTESIAN_POINT('',(18.18,50.8065484702587,2.66480210274458));
#72989=CARTESIAN_POINT('',(18.3,50.8065484702587,2.66480210274458));
#72990=CARTESIAN_POINT('Ctrl Pts',(18.18,50.8065484702587,2.66480210274458));
#72991=CARTESIAN_POINT('Ctrl Pts',(18.18,50.8065484702587,2.53601643294096));
#72992=CARTESIAN_POINT('Ctrl Pts',(18.18,50.7547067344189,2.43888142555952));
#72993=CARTESIAN_POINT('Ctrl Pts',(18.3,50.7126876950264,2.95457023233175));
#72994=CARTESIAN_POINT('Ctrl Pts',(18.1272,50.7126876950264,2.95457023233175));
#72995=CARTESIAN_POINT('Ctrl Pts',(18.3,50.8065484702587,2.83942702263594));
#72996=CARTESIAN_POINT('Ctrl Pts',(18.1272,50.8065484702587,2.83942702263594));
#72997=CARTESIAN_POINT('Ctrl Pts',(18.3,50.8065484702587,2.66480210274458));
#72998=CARTESIAN_POINT('Ctrl Pts',(18.1272,50.8065484702587,2.66480210274458));
#72999=CARTESIAN_POINT('',(18.3,50.7126876950264,2.95457023233175));
#73000=CARTESIAN_POINT('Ctrl Pts',(18.3,50.7126876950264,2.95457023233175));
#73001=CARTESIAN_POINT('Ctrl Pts',(18.3,50.8065484702587,2.83942702263594));
#73002=CARTESIAN_POINT('Ctrl Pts',(18.3,50.8065484702587,2.66480210274458));
#73003=CARTESIAN_POINT('',(18.18,50.7126876950264,2.95457023233175));
#73004=CARTESIAN_POINT('',(18.3,50.7126876950264,2.95457023233175));
#73005=CARTESIAN_POINT('Ctrl Pts',(18.18,50.7126876950264,2.95457023233175));
#73006=CARTESIAN_POINT('Ctrl Pts',(18.18,50.8065484702587,2.83942702263594));
#73007=CARTESIAN_POINT('Ctrl Pts',(18.18,50.8065484702587,2.66480210274458));
#73008=CARTESIAN_POINT('Ctrl Pts',(18.3,50.4458390414715,3.12810364216566));
#73009=CARTESIAN_POINT('Ctrl Pts',(18.1272,50.4458390414715,3.12810364216566));
#73010=CARTESIAN_POINT('Ctrl Pts',(18.3,50.6188267707825,3.06971344202757));
#73011=CARTESIAN_POINT('Ctrl Pts',(18.1272,50.6188267707825,3.06971344202757));
#73012=CARTESIAN_POINT('Ctrl Pts',(18.3,50.7126876950264,2.95457023233175));
#73013=CARTESIAN_POINT('Ctrl Pts',(18.1272,50.7126876950264,2.95457023233175));
#73014=CARTESIAN_POINT('',(18.3,50.4458390414715,3.12810364216566));
#73015=CARTESIAN_POINT('Ctrl Pts',(18.3,50.4458390414715,3.12810364216566));
#73016=CARTESIAN_POINT('Ctrl Pts',(18.3,50.6188267707825,3.06971344202757));
#73017=CARTESIAN_POINT('Ctrl Pts',(18.3,50.7126876950264,2.95457023233175));
#73018=CARTESIAN_POINT('',(18.18,50.4458390414715,3.12810364216566));
#73019=CARTESIAN_POINT('',(18.3,50.4458390414715,3.12810364216566));
#73020=CARTESIAN_POINT('Ctrl Pts',(18.18,50.4458390414715,3.12810364216566));
#73021=CARTESIAN_POINT('Ctrl Pts',(18.18,50.6188267707825,3.06971344202757));
#73022=CARTESIAN_POINT('Ctrl Pts',(18.18,50.7126876950264,2.95457023233175));
#73023=CARTESIAN_POINT('Ctrl Pts',(18.3,49.9890859663486,3.18649384230375));
#73024=CARTESIAN_POINT('Ctrl Pts',(18.1272,49.9890859663486,3.18649384230375));
#73025=CARTESIAN_POINT('Ctrl Pts',(18.3,50.2728513121605,3.18649384230375));
#73026=CARTESIAN_POINT('Ctrl Pts',(18.1272,50.2728513121605,3.18649384230375));
#73027=CARTESIAN_POINT('Ctrl Pts',(18.3,50.4458390414715,3.12810364216566));
#73028=CARTESIAN_POINT('Ctrl Pts',(18.1272,50.4458390414715,3.12810364216566));
#73029=CARTESIAN_POINT('',(18.3,49.9890859663486,3.18649384230375));
#73030=CARTESIAN_POINT('Ctrl Pts',(18.3,49.9890859663486,3.18649384230375));
#73031=CARTESIAN_POINT('Ctrl Pts',(18.3,50.2728513121605,3.18649384230375));
#73032=CARTESIAN_POINT('Ctrl Pts',(18.3,50.4458390414715,3.12810364216566));
#73033=CARTESIAN_POINT('',(18.18,49.9890859663486,3.18649384230375));
#73034=CARTESIAN_POINT('',(18.3,49.9890859663486,3.18649384230375));
#73035=CARTESIAN_POINT('Ctrl Pts',(18.18,49.9890859663486,3.18649384230375));
#73036=CARTESIAN_POINT('Ctrl Pts',(18.18,50.2728513121605,3.18649384230375));
#73037=CARTESIAN_POINT('Ctrl Pts',(18.18,50.4458390414715,3.12810364216566));
#73038=CARTESIAN_POINT('Ctrl Pts',(18.3,49.3386085569858,3.02824008315802));
#73039=CARTESIAN_POINT('Ctrl Pts',(18.1272,49.3386085569858,3.02824008315802));
#73040=CARTESIAN_POINT('Ctrl Pts',(18.3,49.5383356750011,3.18649384230375));
#73041=CARTESIAN_POINT('Ctrl Pts',(18.1272,49.5383356750011,3.18649384230375));
#73042=CARTESIAN_POINT('Ctrl Pts',(18.3,49.9890859663486,3.18649384230375));
#73043=CARTESIAN_POINT('Ctrl Pts',(18.1272,49.9890859663486,3.18649384230375));
#73044=CARTESIAN_POINT('Ctrl Pts',(18.3,49.3386085569858,3.02824008315802));
#73045=CARTESIAN_POINT('Ctrl Pts',(18.3,49.5383356750011,3.18649384230375));
#73046=CARTESIAN_POINT('Ctrl Pts',(18.3,49.9890859663486,3.18649384230375));
#73047=CARTESIAN_POINT('Ctrl Pts',(18.18,49.3386085569858,3.02824008315802));
#73048=CARTESIAN_POINT('Ctrl Pts',(18.18,49.5383356750011,3.18649384230375));
#73049=CARTESIAN_POINT('Ctrl Pts',(18.18,49.9890859663486,3.18649384230375));
#73050=CARTESIAN_POINT('Origin',(18.18,49.9896316468716,3.29999995455146));
#73051=CARTESIAN_POINT('Ctrl Pts',(18.3,49.4952251255512,4.09890851974487));
#73052=CARTESIAN_POINT('Ctrl Pts',(18.1272,49.4952251255512,4.09890851974487));
#73053=CARTESIAN_POINT('Ctrl Pts',(18.3,49.4422920286655,4.14911313951015));
#73054=CARTESIAN_POINT('Ctrl Pts',(18.1272,49.4422920286655,4.14911313951015));
#73055=CARTESIAN_POINT('Ctrl Pts',(18.3,49.3888132512569,4.18185527473688));
#73056=CARTESIAN_POINT('Ctrl Pts',(18.1272,49.3888132512569,4.18185527473688));
#73057=CARTESIAN_POINT('',(18.3,49.4952251255512,4.09890851974487));
#73058=CARTESIAN_POINT('',(18.3,49.3888132512569,4.18185527473688));
#73059=CARTESIAN_POINT('Ctrl Pts',(18.3,49.4952251255512,4.09890851974487));
#73060=CARTESIAN_POINT('Ctrl Pts',(18.3,49.4422920286655,4.14911313951015));
#73061=CARTESIAN_POINT('Ctrl Pts',(18.3,49.3888132512569,4.18185527473688));
#73062=CARTESIAN_POINT('',(18.18,49.4952251255512,4.09890851974487));
#73063=CARTESIAN_POINT('',(18.3,49.4952251255512,4.09890851974487));
#73064=CARTESIAN_POINT('',(18.18,49.3888132512569,4.18185527473688));
#73065=CARTESIAN_POINT('Ctrl Pts',(18.18,49.4952251255512,4.09890851974487));
#73066=CARTESIAN_POINT('Ctrl Pts',(18.18,49.4422920286655,4.14911313951015));
#73067=CARTESIAN_POINT('Ctrl Pts',(18.18,49.3888132512569,4.18185527473688));
#73068=CARTESIAN_POINT('',(18.3,49.3888132512569,4.18185527473688));
#73069=CARTESIAN_POINT('Ctrl Pts',(18.3,49.6965892851353,3.87189629524946));
#73070=CARTESIAN_POINT('Ctrl Pts',(18.1272,49.6965892851353,3.87189629524946));
#73071=CARTESIAN_POINT('Ctrl Pts',(18.3,49.5481582224369,4.04870386272669));
#73072=CARTESIAN_POINT('Ctrl Pts',(18.1272,49.5481582224369,4.04870386272669));
#73073=CARTESIAN_POINT('Ctrl Pts',(18.3,49.4952251255512,4.09890851974487));
#73074=CARTESIAN_POINT('Ctrl Pts',(18.1272,49.4952251255512,4.09890851974487));
#73075=CARTESIAN_POINT('',(18.3,49.6965892851353,3.87189629524946));
#73076=CARTESIAN_POINT('Ctrl Pts',(18.3,49.6965892851353,3.87189629524946));
#73077=CARTESIAN_POINT('Ctrl Pts',(18.3,49.5481582224369,4.04870386272669));
#73078=CARTESIAN_POINT('Ctrl Pts',(18.3,49.4952251255512,4.09890851974487));
#73079=CARTESIAN_POINT('',(18.18,49.6965892851353,3.87189629524946));
#73080=CARTESIAN_POINT('',(18.3,49.6965892851353,3.87189629524946));
#73081=CARTESIAN_POINT('Ctrl Pts',(18.18,49.6965892851353,3.87189629524946));
#73082=CARTESIAN_POINT('Ctrl Pts',(18.18,49.5481582224369,4.04870386272669));
#73083=CARTESIAN_POINT('Ctrl Pts',(18.18,49.4952251255512,4.09890851974487));
#73084=CARTESIAN_POINT('Ctrl Pts',(18.3,49.978172057867,3.5690313860774));
#73085=CARTESIAN_POINT('Ctrl Pts',(18.1272,49.978172057867,3.5690313860774));
#73086=CARTESIAN_POINT('Ctrl Pts',(18.3,49.8755799472332,3.66016360968351));
#73087=CARTESIAN_POINT('Ctrl Pts',(18.1272,49.8755799472332,3.66016360968351));
#73088=CARTESIAN_POINT('Ctrl Pts',(18.3,49.6965892851353,3.87189629524946));
#73089=CARTESIAN_POINT('Ctrl Pts',(18.1272,49.6965892851353,3.87189629524946));
#73090=CARTESIAN_POINT('',(18.3,49.978172057867,3.5690313860774));
#73091=CARTESIAN_POINT('Ctrl Pts',(18.3,49.978172057867,3.5690313860774));
#73092=CARTESIAN_POINT('Ctrl Pts',(18.3,49.8755799472332,3.66016360968351));
#73093=CARTESIAN_POINT('Ctrl Pts',(18.3,49.6965892851353,3.87189629524946));
#73094=CARTESIAN_POINT('',(18.18,49.978172057867,3.5690313860774));
#73095=CARTESIAN_POINT('',(18.3,49.978172057867,3.5690313860774));
#73096=CARTESIAN_POINT('Ctrl Pts',(18.18,49.978172057867,3.5690313860774));
#73097=CARTESIAN_POINT('Ctrl Pts',(18.18,49.8755799472332,3.66016360968351));
#73098=CARTESIAN_POINT('Ctrl Pts',(18.18,49.6965892851353,3.87189629524946));
#73099=CARTESIAN_POINT('Ctrl Pts',(18.3,50.1735334336758,3.4386083766818));
#73100=CARTESIAN_POINT('Ctrl Pts',(18.1272,50.1735334336758,3.4386083766818));
#73101=CARTESIAN_POINT('Ctrl Pts',(18.3,50.0807640194893,3.47789901345968));
#73102=CARTESIAN_POINT('Ctrl Pts',(18.1272,50.0807640194893,3.47789901345968));
#73103=CARTESIAN_POINT('Ctrl Pts',(18.3,49.978172057867,3.5690313860774));
#73104=CARTESIAN_POINT('Ctrl Pts',(18.1272,49.978172057867,3.5690313860774));
#73105=CARTESIAN_POINT('',(18.3,50.1735334336758,3.4386083766818));
#73106=CARTESIAN_POINT('Ctrl Pts',(18.3,50.1735334336758,3.4386083766818));
#73107=CARTESIAN_POINT('Ctrl Pts',(18.3,50.0807640194893,3.47789901345968));
#73108=CARTESIAN_POINT('Ctrl Pts',(18.3,49.978172057867,3.5690313860774));
#73109=CARTESIAN_POINT('',(18.18,50.1735334336758,3.4386083766818));
#73110=CARTESIAN_POINT('',(18.3,50.1735334336758,3.4386083766818));
#73111=CARTESIAN_POINT('Ctrl Pts',(18.18,50.1735334336758,3.4386083766818));
#73112=CARTESIAN_POINT('Ctrl Pts',(18.18,50.0807640194893,3.47789901345968));
#73113=CARTESIAN_POINT('Ctrl Pts',(18.18,49.978172057867,3.5690313860774));
#73114=CARTESIAN_POINT('Ctrl Pts',(18.3,50.3623466432094,3.39931788891554));
#73115=CARTESIAN_POINT('Ctrl Pts',(18.1272,50.3623466432094,3.39931788891554));
#73116=CARTESIAN_POINT('Ctrl Pts',(18.3,50.2663029968738,3.39931788891554));
#73117=CARTESIAN_POINT('Ctrl Pts',(18.1272,50.2663029968738,3.39931788891554));
#73118=CARTESIAN_POINT('Ctrl Pts',(18.3,50.1735334336758,3.4386083766818));
#73119=CARTESIAN_POINT('Ctrl Pts',(18.1272,50.1735334336758,3.4386083766818));
#73120=CARTESIAN_POINT('',(18.3,50.3623466432094,3.39931788891554));
#73121=CARTESIAN_POINT('Ctrl Pts',(18.3,50.3623466432094,3.39931788891554));
#73122=CARTESIAN_POINT('Ctrl Pts',(18.3,50.2663029968738,3.39931788891554));
#73123=CARTESIAN_POINT('Ctrl Pts',(18.3,50.1735334336758,3.4386083766818));
#73124=CARTESIAN_POINT('',(18.18,50.3623466432094,3.39931788891554));
#73125=CARTESIAN_POINT('',(18.3,50.3623466432094,3.39931788891554));
#73126=CARTESIAN_POINT('Ctrl Pts',(18.18,50.3623466432094,3.39931788891554));
#73127=CARTESIAN_POINT('Ctrl Pts',(18.18,50.2663029968738,3.39931788891554));
#73128=CARTESIAN_POINT('Ctrl Pts',(18.18,50.1735334336758,3.4386083766818));
#73129=CARTESIAN_POINT('Ctrl Pts',(18.3,50.6788541615009,3.53356066197157));
#73130=CARTESIAN_POINT('Ctrl Pts',(18.1272,50.6788541615009,3.53356066197157));
#73131=CARTESIAN_POINT('Ctrl Pts',(18.3,50.5511597037315,3.39931788891554));
#73132=CARTESIAN_POINT('Ctrl Pts',(18.1272,50.5511597037315,3.39931788891554));
#73133=CARTESIAN_POINT('Ctrl Pts',(18.3,50.3623466432094,3.39931788891554));
#73134=CARTESIAN_POINT('Ctrl Pts',(18.1272,50.3623466432094,3.39931788891554));
#73135=CARTESIAN_POINT('',(18.3,50.6788541615009,3.53356066197157));
#73136=CARTESIAN_POINT('Ctrl Pts',(18.3,50.6788541615009,3.53356066197157));
#73137=CARTESIAN_POINT('Ctrl Pts',(18.3,50.5511597037315,3.39931788891554));
#73138=CARTESIAN_POINT('Ctrl Pts',(18.3,50.3623466432094,3.39931788891554));
#73139=CARTESIAN_POINT('',(18.18,50.6788541615009,3.53356066197157));
#73140=CARTESIAN_POINT('',(18.3,50.6788541615009,3.53356066197157));
#73141=CARTESIAN_POINT('Ctrl Pts',(18.18,50.6788541615009,3.53356066197157));
#73142=CARTESIAN_POINT('Ctrl Pts',(18.18,50.5511597037315,3.39931788891554));
#73143=CARTESIAN_POINT('Ctrl Pts',(18.18,50.3623466432094,3.39931788891554));
#73144=CARTESIAN_POINT('Ctrl Pts',(18.3,50.8065484702587,3.89809000343084));
#73145=CARTESIAN_POINT('Ctrl Pts',(18.1272,50.8065484702587,3.89809000343084));
#73146=CARTESIAN_POINT('Ctrl Pts',(18.3,50.8065484702587,3.6678034350276));
#73147=CARTESIAN_POINT('Ctrl Pts',(18.1272,50.8065484702587,3.6678034350276));
#73148=CARTESIAN_POINT('Ctrl Pts',(18.3,50.6788541615009,3.53356066197157));
#73149=CARTESIAN_POINT('Ctrl Pts',(18.1272,50.6788541615009,3.53356066197157));
#73150=CARTESIAN_POINT('',(18.3,50.8065484702587,3.89809000343084));
#73151=CARTESIAN_POINT('Ctrl Pts',(18.3,50.8065484702587,3.89809000343084));
#73152=CARTESIAN_POINT('Ctrl Pts',(18.3,50.8065484702587,3.6678034350276));
#73153=CARTESIAN_POINT('Ctrl Pts',(18.3,50.6788541615009,3.53356066197157));
#73154=CARTESIAN_POINT('',(18.18,50.8065484702587,3.89809000343084));
#73155=CARTESIAN_POINT('',(18.3,50.8065484702587,3.89809000343084));
#73156=CARTESIAN_POINT('Ctrl Pts',(18.18,50.8065484702587,3.89809000343084));
#73157=CARTESIAN_POINT('Ctrl Pts',(18.18,50.8065484702587,3.6678034350276));
#73158=CARTESIAN_POINT('Ctrl Pts',(18.18,50.6788541615009,3.53356066197157));
#73159=CARTESIAN_POINT('Ctrl Pts',(18.3,50.6881310284138,4.26152787208557));
#73160=CARTESIAN_POINT('Ctrl Pts',(18.1272,50.6881310284138,4.26152787208557));
#73161=CARTESIAN_POINT('Ctrl Pts',(18.3,50.8065484702587,4.12619362622499));
#73162=CARTESIAN_POINT('Ctrl Pts',(18.1272,50.8065484702587,4.12619362622499));
#73163=CARTESIAN_POINT('Ctrl Pts',(18.3,50.8065484702587,3.89809000343084));
#73164=CARTESIAN_POINT('Ctrl Pts',(18.1272,50.8065484702587,3.89809000343084));
#73165=CARTESIAN_POINT('',(18.3,50.6881310284138,4.26152787208557));
#73166=CARTESIAN_POINT('Ctrl Pts',(18.3,50.6881310284138,4.26152787208557));
#73167=CARTESIAN_POINT('Ctrl Pts',(18.3,50.8065484702587,4.12619362622499));
#73168=CARTESIAN_POINT('Ctrl Pts',(18.3,50.8065484702587,3.89809000343084));
#73169=CARTESIAN_POINT('',(18.18,50.6881310284138,4.26152787208557));
#73170=CARTESIAN_POINT('',(18.3,50.6881310284138,4.26152787208557));
#73171=CARTESIAN_POINT('Ctrl Pts',(18.18,50.6881310284138,4.26152787208557));
#73172=CARTESIAN_POINT('Ctrl Pts',(18.18,50.8065484702587,4.12619362622499));
#73173=CARTESIAN_POINT('Ctrl Pts',(18.18,50.8065484702587,3.89809000343084));
#73174=CARTESIAN_POINT('Ctrl Pts',(18.3,50.3437926113605,4.41759881600738));
#73175=CARTESIAN_POINT('Ctrl Pts',(18.1272,50.3437926113605,4.41759881600738));
#73176=CARTESIAN_POINT('Ctrl Pts',(18.3,50.5697135865688,4.39686211794615));
#73177=CARTESIAN_POINT('Ctrl Pts',(18.1272,50.5697135865688,4.39686211794615));
#73178=CARTESIAN_POINT('Ctrl Pts',(18.3,50.6881310284138,4.26152787208557));
#73179=CARTESIAN_POINT('Ctrl Pts',(18.1272,50.6881310284138,4.26152787208557));
#73180=CARTESIAN_POINT('',(18.3,50.3437926113605,4.41759881600738));
#73181=CARTESIAN_POINT('Ctrl Pts',(18.3,50.3437926113605,4.41759881600738));
#73182=CARTESIAN_POINT('Ctrl Pts',(18.3,50.5697135865688,4.39686211794615));
#73183=CARTESIAN_POINT('Ctrl Pts',(18.3,50.6881310284138,4.26152787208557));
#73184=CARTESIAN_POINT('',(18.18,50.3437926113605,4.41759881600738));
#73185=CARTESIAN_POINT('',(18.3,50.3437926113605,4.41759881600738));
#73186=CARTESIAN_POINT('Ctrl Pts',(18.18,50.3437926113605,4.41759881600738));
#73187=CARTESIAN_POINT('Ctrl Pts',(18.18,50.5697135865688,4.39686211794615));
#73188=CARTESIAN_POINT('Ctrl Pts',(18.18,50.6881310284138,4.26152787208557));
#73189=CARTESIAN_POINT('Origin',(18.3,50.3230560064316,4.21568888276815));
#73190=CARTESIAN_POINT('',(18.3,50.3230560064316,4.21568888276815));
#73191=CARTESIAN_POINT('',(18.3,50.4910090704177,5.85102851782062));
#73192=CARTESIAN_POINT('',(18.18,50.3230560064316,4.21568888276815));
#73193=CARTESIAN_POINT('',(18.3,50.3230560064316,4.21568888276815));
#73194=CARTESIAN_POINT('',(18.18,50.3230560064316,4.21568888276815));
#73195=CARTESIAN_POINT('Ctrl Pts',(18.3,50.5587995290756,4.12946785837412));
#73196=CARTESIAN_POINT('Ctrl Pts',(18.1272,50.5587995290756,4.12946785837412));
#73197=CARTESIAN_POINT('Ctrl Pts',(18.3,50.4736699402332,4.21459744721651));
#73198=CARTESIAN_POINT('Ctrl Pts',(18.1272,50.4736699402332,4.21459744721651));
#73199=CARTESIAN_POINT('Ctrl Pts',(18.3,50.3230560064316,4.21568888276815));
#73200=CARTESIAN_POINT('Ctrl Pts',(18.1272,50.3230560064316,4.21568888276815));
#73201=CARTESIAN_POINT('',(18.3,50.5587995290756,4.12946785837412));
#73202=CARTESIAN_POINT('Ctrl Pts',(18.3,50.5587995290756,4.12946785837412));
#73203=CARTESIAN_POINT('Ctrl Pts',(18.3,50.4736699402332,4.21459744721651));
#73204=CARTESIAN_POINT('Ctrl Pts',(18.3,50.3230560064316,4.21568888276815));
#73205=CARTESIAN_POINT('',(18.18,50.5587995290756,4.12946785837412));
#73206=CARTESIAN_POINT('',(18.3,50.5587995290756,4.12946785837412));
#73207=CARTESIAN_POINT('Ctrl Pts',(18.18,50.5587995290756,4.12946785837412));
#73208=CARTESIAN_POINT('Ctrl Pts',(18.18,50.4736699402332,4.21459744721651));
#73209=CARTESIAN_POINT('Ctrl Pts',(18.18,50.3230560064316,4.21568888276815));
#73210=CARTESIAN_POINT('Ctrl Pts',(18.3,50.643929117918,3.9024555966258));
#73211=CARTESIAN_POINT('Ctrl Pts',(18.1272,50.643929117918,3.9024555966258));
#73212=CARTESIAN_POINT('Ctrl Pts',(18.3,50.643929117918,4.04433826953173));
#73213=CARTESIAN_POINT('Ctrl Pts',(18.1272,50.643929117918,4.04433826953173));
#73214=CARTESIAN_POINT('Ctrl Pts',(18.3,50.5587995290756,4.12946785837412));
#73215=CARTESIAN_POINT('Ctrl Pts',(18.1272,50.5587995290756,4.12946785837412));
#73216=CARTESIAN_POINT('',(18.3,50.643929117918,3.9024555966258));
#73217=CARTESIAN_POINT('Ctrl Pts',(18.3,50.643929117918,3.9024555966258));
#73218=CARTESIAN_POINT('Ctrl Pts',(18.3,50.643929117918,4.04433826953173));
#73219=CARTESIAN_POINT('Ctrl Pts',(18.3,50.5587995290756,4.12946785837412));
#73220=CARTESIAN_POINT('',(18.18,50.643929117918,3.9024555966258));
#73221=CARTESIAN_POINT('',(18.3,50.643929117918,3.9024555966258));
#73222=CARTESIAN_POINT('Ctrl Pts',(18.18,50.643929117918,3.9024555966258));
#73223=CARTESIAN_POINT('Ctrl Pts',(18.18,50.643929117918,4.04433826953173));
#73224=CARTESIAN_POINT('Ctrl Pts',(18.18,50.5587995290756,4.12946785837412));
#73225=CARTESIAN_POINT('Ctrl Pts',(18.3,50.5637108027935,3.68472027629614));
#73226=CARTESIAN_POINT('Ctrl Pts',(18.1272,50.5637108027935,3.68472027629614));
#73227=CARTESIAN_POINT('Ctrl Pts',(18.3,50.643929117918,3.76821282356977));
#73228=CARTESIAN_POINT('Ctrl Pts',(18.1272,50.643929117918,3.76821282356977));
#73229=CARTESIAN_POINT('Ctrl Pts',(18.3,50.643929117918,3.9024555966258));
#73230=CARTESIAN_POINT('Ctrl Pts',(18.1272,50.643929117918,3.9024555966258));
#73231=CARTESIAN_POINT('',(18.3,50.5637108027935,3.68472027629614));
#73232=CARTESIAN_POINT('Ctrl Pts',(18.3,50.5637108027935,3.68472027629614));
#73233=CARTESIAN_POINT('Ctrl Pts',(18.3,50.643929117918,3.76821282356977));
#73234=CARTESIAN_POINT('Ctrl Pts',(18.3,50.643929117918,3.9024555966258));
#73235=CARTESIAN_POINT('',(18.18,50.5637108027935,3.68472027629614));
#73236=CARTESIAN_POINT('',(18.3,50.5637108027935,3.68472027629614));
#73237=CARTESIAN_POINT('Ctrl Pts',(18.18,50.5637108027935,3.68472027629614));
#73238=CARTESIAN_POINT('Ctrl Pts',(18.18,50.643929117918,3.76821282356977));
#73239=CARTESIAN_POINT('Ctrl Pts',(18.18,50.643929117918,3.9024555966258));
#73240=CARTESIAN_POINT('Ctrl Pts',(18.3,50.3667122364044,3.6012277290225));
#73241=CARTESIAN_POINT('Ctrl Pts',(18.1272,50.3667122364044,3.6012277290225));
#73242=CARTESIAN_POINT('Ctrl Pts',(18.3,50.4834926366806,3.6012277290225));
#73243=CARTESIAN_POINT('Ctrl Pts',(18.1272,50.4834926366806,3.6012277290225));
#73244=CARTESIAN_POINT('Ctrl Pts',(18.3,50.5637108027935,3.68472027629614));
#73245=CARTESIAN_POINT('Ctrl Pts',(18.1272,50.5637108027935,3.68472027629614));
#73246=CARTESIAN_POINT('',(18.3,50.3667122364044,3.6012277290225));
#73247=CARTESIAN_POINT('Ctrl Pts',(18.3,50.3667122364044,3.6012277290225));
#73248=CARTESIAN_POINT('Ctrl Pts',(18.3,50.4834926366806,3.6012277290225));
#73249=CARTESIAN_POINT('Ctrl Pts',(18.3,50.5637108027935,3.68472027629614));
#73250=CARTESIAN_POINT('',(18.18,50.3667122364044,3.6012277290225));
#73251=CARTESIAN_POINT('',(18.3,50.3667122364044,3.6012277290225));
#73252=CARTESIAN_POINT('Ctrl Pts',(18.18,50.3667122364044,3.6012277290225));
#73253=CARTESIAN_POINT('Ctrl Pts',(18.18,50.4834926366806,3.6012277290225));
#73254=CARTESIAN_POINT('Ctrl Pts',(18.18,50.5637108027935,3.68472027629614));
#73255=CARTESIAN_POINT('Ctrl Pts',(18.3,50.1304228842258,3.69290578216314));
#73256=CARTESIAN_POINT('Ctrl Pts',(18.1272,50.1304228842258,3.69290578216314));
#73257=CARTESIAN_POINT('Ctrl Pts',(18.3,50.255388790369,3.6012277290225));
#73258=CARTESIAN_POINT('Ctrl Pts',(18.1272,50.255388790369,3.6012277290225));
#73259=CARTESIAN_POINT('Ctrl Pts',(18.3,50.3667122364044,3.6012277290225));
#73260=CARTESIAN_POINT('Ctrl Pts',(18.1272,50.3667122364044,3.6012277290225));
#73261=CARTESIAN_POINT('',(18.3,50.1304228842258,3.69290578216314));
#73262=CARTESIAN_POINT('Ctrl Pts',(18.3,50.1304228842258,3.69290578216314));
#73263=CARTESIAN_POINT('Ctrl Pts',(18.3,50.255388790369,3.6012277290225));
#73264=CARTESIAN_POINT('Ctrl Pts',(18.3,50.3667122364044,3.6012277290225));
#73265=CARTESIAN_POINT('',(18.18,50.1304228842258,3.69290578216314));
#73266=CARTESIAN_POINT('',(18.3,50.1304228842258,3.69290578216314));
#73267=CARTESIAN_POINT('Ctrl Pts',(18.18,50.1304228842258,3.69290578216314));
#73268=CARTESIAN_POINT('Ctrl Pts',(18.18,50.255388790369,3.6012277290225));
#73269=CARTESIAN_POINT('Ctrl Pts',(18.18,50.3667122364044,3.6012277290225));
#73270=CARTESIAN_POINT('Ctrl Pts',(18.3,49.791541570425,4.04542966783047));
#73271=CARTESIAN_POINT('Ctrl Pts',(18.1272,49.791541570425,4.04542966783047));
#73272=CARTESIAN_POINT('Ctrl Pts',(18.3,50.0054569780826,3.78458383530378));
#73273=CARTESIAN_POINT('Ctrl Pts',(18.1272,50.0054569780826,3.78458383530378));
#73274=CARTESIAN_POINT('Ctrl Pts',(18.3,50.1304228842258,3.69290578216314));
#73275=CARTESIAN_POINT('Ctrl Pts',(18.1272,50.1304228842258,3.69290578216314));
#73276=CARTESIAN_POINT('',(18.3,49.791541570425,4.04542966783047));
#73277=CARTESIAN_POINT('Ctrl Pts',(18.3,49.791541570425,4.04542966783047));
#73278=CARTESIAN_POINT('Ctrl Pts',(18.3,50.0054569780826,3.78458383530378));
#73279=CARTESIAN_POINT('Ctrl Pts',(18.3,50.1304228842258,3.69290578216314));
#73280=CARTESIAN_POINT('',(18.18,49.791541570425,4.04542966783047));
#73281=CARTESIAN_POINT('',(18.3,49.791541570425,4.04542966783047));
#73282=CARTESIAN_POINT('Ctrl Pts',(18.18,49.791541570425,4.04542966783047));
#73283=CARTESIAN_POINT('Ctrl Pts',(18.18,50.0054569780826,3.78458383530378));
#73284=CARTESIAN_POINT('Ctrl Pts',(18.18,50.1304228842258,3.69290578216314));
#73285=CARTESIAN_POINT('Ctrl Pts',(18.3,49.5492495834827,4.30245558768511));
#73286=CARTESIAN_POINT('Ctrl Pts',(18.1272,49.5492495834827,4.30245558768511));
#73287=CARTESIAN_POINT('Ctrl Pts',(18.3,49.6540247142315,4.21350604891777));
#73288=CARTESIAN_POINT('Ctrl Pts',(18.1272,49.6540247142315,4.21350604891777));
#73289=CARTESIAN_POINT('Ctrl Pts',(18.3,49.791541570425,4.04542966783047));
#73290=CARTESIAN_POINT('Ctrl Pts',(18.1272,49.791541570425,4.04542966783047));
#73291=CARTESIAN_POINT('',(18.3,49.5492495834827,4.30245558768511));
#73292=CARTESIAN_POINT('Ctrl Pts',(18.3,49.5492495834827,4.30245558768511));
#73293=CARTESIAN_POINT('Ctrl Pts',(18.3,49.6540247142315,4.21350604891777));
#73294=CARTESIAN_POINT('Ctrl Pts',(18.3,49.791541570425,4.04542966783047));
#73295=CARTESIAN_POINT('',(18.18,49.5492495834827,4.30245558768511));
#73296=CARTESIAN_POINT('',(18.3,49.5492495834827,4.30245558768511));
#73297=CARTESIAN_POINT('Ctrl Pts',(18.18,49.5492495834827,4.30245558768511));
#73298=CARTESIAN_POINT('Ctrl Pts',(18.18,49.6540247142315,4.21350604891777));
#73299=CARTESIAN_POINT('Ctrl Pts',(18.18,49.791541570425,4.04542966783047));
#73300=CARTESIAN_POINT('Ctrl Pts',(18.3,49.3364258348942,4.43178708702326));
#73301=CARTESIAN_POINT('Ctrl Pts',(18.1272,49.3364258348942,4.43178708702326));
#73302=CARTESIAN_POINT('Ctrl Pts',(18.3,49.4444747507572,4.39140508919954));
#73303=CARTESIAN_POINT('Ctrl Pts',(18.1272,49.4444747507572,4.39140508919954));
#73304=CARTESIAN_POINT('Ctrl Pts',(18.3,49.5492495834827,4.30245558768511));
#73305=CARTESIAN_POINT('Ctrl Pts',(18.1272,49.5492495834827,4.30245558768511));
#73306=CARTESIAN_POINT('',(18.3,49.3364258348942,4.43178708702326));
#73307=CARTESIAN_POINT('Ctrl Pts',(18.3,49.3364258348942,4.43178708702326));
#73308=CARTESIAN_POINT('Ctrl Pts',(18.3,49.4444747507572,4.39140508919954));
#73309=CARTESIAN_POINT('Ctrl Pts',(18.3,49.5492495834827,4.30245558768511));
#73310=CARTESIAN_POINT('',(18.18,49.3364258348942,4.43178708702326));
#73311=CARTESIAN_POINT('',(18.3,49.3364258348942,4.43178708702326));
#73312=CARTESIAN_POINT('Ctrl Pts',(18.18,49.3364258348942,4.43178708702326));
#73313=CARTESIAN_POINT('Ctrl Pts',(18.18,49.4444747507572,4.39140508919954));
#73314=CARTESIAN_POINT('Ctrl Pts',(18.18,49.5492495834827,4.30245558768511));
#73315=CARTESIAN_POINT('Ctrl Pts',(18.3,49.2000000417232,4.45470658168197));
#73316=CARTESIAN_POINT('Ctrl Pts',(18.1272,49.2000000417232,4.45470658168197));
#73317=CARTESIAN_POINT('Ctrl Pts',(18.3,49.2709414899349,4.4568893969059));
#73318=CARTESIAN_POINT('Ctrl Pts',(18.1272,49.2709414899349,4.4568893969059));
#73319=CARTESIAN_POINT('Ctrl Pts',(18.3,49.3364258348942,4.43178708702326));
#73320=CARTESIAN_POINT('Ctrl Pts',(18.1272,49.3364258348942,4.43178708702326));
#73321=CARTESIAN_POINT('',(18.3,49.2000000417232,4.45470658168197));
#73322=CARTESIAN_POINT('Ctrl Pts',(18.3,49.2000000417232,4.45470658168197));
#73323=CARTESIAN_POINT('Ctrl Pts',(18.3,49.2709414899349,4.4568893969059));
#73324=CARTESIAN_POINT('Ctrl Pts',(18.3,49.3364258348942,4.43178708702326));
#73325=CARTESIAN_POINT('',(18.18,49.2000000417232,4.45470658168197));
#73326=CARTESIAN_POINT('',(18.3,49.2000000417232,4.45470658168197));
#73327=CARTESIAN_POINT('Ctrl Pts',(18.18,49.2000000417232,4.45470658168197));
#73328=CARTESIAN_POINT('Ctrl Pts',(18.18,49.2709414899349,4.4568893969059));
#73329=CARTESIAN_POINT('Ctrl Pts',(18.18,49.3364258348942,4.43178708702326));
#73330=CARTESIAN_POINT('Origin',(18.3,49.2000000417232,3.39713501781225));
#73331=CARTESIAN_POINT('',(18.3,49.2000000417232,3.39713501781225));
#73332=CARTESIAN_POINT('',(18.3,49.2000000417232,4.44856750890613));
#73333=CARTESIAN_POINT('',(18.18,49.2000000417232,3.39713501781225));
#73334=CARTESIAN_POINT('',(18.3,49.2000000417232,3.39713501781225));
#73335=CARTESIAN_POINT('',(18.18,49.2000000417232,3.39713501781225));
#73336=CARTESIAN_POINT('Origin',(18.3,49.3888132512569,3.39713501781225));
#73337=CARTESIAN_POINT('',(18.3,49.3888132512569,3.39713501781225));
#73338=CARTESIAN_POINT('',(18.3,59.6944066256285,3.39713501781225));
#73339=CARTESIAN_POINT('',(18.18,49.3888132512569,3.39713501781225));
#73340=CARTESIAN_POINT('',(18.3,49.3888132512569,3.39713501781225));
#73341=CARTESIAN_POINT('',(18.18,49.3888132512569,3.39713501781225));
#73342=CARTESIAN_POINT('Origin',(18.3,49.3888132512569,4.18185527473688));
#73343=CARTESIAN_POINT('',(18.3,49.3888132512569,4.84092763736844));
#73344=CARTESIAN_POINT('',(18.18,49.3888132512569,4.18185527473688));
#73345=CARTESIAN_POINT('Origin',(18.18,49.9896316468716,3.29999995455146));
#73346=CARTESIAN_POINT('Origin',(18.3,70.,5.5));
#73347=CARTESIAN_POINT('Ctrl Pts',(18.3,40.643929117918,2.68117321692407));
#73348=CARTESIAN_POINT('Ctrl Pts',(18.1272,40.643929117918,2.68117321692407));
#73349=CARTESIAN_POINT('Ctrl Pts',(18.3,40.643929117918,2.81650750003755));
#73350=CARTESIAN_POINT('Ctrl Pts',(18.1272,40.643929117918,2.81650750003755));
#73351=CARTESIAN_POINT('Ctrl Pts',(18.3,40.5293315887451,2.89727149568498));
#73352=CARTESIAN_POINT('Ctrl Pts',(18.1272,40.5293315887451,2.89727149568498));
#73353=CARTESIAN_POINT('',(18.3,40.643929117918,2.68117321692407));
#73354=CARTESIAN_POINT('',(18.3,40.5293315887451,2.89727149568498));
#73355=CARTESIAN_POINT('Ctrl Pts',(18.3,40.643929117918,2.68117321692407));
#73356=CARTESIAN_POINT('Ctrl Pts',(18.3,40.643929117918,2.81650750003755));
#73357=CARTESIAN_POINT('Ctrl Pts',(18.3,40.5293315887451,2.89727149568498));
#73358=CARTESIAN_POINT('',(18.18,40.643929117918,2.68117321692407));
#73359=CARTESIAN_POINT('',(18.3,40.643929117918,2.68117321692407));
#73360=CARTESIAN_POINT('',(18.18,40.5293315887451,2.89727149568498));
#73361=CARTESIAN_POINT('Ctrl Pts',(18.18,40.643929117918,2.68117321692407));
#73362=CARTESIAN_POINT('Ctrl Pts',(18.18,40.643929117918,2.81650750003755));
#73363=CARTESIAN_POINT('Ctrl Pts',(18.18,40.5293315887451,2.89727149568498));
#73364=CARTESIAN_POINT('',(18.3,40.5293315887451,2.89727149568498));
#73365=CARTESIAN_POINT('Ctrl Pts',(18.3,40.5140519380569,2.45143247805536));
#73366=CARTESIAN_POINT('Ctrl Pts',(18.1272,40.5140519380569,2.45143247805536));
#73367=CARTESIAN_POINT('Ctrl Pts',(18.3,40.643929117918,2.54365621171892));
#73368=CARTESIAN_POINT('Ctrl Pts',(18.1272,40.643929117918,2.54365621171892));
#73369=CARTESIAN_POINT('Ctrl Pts',(18.3,40.643929117918,2.68117321692407));
#73370=CARTESIAN_POINT('Ctrl Pts',(18.1272,40.643929117918,2.68117321692407));
#73371=CARTESIAN_POINT('',(18.3,40.5140519380569,2.45143247805536));
#73372=CARTESIAN_POINT('Ctrl Pts',(18.3,40.5140519380569,2.45143247805536));
#73373=CARTESIAN_POINT('Ctrl Pts',(18.3,40.643929117918,2.54365621171892));
#73374=CARTESIAN_POINT('Ctrl Pts',(18.3,40.643929117918,2.68117321692407));
#73375=CARTESIAN_POINT('',(18.18,40.5140519380569,2.45143247805536));
#73376=CARTESIAN_POINT('',(18.3,40.5140519380569,2.45143247805536));
#73377=CARTESIAN_POINT('Ctrl Pts',(18.18,40.5140519380569,2.45143247805536));
#73378=CARTESIAN_POINT('Ctrl Pts',(18.18,40.643929117918,2.54365621171892));
#73379=CARTESIAN_POINT('Ctrl Pts',(18.18,40.643929117918,2.68117321692407));
#73380=CARTESIAN_POINT('Ctrl Pts',(18.3,39.9890859663486,2.3592087443918));
#73381=CARTESIAN_POINT('Ctrl Pts',(18.1272,39.9890859663486,2.3592087443918));
#73382=CARTESIAN_POINT('Ctrl Pts',(18.3,40.3841746091843,2.3592087443918));
#73383=CARTESIAN_POINT('Ctrl Pts',(18.1272,40.3841746091843,2.3592087443918));
#73384=CARTESIAN_POINT('Ctrl Pts',(18.3,40.5140519380569,2.45143247805536));
#73385=CARTESIAN_POINT('Ctrl Pts',(18.1272,40.5140519380569,2.45143247805536));
#73386=CARTESIAN_POINT('',(18.3,39.9890859663486,2.3592087443918));
#73387=CARTESIAN_POINT('Ctrl Pts',(18.3,39.9890859663486,2.3592087443918));
#73388=CARTESIAN_POINT('Ctrl Pts',(18.3,40.3841746091843,2.3592087443918));
#73389=CARTESIAN_POINT('Ctrl Pts',(18.3,40.5140519380569,2.45143247805536));
#73390=CARTESIAN_POINT('',(18.18,39.9890859663486,2.3592087443918));
#73391=CARTESIAN_POINT('',(18.3,39.9890859663486,2.3592087443918));
#73392=CARTESIAN_POINT('Ctrl Pts',(18.18,39.9890859663486,2.3592087443918));
#73393=CARTESIAN_POINT('Ctrl Pts',(18.18,40.3841746091843,2.3592087443918));
#73394=CARTESIAN_POINT('Ctrl Pts',(18.18,40.5140519380569,2.45143247805536));
#73395=CARTESIAN_POINT('Ctrl Pts',(18.3,39.4652115046978,2.45143247805536));
#73396=CARTESIAN_POINT('Ctrl Pts',(18.1272,39.4652115046978,2.45143247805536));
#73397=CARTESIAN_POINT('Ctrl Pts',(18.3,39.5961801946163,2.3592087443918));
#73398=CARTESIAN_POINT('Ctrl Pts',(18.1272,39.5961801946163,2.3592087443918));
#73399=CARTESIAN_POINT('Ctrl Pts',(18.3,39.9890859663486,2.3592087443918));
#73400=CARTESIAN_POINT('Ctrl Pts',(18.1272,39.9890859663486,2.3592087443918));
#73401=CARTESIAN_POINT('',(18.3,39.4652115046978,2.45143247805536));
#73402=CARTESIAN_POINT('Ctrl Pts',(18.3,39.4652115046978,2.45143247805536));
#73403=CARTESIAN_POINT('Ctrl Pts',(18.3,39.5961801946163,2.3592087443918));
#73404=CARTESIAN_POINT('Ctrl Pts',(18.3,39.9890859663486,2.3592087443918));
#73405=CARTESIAN_POINT('',(18.18,39.4652115046978,2.45143247805536));
#73406=CARTESIAN_POINT('',(18.3,39.4652115046978,2.45143247805536));
#73407=CARTESIAN_POINT('Ctrl Pts',(18.18,39.4652115046978,2.45143247805536));
#73408=CARTESIAN_POINT('Ctrl Pts',(18.18,39.5961801946163,2.3592087443918));
#73409=CARTESIAN_POINT('Ctrl Pts',(18.18,39.9890859663486,2.3592087443918));
#73410=CARTESIAN_POINT('Ctrl Pts',(18.3,39.3342428147793,2.67899034582078));
#73411=CARTESIAN_POINT('Ctrl Pts',(18.1272,39.3342428147793,2.67899034582078));
#73412=CARTESIAN_POINT('Ctrl Pts',(18.3,39.3342428147793,2.54365621171892));
#73413=CARTESIAN_POINT('Ctrl Pts',(18.1272,39.3342428147793,2.54365621171892));
#73414=CARTESIAN_POINT('Ctrl Pts',(18.3,39.4652115046978,2.45143247805536));
#73415=CARTESIAN_POINT('Ctrl Pts',(18.1272,39.4652115046978,2.45143247805536));
#73416=CARTESIAN_POINT('',(18.3,39.3342428147793,2.67899034582078));
#73417=CARTESIAN_POINT('Ctrl Pts',(18.3,39.3342428147793,2.67899034582078));
#73418=CARTESIAN_POINT('Ctrl Pts',(18.3,39.3342428147793,2.54365621171892));
#73419=CARTESIAN_POINT('Ctrl Pts',(18.3,39.4652115046978,2.45143247805536));
#73420=CARTESIAN_POINT('',(18.18,39.3342428147793,2.67899034582078));
#73421=CARTESIAN_POINT('',(18.3,39.3342428147793,2.67899034582078));
#73422=CARTESIAN_POINT('Ctrl Pts',(18.18,39.3342428147793,2.67899034582078));
#73423=CARTESIAN_POINT('Ctrl Pts',(18.18,39.3342428147793,2.54365621171892));
#73424=CARTESIAN_POINT('Ctrl Pts',(18.18,39.4652115046978,2.45143247805536));
#73425=CARTESIAN_POINT('Ctrl Pts',(18.3,39.4646658241749,2.90654836259782));
#73426=CARTESIAN_POINT('Ctrl Pts',(18.1272,39.4646658241749,2.90654836259782));
#73427=CARTESIAN_POINT('Ctrl Pts',(18.3,39.3342428147793,2.81432462893426));
#73428=CARTESIAN_POINT('Ctrl Pts',(18.1272,39.3342428147793,2.81432462893426));
#73429=CARTESIAN_POINT('Ctrl Pts',(18.3,39.3342428147793,2.67899034582078));
#73430=CARTESIAN_POINT('Ctrl Pts',(18.1272,39.3342428147793,2.67899034582078));
#73431=CARTESIAN_POINT('',(18.3,39.4646658241749,2.90654836259782));
#73432=CARTESIAN_POINT('Ctrl Pts',(18.3,39.4646658241749,2.90654836259782));
#73433=CARTESIAN_POINT('Ctrl Pts',(18.3,39.3342428147793,2.81432462893426));
#73434=CARTESIAN_POINT('Ctrl Pts',(18.3,39.3342428147793,2.67899034582078));
#73435=CARTESIAN_POINT('',(18.18,39.4646658241749,2.90654836259782));
#73436=CARTESIAN_POINT('',(18.3,39.4646658241749,2.90654836259782));
#73437=CARTESIAN_POINT('Ctrl Pts',(18.18,39.4646658241749,2.90654836259782));
#73438=CARTESIAN_POINT('Ctrl Pts',(18.18,39.3342428147793,2.81432462893426));
#73439=CARTESIAN_POINT('Ctrl Pts',(18.18,39.3342428147793,2.67899034582078));
#73440=CARTESIAN_POINT('Ctrl Pts',(18.3,39.9890859663486,2.99877209626138));
#73441=CARTESIAN_POINT('Ctrl Pts',(18.1272,39.9890859663486,2.99877209626138));
#73442=CARTESIAN_POINT('Ctrl Pts',(18.3,39.5950888335705,2.99877209626138));
#73443=CARTESIAN_POINT('Ctrl Pts',(18.1272,39.5950888335705,2.99877209626138));
#73444=CARTESIAN_POINT('Ctrl Pts',(18.3,39.4646658241749,2.90654836259782));
#73445=CARTESIAN_POINT('Ctrl Pts',(18.1272,39.4646658241749,2.90654836259782));
#73446=CARTESIAN_POINT('',(18.3,39.9890859663486,2.99877209626138));
#73447=CARTESIAN_POINT('Ctrl Pts',(18.3,39.9890859663486,2.99877209626138));
#73448=CARTESIAN_POINT('Ctrl Pts',(18.3,39.5950888335705,2.99877209626138));
#73449=CARTESIAN_POINT('Ctrl Pts',(18.3,39.4646658241749,2.90654836259782));
#73450=CARTESIAN_POINT('',(18.18,39.9890859663486,2.99877209626138));
#73451=CARTESIAN_POINT('',(18.3,39.9890859663486,2.99877209626138));
#73452=CARTESIAN_POINT('Ctrl Pts',(18.18,39.9890859663486,2.99877209626138));
#73453=CARTESIAN_POINT('Ctrl Pts',(18.18,39.5950888335705,2.99877209626138));
#73454=CARTESIAN_POINT('Ctrl Pts',(18.18,39.4646658241749,2.90654836259782));
#73455=CARTESIAN_POINT('Ctrl Pts',(18.3,40.5293315887451,2.89727149568498));
#73456=CARTESIAN_POINT('Ctrl Pts',(18.1272,40.5293315887451,2.89727149568498));
#73457=CARTESIAN_POINT('Ctrl Pts',(18.3,40.3830830991268,2.99877209626138));
#73458=CARTESIAN_POINT('Ctrl Pts',(18.1272,40.3830830991268,2.99877209626138));
#73459=CARTESIAN_POINT('Ctrl Pts',(18.3,39.9890859663486,2.99877209626138));
#73460=CARTESIAN_POINT('Ctrl Pts',(18.1272,39.9890859663486,2.99877209626138));
#73461=CARTESIAN_POINT('Ctrl Pts',(18.3,40.5293315887451,2.89727149568498));
#73462=CARTESIAN_POINT('Ctrl Pts',(18.3,40.3830830991268,2.99877209626138));
#73463=CARTESIAN_POINT('Ctrl Pts',(18.3,39.9890859663486,2.99877209626138));
#73464=CARTESIAN_POINT('Ctrl Pts',(18.18,40.5293315887451,2.89727149568498));
#73465=CARTESIAN_POINT('Ctrl Pts',(18.18,40.3830830991268,2.99877209626138));
#73466=CARTESIAN_POINT('Ctrl Pts',(18.18,39.9890859663486,2.99877209626138));
#73467=CARTESIAN_POINT('Ctrl Pts',(18.3,39.1727148234844,2.67899034582078));
#73468=CARTESIAN_POINT('Ctrl Pts',(18.1272,39.1727148234844,2.67899034582078));
#73469=CARTESIAN_POINT('Ctrl Pts',(18.3,39.1727148234844,2.91036827526987));
#73470=CARTESIAN_POINT('Ctrl Pts',(18.1272,39.1727148234844,2.91036827526987));
#73471=CARTESIAN_POINT('Ctrl Pts',(18.3,39.3386085569858,3.04242832623422));
#73472=CARTESIAN_POINT('Ctrl Pts',(18.1272,39.3386085569858,3.04242832623422));
#73473=CARTESIAN_POINT('',(18.3,39.1727148234844,2.67899034582078));
#73474=CARTESIAN_POINT('',(18.3,39.3386085569858,3.04242832623422));
#73475=CARTESIAN_POINT('Ctrl Pts',(18.3,39.1727148234844,2.67899034582078));
#73476=CARTESIAN_POINT('Ctrl Pts',(18.3,39.1727148234844,2.91036827526987));
#73477=CARTESIAN_POINT('Ctrl Pts',(18.3,39.3386085569858,3.04242832623422));
#73478=CARTESIAN_POINT('',(18.18,39.1727148234844,2.67899034582078));
#73479=CARTESIAN_POINT('',(18.3,39.1727148234844,2.67899034582078));
#73480=CARTESIAN_POINT('',(18.18,39.3386085569858,3.04242832623422));
#73481=CARTESIAN_POINT('Ctrl Pts',(18.18,39.1727148234844,2.67899034582078));
#73482=CARTESIAN_POINT('Ctrl Pts',(18.18,39.1727148234844,2.91036827526987));
#73483=CARTESIAN_POINT('Ctrl Pts',(18.18,39.3386085569858,3.04242832623422));
#73484=CARTESIAN_POINT('',(18.3,39.3386085569858,3.04242832623422));
#73485=CARTESIAN_POINT('Ctrl Pts',(18.3,39.2671214282513,2.38813100419939));
#73486=CARTESIAN_POINT('Ctrl Pts',(18.1272,39.2671214282513,2.38813100419939));
#73487=CARTESIAN_POINT('Ctrl Pts',(18.3,39.1727148234844,2.5032742138952));
#73488=CARTESIAN_POINT('Ctrl Pts',(18.1272,39.1727148234844,2.5032742138952));
#73489=CARTESIAN_POINT('Ctrl Pts',(18.3,39.1727148234844,2.67899034582078));
#73490=CARTESIAN_POINT('Ctrl Pts',(18.1272,39.1727148234844,2.67899034582078));
#73491=CARTESIAN_POINT('',(18.3,39.2671214282513,2.38813100419939));
#73492=CARTESIAN_POINT('Ctrl Pts',(18.3,39.2671214282513,2.38813100419939));
#73493=CARTESIAN_POINT('Ctrl Pts',(18.3,39.1727148234844,2.5032742138952));
#73494=CARTESIAN_POINT('Ctrl Pts',(18.3,39.1727148234844,2.67899034582078));
#73495=CARTESIAN_POINT('',(18.18,39.2671214282513,2.38813100419939));
#73496=CARTESIAN_POINT('',(18.3,39.2671214282513,2.38813100419939));
#73497=CARTESIAN_POINT('Ctrl Pts',(18.18,39.2671214282513,2.38813100419939));
#73498=CARTESIAN_POINT('Ctrl Pts',(18.18,39.1727148234844,2.5032742138952));
#73499=CARTESIAN_POINT('Ctrl Pts',(18.18,39.1727148234844,2.67899034582078));
#73500=CARTESIAN_POINT('Ctrl Pts',(18.3,39.5345156133175,2.2151432748884));
#73501=CARTESIAN_POINT('Ctrl Pts',(18.1272,39.5345156133175,2.2151432748884));
#73502=CARTESIAN_POINT('Ctrl Pts',(18.3,39.3615280330181,2.27298764549196));
#73503=CARTESIAN_POINT('Ctrl Pts',(18.1272,39.3615280330181,2.27298764549196));
#73504=CARTESIAN_POINT('Ctrl Pts',(18.3,39.2671214282513,2.38813100419939));
#73505=CARTESIAN_POINT('Ctrl Pts',(18.1272,39.2671214282513,2.38813100419939));
#73506=CARTESIAN_POINT('',(18.3,39.5345156133175,2.2151432748884));
#73507=CARTESIAN_POINT('Ctrl Pts',(18.3,39.5345156133175,2.2151432748884));
#73508=CARTESIAN_POINT('Ctrl Pts',(18.3,39.3615280330181,2.27298764549196));
#73509=CARTESIAN_POINT('Ctrl Pts',(18.3,39.2671214282513,2.38813100419939));
#73510=CARTESIAN_POINT('',(18.18,39.5345156133175,2.2151432748884));
#73511=CARTESIAN_POINT('',(18.3,39.5345156133175,2.2151432748884));
#73512=CARTESIAN_POINT('Ctrl Pts',(18.18,39.5345156133175,2.2151432748884));
#73513=CARTESIAN_POINT('Ctrl Pts',(18.18,39.3615280330181,2.27298764549196));
#73514=CARTESIAN_POINT('Ctrl Pts',(18.18,39.2671214282513,2.38813100419939));
#73515=CARTESIAN_POINT('Ctrl Pts',(18.3,39.9890859663486,2.15729875527322));
#73516=CARTESIAN_POINT('Ctrl Pts',(18.1272,39.9890859663486,2.15729875527322));
#73517=CARTESIAN_POINT('Ctrl Pts',(18.3,39.7075034916401,2.15729875527322));
#73518=CARTESIAN_POINT('Ctrl Pts',(18.1272,39.7075034916401,2.15729875527322));
#73519=CARTESIAN_POINT('Ctrl Pts',(18.3,39.5345156133175,2.2151432748884));
#73520=CARTESIAN_POINT('Ctrl Pts',(18.1272,39.5345156133175,2.2151432748884));
#73521=CARTESIAN_POINT('',(18.3,39.9890859663486,2.15729875527322));
#73522=CARTESIAN_POINT('Ctrl Pts',(18.3,39.9890859663486,2.15729875527322));
#73523=CARTESIAN_POINT('Ctrl Pts',(18.3,39.7075034916401,2.15729875527322));
#73524=CARTESIAN_POINT('Ctrl Pts',(18.3,39.5345156133175,2.2151432748884));
#73525=CARTESIAN_POINT('',(18.18,39.9890859663486,2.15729875527322));
#73526=CARTESIAN_POINT('',(18.3,39.9890859663486,2.15729875527322));
#73527=CARTESIAN_POINT('Ctrl Pts',(18.18,39.9890859663486,2.15729875527322));
#73528=CARTESIAN_POINT('Ctrl Pts',(18.18,39.7075034916401,2.15729875527322));
#73529=CARTESIAN_POINT('Ctrl Pts',(18.18,39.5345156133175,2.2151432748884));
#73530=CARTESIAN_POINT('Ctrl Pts',(18.3,40.3672577679157,2.19331515990198));
#73531=CARTESIAN_POINT('Ctrl Pts',(18.1272,40.3672577679157,2.19331515990198));
#73532=CARTESIAN_POINT('Ctrl Pts',(18.3,40.2270122110844,2.15729875527322));
#73533=CARTESIAN_POINT('Ctrl Pts',(18.1272,40.2270122110844,2.15729875527322));
#73534=CARTESIAN_POINT('Ctrl Pts',(18.3,39.9890859663486,2.15729875527322));
#73535=CARTESIAN_POINT('Ctrl Pts',(18.1272,39.9890859663486,2.15729875527322));
#73536=CARTESIAN_POINT('',(18.3,40.3672577679157,2.19331515990198));
#73537=CARTESIAN_POINT('Ctrl Pts',(18.3,40.3672577679157,2.19331515990198));
#73538=CARTESIAN_POINT('Ctrl Pts',(18.3,40.2270122110844,2.15729875527322));
#73539=CARTESIAN_POINT('Ctrl Pts',(18.3,39.9890859663486,2.15729875527322));
#73540=CARTESIAN_POINT('',(18.18,40.3672577679157,2.19331515990198));
#73541=CARTESIAN_POINT('',(18.3,40.3672577679157,2.19331515990198));
#73542=CARTESIAN_POINT('Ctrl Pts',(18.18,40.3672577679157,2.19331515990198));
#73543=CARTESIAN_POINT('Ctrl Pts',(18.18,40.2270122110844,2.15729875527322));
#73544=CARTESIAN_POINT('Ctrl Pts',(18.18,39.9890859663486,2.15729875527322));
#73545=CARTESIAN_POINT('Ctrl Pts',(18.3,40.605184161663,2.2926330383867));
#73546=CARTESIAN_POINT('Ctrl Pts',(18.1272,40.605184161663,2.2926330383867));
#73547=CARTESIAN_POINT('Ctrl Pts',(18.3,40.5075034737587,2.22933141551912));
#73548=CARTESIAN_POINT('Ctrl Pts',(18.1272,40.5075034737587,2.22933141551912));
#73549=CARTESIAN_POINT('Ctrl Pts',(18.3,40.3672577679157,2.19331515990198));
#73550=CARTESIAN_POINT('Ctrl Pts',(18.1272,40.3672577679157,2.19331515990198));
#73551=CARTESIAN_POINT('',(18.3,40.605184161663,2.2926330383867));
#73552=CARTESIAN_POINT('Ctrl Pts',(18.3,40.605184161663,2.2926330383867));
#73553=CARTESIAN_POINT('Ctrl Pts',(18.3,40.5075034737587,2.22933141551912));
#73554=CARTESIAN_POINT('Ctrl Pts',(18.3,40.3672577679157,2.19331515990198));
#73555=CARTESIAN_POINT('',(18.18,40.605184161663,2.2926330383867));
#73556=CARTESIAN_POINT('',(18.3,40.605184161663,2.2926330383867));
#73557=CARTESIAN_POINT('Ctrl Pts',(18.18,40.605184161663,2.2926330383867));
#73558=CARTESIAN_POINT('Ctrl Pts',(18.18,40.5075034737587,2.22933141551912));
#73559=CARTESIAN_POINT('Ctrl Pts',(18.18,40.3672577679157,2.19331515990198));
#73560=CARTESIAN_POINT('Ctrl Pts',(18.3,40.7547067344189,2.45306966863573));
#73561=CARTESIAN_POINT('Ctrl Pts',(18.1272,40.7547067344189,2.45306966863573));
#73562=CARTESIAN_POINT('Ctrl Pts',(18.3,40.702864998579,2.35593451224267));
#73563=CARTESIAN_POINT('Ctrl Pts',(18.1272,40.702864998579,2.35593451224267));
#73564=CARTESIAN_POINT('Ctrl Pts',(18.3,40.605184161663,2.2926330383867));
#73565=CARTESIAN_POINT('Ctrl Pts',(18.1272,40.605184161663,2.2926330383867));
#73566=CARTESIAN_POINT('',(18.3,40.7547067344189,2.45306966863573));
#73567=CARTESIAN_POINT('Ctrl Pts',(18.3,40.7547067344189,2.45306966863573));
#73568=CARTESIAN_POINT('Ctrl Pts',(18.3,40.702864998579,2.35593451224267));
#73569=CARTESIAN_POINT('Ctrl Pts',(18.3,40.605184161663,2.2926330383867));
#73570=CARTESIAN_POINT('',(18.18,40.7547067344189,2.45306966863573));
#73571=CARTESIAN_POINT('',(18.3,40.7547067344189,2.45306966863573));
#73572=CARTESIAN_POINT('Ctrl Pts',(18.18,40.7547067344189,2.45306966863573));
#73573=CARTESIAN_POINT('Ctrl Pts',(18.18,40.702864998579,2.35593451224267));
#73574=CARTESIAN_POINT('Ctrl Pts',(18.18,40.605184161663,2.2926330383867));
#73575=CARTESIAN_POINT('Ctrl Pts',(18.3,40.8065484702587,2.67899034582078));
#73576=CARTESIAN_POINT('Ctrl Pts',(18.1272,40.8065484702587,2.67899034582078));
#73577=CARTESIAN_POINT('Ctrl Pts',(18.3,40.8065484702587,2.55020467601716));
#73578=CARTESIAN_POINT('Ctrl Pts',(18.1272,40.8065484702587,2.55020467601716));
#73579=CARTESIAN_POINT('Ctrl Pts',(18.3,40.7547067344189,2.45306966863573));
#73580=CARTESIAN_POINT('Ctrl Pts',(18.1272,40.7547067344189,2.45306966863573));
#73581=CARTESIAN_POINT('',(18.3,40.8065484702587,2.67899034582078));
#73582=CARTESIAN_POINT('Ctrl Pts',(18.3,40.8065484702587,2.67899034582078));
#73583=CARTESIAN_POINT('Ctrl Pts',(18.3,40.8065484702587,2.55020467601716));
#73584=CARTESIAN_POINT('Ctrl Pts',(18.3,40.7547067344189,2.45306966863573));
#73585=CARTESIAN_POINT('',(18.18,40.8065484702587,2.67899034582078));
#73586=CARTESIAN_POINT('',(18.3,40.8065484702587,2.67899034582078));
#73587=CARTESIAN_POINT('Ctrl Pts',(18.18,40.8065484702587,2.67899034582078));
#73588=CARTESIAN_POINT('Ctrl Pts',(18.18,40.8065484702587,2.55020467601716));
#73589=CARTESIAN_POINT('Ctrl Pts',(18.18,40.7547067344189,2.45306966863573));
#73590=CARTESIAN_POINT('Ctrl Pts',(18.3,40.7126876950264,2.96875847540796));
#73591=CARTESIAN_POINT('Ctrl Pts',(18.1272,40.7126876950264,2.96875847540796));
#73592=CARTESIAN_POINT('Ctrl Pts',(18.3,40.8065484702587,2.85361526571214));
#73593=CARTESIAN_POINT('Ctrl Pts',(18.1272,40.8065484702587,2.85361526571214));
#73594=CARTESIAN_POINT('Ctrl Pts',(18.3,40.8065484702587,2.67899034582078));
#73595=CARTESIAN_POINT('Ctrl Pts',(18.1272,40.8065484702587,2.67899034582078));
#73596=CARTESIAN_POINT('',(18.3,40.7126876950264,2.96875847540796));
#73597=CARTESIAN_POINT('Ctrl Pts',(18.3,40.7126876950264,2.96875847540796));
#73598=CARTESIAN_POINT('Ctrl Pts',(18.3,40.8065484702587,2.85361526571214));
#73599=CARTESIAN_POINT('Ctrl Pts',(18.3,40.8065484702587,2.67899034582078));
#73600=CARTESIAN_POINT('',(18.18,40.7126876950264,2.96875847540796));
#73601=CARTESIAN_POINT('',(18.3,40.7126876950264,2.96875847540796));
#73602=CARTESIAN_POINT('Ctrl Pts',(18.18,40.7126876950264,2.96875847540796));
#73603=CARTESIAN_POINT('Ctrl Pts',(18.18,40.8065484702587,2.85361526571214));
#73604=CARTESIAN_POINT('Ctrl Pts',(18.18,40.8065484702587,2.67899034582078));
#73605=CARTESIAN_POINT('Ctrl Pts',(18.3,40.4458390414715,3.14229188524187));
#73606=CARTESIAN_POINT('Ctrl Pts',(18.1272,40.4458390414715,3.14229188524187));
#73607=CARTESIAN_POINT('Ctrl Pts',(18.3,40.6188267707825,3.08390168510377));
#73608=CARTESIAN_POINT('Ctrl Pts',(18.1272,40.6188267707825,3.08390168510377));
#73609=CARTESIAN_POINT('Ctrl Pts',(18.3,40.7126876950264,2.96875847540796));
#73610=CARTESIAN_POINT('Ctrl Pts',(18.1272,40.7126876950264,2.96875847540796));
#73611=CARTESIAN_POINT('',(18.3,40.4458390414715,3.14229188524187));
#73612=CARTESIAN_POINT('Ctrl Pts',(18.3,40.4458390414715,3.14229188524187));
#73613=CARTESIAN_POINT('Ctrl Pts',(18.3,40.6188267707825,3.08390168510377));
#73614=CARTESIAN_POINT('Ctrl Pts',(18.3,40.7126876950264,2.96875847540796));
#73615=CARTESIAN_POINT('',(18.18,40.4458390414715,3.14229188524187));
#73616=CARTESIAN_POINT('',(18.3,40.4458390414715,3.14229188524187));
#73617=CARTESIAN_POINT('Ctrl Pts',(18.18,40.4458390414715,3.14229188524187));
#73618=CARTESIAN_POINT('Ctrl Pts',(18.18,40.6188267707825,3.08390168510377));
#73619=CARTESIAN_POINT('Ctrl Pts',(18.18,40.7126876950264,2.96875847540796));
#73620=CARTESIAN_POINT('Ctrl Pts',(18.3,39.9890859663486,3.20068208537996));
#73621=CARTESIAN_POINT('Ctrl Pts',(18.1272,39.9890859663486,3.20068208537996));
#73622=CARTESIAN_POINT('Ctrl Pts',(18.3,40.2728513121605,3.20068208537996));
#73623=CARTESIAN_POINT('Ctrl Pts',(18.1272,40.2728513121605,3.20068208537996));
#73624=CARTESIAN_POINT('Ctrl Pts',(18.3,40.4458390414715,3.14229188524187));
#73625=CARTESIAN_POINT('Ctrl Pts',(18.1272,40.4458390414715,3.14229188524187));
#73626=CARTESIAN_POINT('',(18.3,39.9890859663486,3.20068208537996));
#73627=CARTESIAN_POINT('Ctrl Pts',(18.3,39.9890859663486,3.20068208537996));
#73628=CARTESIAN_POINT('Ctrl Pts',(18.3,40.2728513121605,3.20068208537996));
#73629=CARTESIAN_POINT('Ctrl Pts',(18.3,40.4458390414715,3.14229188524187));
#73630=CARTESIAN_POINT('',(18.18,39.9890859663486,3.20068208537996));
#73631=CARTESIAN_POINT('',(18.3,39.9890859663486,3.20068208537996));
#73632=CARTESIAN_POINT('Ctrl Pts',(18.18,39.9890859663486,3.20068208537996));
#73633=CARTESIAN_POINT('Ctrl Pts',(18.18,40.2728513121605,3.20068208537996));
#73634=CARTESIAN_POINT('Ctrl Pts',(18.18,40.4458390414715,3.14229188524187));
#73635=CARTESIAN_POINT('Ctrl Pts',(18.3,39.3386085569858,3.04242832623422));
#73636=CARTESIAN_POINT('Ctrl Pts',(18.1272,39.3386085569858,3.04242832623422));
#73637=CARTESIAN_POINT('Ctrl Pts',(18.3,39.5383356750011,3.20068208537996));
#73638=CARTESIAN_POINT('Ctrl Pts',(18.1272,39.5383356750011,3.20068208537996));
#73639=CARTESIAN_POINT('Ctrl Pts',(18.3,39.9890859663486,3.20068208537996));
#73640=CARTESIAN_POINT('Ctrl Pts',(18.1272,39.9890859663486,3.20068208537996));
#73641=CARTESIAN_POINT('Ctrl Pts',(18.3,39.3386085569858,3.04242832623422));
#73642=CARTESIAN_POINT('Ctrl Pts',(18.3,39.5383356750011,3.20068208537996));
#73643=CARTESIAN_POINT('Ctrl Pts',(18.3,39.9890859663486,3.20068208537996));
#73644=CARTESIAN_POINT('Ctrl Pts',(18.18,39.3386085569858,3.04242832623422));
#73645=CARTESIAN_POINT('Ctrl Pts',(18.18,39.5383356750011,3.20068208537996));
#73646=CARTESIAN_POINT('Ctrl Pts',(18.18,39.9890859663486,3.20068208537996));
#73647=CARTESIAN_POINT('Origin',(18.18,39.9890859663486,3.29999992661178));
#73648=CARTESIAN_POINT('Ctrl Pts',(18.3,39.1716234624386,3.93410628698766));
#73649=CARTESIAN_POINT('Ctrl Pts',(18.1272,39.1716234624386,3.93410628698766));
#73650=CARTESIAN_POINT('Ctrl Pts',(18.3,39.1716234624386,4.14474749974906));
#73651=CARTESIAN_POINT('Ctrl Pts',(18.1272,39.1716234624386,4.14474749974906));
#73652=CARTESIAN_POINT('Ctrl Pts',(18.3,39.2971350491047,4.28390165828168));
#73653=CARTESIAN_POINT('Ctrl Pts',(18.1272,39.2971350491047,4.28390165828168));
#73654=CARTESIAN_POINT('',(18.3,39.1716234624386,3.93410628698766));
#73655=CARTESIAN_POINT('',(18.3,39.2971350491047,4.28390165828168));
#73656=CARTESIAN_POINT('Ctrl Pts',(18.3,39.1716234624386,3.93410628698766));
#73657=CARTESIAN_POINT('Ctrl Pts',(18.3,39.1716234624386,4.14474749974906));
#73658=CARTESIAN_POINT('Ctrl Pts',(18.3,39.2971350491047,4.28390165828168));
#73659=CARTESIAN_POINT('',(18.18,39.1716234624386,3.93410628698766));
#73660=CARTESIAN_POINT('',(18.3,39.1716234624386,3.93410628698766));
#73661=CARTESIAN_POINT('',(18.18,39.2971350491047,4.28390165828168));
#73662=CARTESIAN_POINT('Ctrl Pts',(18.18,39.1716234624386,3.93410628698766));
#73663=CARTESIAN_POINT('Ctrl Pts',(18.18,39.1716234624386,4.14474749974906));
#73664=CARTESIAN_POINT('Ctrl Pts',(18.18,39.2971350491047,4.28390165828168));
#73665=CARTESIAN_POINT('',(18.3,39.2971350491047,4.28390165828168));
#73666=CARTESIAN_POINT('Ctrl Pts',(18.3,39.3173261225223,3.54774890504777));
#73667=CARTESIAN_POINT('Ctrl Pts',(18.1272,39.3173261225223,3.54774890504777));
#73668=CARTESIAN_POINT('Ctrl Pts',(18.3,39.1716234624386,3.70054563544691));
#73669=CARTESIAN_POINT('Ctrl Pts',(18.1272,39.1716234624386,3.70054563544691));
#73670=CARTESIAN_POINT('Ctrl Pts',(18.3,39.1716234624386,3.93410628698766));
#73671=CARTESIAN_POINT('Ctrl Pts',(18.1272,39.1716234624386,3.93410628698766));
#73672=CARTESIAN_POINT('',(18.3,39.3173261225223,3.54774890504777));
#73673=CARTESIAN_POINT('Ctrl Pts',(18.3,39.3173261225223,3.54774890504777));
#73674=CARTESIAN_POINT('Ctrl Pts',(18.3,39.1716234624386,3.70054563544691));
#73675=CARTESIAN_POINT('Ctrl Pts',(18.3,39.1716234624386,3.93410628698766));
#73676=CARTESIAN_POINT('',(18.18,39.3173261225223,3.54774890504777));
#73677=CARTESIAN_POINT('',(18.3,39.3173261225223,3.54774890504777));
#73678=CARTESIAN_POINT('Ctrl Pts',(18.18,39.3173261225223,3.54774890504777));
#73679=CARTESIAN_POINT('Ctrl Pts',(18.18,39.1716234624386,3.70054563544691));
#73680=CARTESIAN_POINT('Ctrl Pts',(18.18,39.1716234624386,3.93410628698766));
#73681=CARTESIAN_POINT('Ctrl Pts',(18.3,39.6725784480572,3.39495224915445));
#73682=CARTESIAN_POINT('Ctrl Pts',(18.1272,39.6725784480572,3.39495224915445));
#73683=CARTESIAN_POINT('Ctrl Pts',(18.3,39.4630287826061,3.39495224915445));
#73684=CARTESIAN_POINT('Ctrl Pts',(18.1272,39.4630287826061,3.39495224915445));
#73685=CARTESIAN_POINT('Ctrl Pts',(18.3,39.3173261225223,3.54774890504777));
#73686=CARTESIAN_POINT('Ctrl Pts',(18.1272,39.3173261225223,3.54774890504777));
#73687=CARTESIAN_POINT('',(18.3,39.6725784480572,3.39495224915445));
#73688=CARTESIAN_POINT('Ctrl Pts',(18.3,39.6725784480572,3.39495224915445));
#73689=CARTESIAN_POINT('Ctrl Pts',(18.3,39.4630287826061,3.39495224915445));
#73690=CARTESIAN_POINT('Ctrl Pts',(18.3,39.3173261225223,3.54774890504777));
#73691=CARTESIAN_POINT('',(18.18,39.6725784480572,3.39495224915445));
#73692=CARTESIAN_POINT('',(18.3,39.6725784480572,3.39495224915445));
#73693=CARTESIAN_POINT('Ctrl Pts',(18.18,39.6725784480572,3.39495224915445));
#73694=CARTESIAN_POINT('Ctrl Pts',(18.18,39.4630287826061,3.39495224915445));
#73695=CARTESIAN_POINT('Ctrl Pts',(18.18,39.3173261225223,3.54774890504777));
#73696=CARTESIAN_POINT('Ctrl Pts',(18.3,39.9306957662105,3.47353329919279));
#73697=CARTESIAN_POINT('Ctrl Pts',(18.1272,39.9306957662105,3.47353329919279));
#73698=CARTESIAN_POINT('Ctrl Pts',(18.3,39.8275579750538,3.39495224915445));
#73699=CARTESIAN_POINT('Ctrl Pts',(18.1272,39.8275579750538,3.39495224915445));
#73700=CARTESIAN_POINT('Ctrl Pts',(18.3,39.6725784480572,3.39495224915445));
#73701=CARTESIAN_POINT('Ctrl Pts',(18.1272,39.6725784480572,3.39495224915445));
#73702=CARTESIAN_POINT('',(18.3,39.9306957662105,3.47353329919279));
#73703=CARTESIAN_POINT('Ctrl Pts',(18.3,39.9306957662105,3.47353329919279));
#73704=CARTESIAN_POINT('Ctrl Pts',(18.3,39.8275579750538,3.39495224915445));
#73705=CARTESIAN_POINT('Ctrl Pts',(18.3,39.6725784480572,3.39495224915445));
#73706=CARTESIAN_POINT('',(18.18,39.9306957662105,3.47353329919279));
#73707=CARTESIAN_POINT('',(18.3,39.9306957662105,3.47353329919279));
#73708=CARTESIAN_POINT('Ctrl Pts',(18.18,39.9306957662105,3.47353329919279));
#73709=CARTESIAN_POINT('Ctrl Pts',(18.18,39.8275579750538,3.39495224915445));
#73710=CARTESIAN_POINT('Ctrl Pts',(18.18,39.6725784480572,3.39495224915445));
#73711=CARTESIAN_POINT('Ctrl Pts',(18.3,40.0665757298469,3.69399717114866));
#73712=CARTESIAN_POINT('Ctrl Pts',(18.1272,40.0665757298469,3.69399717114866));
#73713=CARTESIAN_POINT('Ctrl Pts',(18.3,40.0338335573673,3.55211449824274));
#73714=CARTESIAN_POINT('Ctrl Pts',(18.1272,40.0338335573673,3.55211449824274));
#73715=CARTESIAN_POINT('Ctrl Pts',(18.3,39.9306957662105,3.47353329919279));
#73716=CARTESIAN_POINT('Ctrl Pts',(18.1272,39.9306957662105,3.47353329919279));
#73717=CARTESIAN_POINT('',(18.3,40.0665757298469,3.69399717114866));
#73718=CARTESIAN_POINT('Ctrl Pts',(18.3,40.0665757298469,3.69399717114866));
#73719=CARTESIAN_POINT('Ctrl Pts',(18.3,40.0338335573673,3.55211449824274));
#73720=CARTESIAN_POINT('Ctrl Pts',(18.3,39.9306957662105,3.47353329919279));
#73721=CARTESIAN_POINT('',(18.18,40.0665757298469,3.69399717114866));
#73722=CARTESIAN_POINT('',(18.3,40.0665757298469,3.69399717114866));
#73723=CARTESIAN_POINT('Ctrl Pts',(18.18,40.0665757298469,3.69399717114866));
#73724=CARTESIAN_POINT('Ctrl Pts',(18.18,40.0338335573673,3.55211449824274));
#73725=CARTESIAN_POINT('Ctrl Pts',(18.18,39.9306957662105,3.47353329919279));
#73726=CARTESIAN_POINT('Ctrl Pts',(18.3,40.2019100129604,3.52919502221048));
#73727=CARTESIAN_POINT('Ctrl Pts',(18.1272,40.2019100129604,3.52919502221048));
#73728=CARTESIAN_POINT('Ctrl Pts',(18.3,40.1167802751064,3.58485667072237));
#73729=CARTESIAN_POINT('Ctrl Pts',(18.1272,40.1167802751064,3.58485667072237));
#73730=CARTESIAN_POINT('Ctrl Pts',(18.3,40.0665757298469,3.69399717114866));
#73731=CARTESIAN_POINT('Ctrl Pts',(18.1272,40.0665757298469,3.69399717114866));
#73732=CARTESIAN_POINT('',(18.3,40.2019100129604,3.52919502221048));
#73733=CARTESIAN_POINT('Ctrl Pts',(18.3,40.2019100129604,3.52919502221048));
#73734=CARTESIAN_POINT('Ctrl Pts',(18.3,40.1167802751064,3.58485667072237));
#73735=CARTESIAN_POINT('Ctrl Pts',(18.3,40.0665757298469,3.69399717114866));
#73736=CARTESIAN_POINT('',(18.18,40.2019100129604,3.52919502221048));
#73737=CARTESIAN_POINT('',(18.3,40.2019100129604,3.52919502221048));
#73738=CARTESIAN_POINT('Ctrl Pts',(18.18,40.2019100129604,3.52919502221048));
#73739=CARTESIAN_POINT('Ctrl Pts',(18.18,40.1167802751064,3.58485667072237));
#73740=CARTESIAN_POINT('Ctrl Pts',(18.18,40.0665757298469,3.69399717114866));
#73741=CARTESIAN_POINT('Ctrl Pts',(18.3,40.3907230734825,3.47353329919279));
#73742=CARTESIAN_POINT('Ctrl Pts',(18.1272,40.3907230734825,3.47353329919279));
#73743=CARTESIAN_POINT('Ctrl Pts',(18.3,40.2870396018028,3.47353329919279));
#73744=CARTESIAN_POINT('Ctrl Pts',(18.1272,40.2870396018028,3.47353329919279));
#73745=CARTESIAN_POINT('Ctrl Pts',(18.3,40.2019100129604,3.52919502221048));
#73746=CARTESIAN_POINT('Ctrl Pts',(18.1272,40.2019100129604,3.52919502221048));
#73747=CARTESIAN_POINT('',(18.3,40.3907230734825,3.47353329919279));
#73748=CARTESIAN_POINT('Ctrl Pts',(18.3,40.3907230734825,3.47353329919279));
#73749=CARTESIAN_POINT('Ctrl Pts',(18.3,40.2870396018028,3.47353329919279));
#73750=CARTESIAN_POINT('Ctrl Pts',(18.3,40.2019100129604,3.52919502221048));
#73751=CARTESIAN_POINT('',(18.18,40.3907230734825,3.47353329919279));
#73752=CARTESIAN_POINT('',(18.3,40.3907230734825,3.47353329919279));
#73753=CARTESIAN_POINT('Ctrl Pts',(18.18,40.3907230734825,3.47353329919279));
#73754=CARTESIAN_POINT('Ctrl Pts',(18.18,40.2870396018028,3.47353329919279));
#73755=CARTESIAN_POINT('Ctrl Pts',(18.18,40.2019100129604,3.52919502221048));
#73756=CARTESIAN_POINT('Ctrl Pts',(18.3,40.5969985067844,3.53192349933088));
#73757=CARTESIAN_POINT('Ctrl Pts',(18.1272,40.5969985067844,3.53192349933088));
#73758=CARTESIAN_POINT('Ctrl Pts',(18.3,40.499863499403,3.47353329919279));
#73759=CARTESIAN_POINT('Ctrl Pts',(18.1272,40.499863499403,3.47353329919279));
#73760=CARTESIAN_POINT('Ctrl Pts',(18.3,40.3907230734825,3.47353329919279));
#73761=CARTESIAN_POINT('Ctrl Pts',(18.1272,40.3907230734825,3.47353329919279));
#73762=CARTESIAN_POINT('',(18.3,40.5969985067844,3.53192349933088));
#73763=CARTESIAN_POINT('Ctrl Pts',(18.3,40.5969985067844,3.53192349933088));
#73764=CARTESIAN_POINT('Ctrl Pts',(18.3,40.499863499403,3.47353329919279));
#73765=CARTESIAN_POINT('Ctrl Pts',(18.3,40.3907230734825,3.47353329919279));
#73766=CARTESIAN_POINT('',(18.18,40.5969985067844,3.53192349933088));
#73767=CARTESIAN_POINT('',(18.3,40.5969985067844,3.53192349933088));
#73768=CARTESIAN_POINT('Ctrl Pts',(18.18,40.5969985067844,3.53192349933088));
#73769=CARTESIAN_POINT('Ctrl Pts',(18.18,40.499863499403,3.47353329919279));
#73770=CARTESIAN_POINT('Ctrl Pts',(18.18,40.3907230734825,3.47353329919279));
#73771=CARTESIAN_POINT('Ctrl Pts',(18.3,40.7503409922123,3.70054563544691));
#73772=CARTESIAN_POINT('Ctrl Pts',(18.1272,40.7503409922123,3.70054563544691));
#73773=CARTESIAN_POINT('Ctrl Pts',(18.3,40.6941336631775,3.59031369946897));
#73774=CARTESIAN_POINT('Ctrl Pts',(18.1272,40.6941336631775,3.59031369946897));
#73775=CARTESIAN_POINT('Ctrl Pts',(18.3,40.5969985067844,3.53192349933088));
#73776=CARTESIAN_POINT('Ctrl Pts',(18.1272,40.5969985067844,3.53192349933088));
#73777=CARTESIAN_POINT('',(18.3,40.7503409922123,3.70054563544691));
#73778=CARTESIAN_POINT('Ctrl Pts',(18.3,40.7503409922123,3.70054563544691));
#73779=CARTESIAN_POINT('Ctrl Pts',(18.3,40.6941336631775,3.59031369946897));
#73780=CARTESIAN_POINT('Ctrl Pts',(18.3,40.5969985067844,3.53192349933088));
#73781=CARTESIAN_POINT('',(18.18,40.7503409922123,3.70054563544691));
#73782=CARTESIAN_POINT('',(18.3,40.7503409922123,3.70054563544691));
#73783=CARTESIAN_POINT('Ctrl Pts',(18.18,40.7503409922123,3.70054563544691));
#73784=CARTESIAN_POINT('Ctrl Pts',(18.18,40.6941336631775,3.59031369946897));
#73785=CARTESIAN_POINT('Ctrl Pts',(18.18,40.5969985067844,3.53192349933088));
#73786=CARTESIAN_POINT('Ctrl Pts',(18.3,40.8065483212471,3.94174618683755));
#73787=CARTESIAN_POINT('Ctrl Pts',(18.1272,40.8065483212471,3.94174618683755));
#73788=CARTESIAN_POINT('Ctrl Pts',(18.3,40.8065483212471,3.81077749691904));
#73789=CARTESIAN_POINT('Ctrl Pts',(18.1272,40.8065483212471,3.81077749691904));
#73790=CARTESIAN_POINT('Ctrl Pts',(18.3,40.7503409922123,3.70054563544691));
#73791=CARTESIAN_POINT('Ctrl Pts',(18.1272,40.7503409922123,3.70054563544691));
#73792=CARTESIAN_POINT('',(18.3,40.8065483212471,3.94174618683755));
#73793=CARTESIAN_POINT('Ctrl Pts',(18.3,40.8065483212471,3.94174618683755));
#73794=CARTESIAN_POINT('Ctrl Pts',(18.3,40.8065483212471,3.81077749691904));
#73795=CARTESIAN_POINT('Ctrl Pts',(18.3,40.7503409922123,3.70054563544691));
#73796=CARTESIAN_POINT('',(18.18,40.8065483212471,3.94174618683755));
#73797=CARTESIAN_POINT('',(18.3,40.8065483212471,3.94174618683755));
#73798=CARTESIAN_POINT('Ctrl Pts',(18.18,40.8065483212471,3.94174618683755));
#73799=CARTESIAN_POINT('Ctrl Pts',(18.18,40.8065483212471,3.81077749691904));
#73800=CARTESIAN_POINT('Ctrl Pts',(18.18,40.7503409922123,3.70054563544691));
#73801=CARTESIAN_POINT('Ctrl Pts',(18.3,40.6979535758495,4.25934502892196));
#73802=CARTESIAN_POINT('Ctrl Pts',(18.1272,40.6979535758495,4.25934502892196));
#73803=CARTESIAN_POINT('Ctrl Pts',(18.3,40.8065483212471,4.13165064565837));
#73804=CARTESIAN_POINT('Ctrl Pts',(18.1272,40.8065483212471,4.13165064565837));
#73805=CARTESIAN_POINT('Ctrl Pts',(18.3,40.8065483212471,3.94174618683755));
#73806=CARTESIAN_POINT('Ctrl Pts',(18.1272,40.8065483212471,3.94174618683755));
#73807=CARTESIAN_POINT('',(18.3,40.6979535758495,4.25934502892196));
#73808=CARTESIAN_POINT('Ctrl Pts',(18.3,40.6979535758495,4.25934502892196));
#73809=CARTESIAN_POINT('Ctrl Pts',(18.3,40.8065483212471,4.13165064565837));
#73810=CARTESIAN_POINT('Ctrl Pts',(18.3,40.8065483212471,3.94174618683755));
#73811=CARTESIAN_POINT('',(18.18,40.6979535758495,4.25934502892196));
#73812=CARTESIAN_POINT('',(18.3,40.6979535758495,4.25934502892196));
#73813=CARTESIAN_POINT('Ctrl Pts',(18.18,40.6979535758495,4.25934502892196));
#73814=CARTESIAN_POINT('Ctrl Pts',(18.18,40.8065483212471,4.13165064565837));
#73815=CARTESIAN_POINT('Ctrl Pts',(18.18,40.8065483212471,3.94174618683755));
#73816=CARTESIAN_POINT('Ctrl Pts',(18.3,40.39181458354,4.4230558168143));
#73817=CARTESIAN_POINT('Ctrl Pts',(18.1272,40.39181458354,4.4230558168143));
#73818=CARTESIAN_POINT('Ctrl Pts',(18.3,40.5893586814403,4.38703944943845));
#73819=CARTESIAN_POINT('Ctrl Pts',(18.1272,40.5893586814403,4.38703944943845));
#73820=CARTESIAN_POINT('Ctrl Pts',(18.3,40.6979535758495,4.25934502892196));
#73821=CARTESIAN_POINT('Ctrl Pts',(18.1272,40.6979535758495,4.25934502892196));
#73822=CARTESIAN_POINT('',(18.3,40.39181458354,4.4230558168143));
#73823=CARTESIAN_POINT('Ctrl Pts',(18.3,40.39181458354,4.4230558168143));
#73824=CARTESIAN_POINT('Ctrl Pts',(18.3,40.5893586814403,4.38703944943845));
#73825=CARTESIAN_POINT('Ctrl Pts',(18.3,40.6979535758495,4.25934502892196));
#73826=CARTESIAN_POINT('',(18.18,40.39181458354,4.4230558168143));
#73827=CARTESIAN_POINT('',(18.3,40.39181458354,4.4230558168143));
#73828=CARTESIAN_POINT('Ctrl Pts',(18.18,40.39181458354,4.4230558168143));
#73829=CARTESIAN_POINT('Ctrl Pts',(18.18,40.5893586814403,4.38703944943845));
#73830=CARTESIAN_POINT('Ctrl Pts',(18.18,40.6979535758495,4.25934502892196));
#73831=CARTESIAN_POINT('Origin',(18.3,40.356889539957,4.22660289369523));
#73832=CARTESIAN_POINT('',(18.3,40.356889539957,4.22660289369523));
#73833=CARTESIAN_POINT('',(18.3,40.9206979115535,7.39801776727049));
#73834=CARTESIAN_POINT('',(18.18,40.356889539957,4.22660289369523));
#73835=CARTESIAN_POINT('',(18.3,40.356889539957,4.22660289369523));
#73836=CARTESIAN_POINT('',(18.18,40.356889539957,4.22660289369523));
#73837=CARTESIAN_POINT('Ctrl Pts',(18.3,40.5729876697063,4.12837641350925));
#73838=CARTESIAN_POINT('Ctrl Pts',(18.1272,40.5729876697063,4.12837641350925));
#73839=CARTESIAN_POINT('Ctrl Pts',(18.3,40.5009548604488,4.20477477870882));
#73840=CARTESIAN_POINT('Ctrl Pts',(18.1272,40.5009548604488,4.20477477870882));
#73841=CARTESIAN_POINT('Ctrl Pts',(18.3,40.356889539957,4.22660289369523));
#73842=CARTESIAN_POINT('Ctrl Pts',(18.1272,40.356889539957,4.22660289369523));
#73843=CARTESIAN_POINT('',(18.3,40.5729876697063,4.12837641350925));
#73844=CARTESIAN_POINT('Ctrl Pts',(18.3,40.5729876697063,4.12837641350925));
#73845=CARTESIAN_POINT('Ctrl Pts',(18.3,40.5009548604488,4.20477477870882));
#73846=CARTESIAN_POINT('Ctrl Pts',(18.3,40.356889539957,4.22660289369523));
#73847=CARTESIAN_POINT('',(18.18,40.5729876697063,4.12837641350925));
#73848=CARTESIAN_POINT('',(18.3,40.5729876697063,4.12837641350925));
#73849=CARTESIAN_POINT('Ctrl Pts',(18.18,40.5729876697063,4.12837641350925));
#73850=CARTESIAN_POINT('Ctrl Pts',(18.18,40.5009548604488,4.20477477870882));
#73851=CARTESIAN_POINT('Ctrl Pts',(18.18,40.356889539957,4.22660289369523));
#73852=CARTESIAN_POINT('Ctrl Pts',(18.3,40.6450203299522,3.93738051913679));
#73853=CARTESIAN_POINT('Ctrl Pts',(18.1272,40.6450203299522,3.93738051913679));
#73854=CARTESIAN_POINT('Ctrl Pts',(18.3,40.6450203299522,4.05197804830968));
#73855=CARTESIAN_POINT('Ctrl Pts',(18.1272,40.6450203299522,4.05197804830968));
#73856=CARTESIAN_POINT('Ctrl Pts',(18.3,40.5729876697063,4.12837641350925));
#73857=CARTESIAN_POINT('Ctrl Pts',(18.1272,40.5729876697063,4.12837641350925));
#73858=CARTESIAN_POINT('',(18.3,40.6450203299522,3.93738051913679));
#73859=CARTESIAN_POINT('Ctrl Pts',(18.3,40.6450203299522,3.93738051913679));
#73860=CARTESIAN_POINT('Ctrl Pts',(18.3,40.6450203299522,4.05197804830968));
#73861=CARTESIAN_POINT('Ctrl Pts',(18.3,40.5729876697063,4.12837641350925));
#73862=CARTESIAN_POINT('',(18.18,40.6450203299522,3.93738051913679));
#73863=CARTESIAN_POINT('',(18.3,40.6450203299522,3.93738051913679));
#73864=CARTESIAN_POINT('Ctrl Pts',(18.18,40.6450203299522,3.93738051913679));
#73865=CARTESIAN_POINT('Ctrl Pts',(18.18,40.6450203299522,4.05197804830968));
#73866=CARTESIAN_POINT('Ctrl Pts',(18.18,40.5729876697063,4.12837641350925));
#73867=CARTESIAN_POINT('Ctrl Pts',(18.3,40.5740790307522,3.74856745861471));
#73868=CARTESIAN_POINT('Ctrl Pts',(18.1272,40.5740790307522,3.74856745861471));
#73869=CARTESIAN_POINT('Ctrl Pts',(18.3,40.6450203299522,3.82169162891805));
#73870=CARTESIAN_POINT('Ctrl Pts',(18.1272,40.6450203299522,3.82169162891805));
#73871=CARTESIAN_POINT('Ctrl Pts',(18.3,40.6450203299522,3.93738051913679));
#73872=CARTESIAN_POINT('Ctrl Pts',(18.1272,40.6450203299522,3.93738051913679));
#73873=CARTESIAN_POINT('',(18.3,40.5740790307522,3.74856745861471));
#73874=CARTESIAN_POINT('Ctrl Pts',(18.3,40.5740790307522,3.74856745861471));
#73875=CARTESIAN_POINT('Ctrl Pts',(18.3,40.6450203299522,3.82169162891805));
#73876=CARTESIAN_POINT('Ctrl Pts',(18.3,40.6450203299522,3.93738051913679));
#73877=CARTESIAN_POINT('',(18.18,40.5740790307522,3.74856745861471));
#73878=CARTESIAN_POINT('',(18.3,40.5740790307522,3.74856745861471));
#73879=CARTESIAN_POINT('Ctrl Pts',(18.18,40.5740790307522,3.74856745861471));
#73880=CARTESIAN_POINT('Ctrl Pts',(18.18,40.6450203299522,3.82169162891805));
#73881=CARTESIAN_POINT('Ctrl Pts',(18.18,40.6450203299522,3.93738051913679));
#73882=CARTESIAN_POINT('Ctrl Pts',(18.3,40.3950886666775,3.67544328831136));
#73883=CARTESIAN_POINT('Ctrl Pts',(18.1272,40.3950886666775,3.67544328831136));
#73884=CARTESIAN_POINT('Ctrl Pts',(18.3,40.5031377315521,3.67544328831136));
#73885=CARTESIAN_POINT('Ctrl Pts',(18.1272,40.5031377315521,3.67544328831136));
#73886=CARTESIAN_POINT('Ctrl Pts',(18.3,40.5740790307522,3.74856745861471));
#73887=CARTESIAN_POINT('Ctrl Pts',(18.1272,40.5740790307522,3.74856745861471));
#73888=CARTESIAN_POINT('',(18.3,40.3950886666775,3.67544328831136));
#73889=CARTESIAN_POINT('Ctrl Pts',(18.3,40.3950886666775,3.67544328831136));
#73890=CARTESIAN_POINT('Ctrl Pts',(18.3,40.5031377315521,3.67544328831136));
#73891=CARTESIAN_POINT('Ctrl Pts',(18.3,40.5740790307522,3.74856745861471));
#73892=CARTESIAN_POINT('',(18.18,40.3950886666775,3.67544328831136));
#73893=CARTESIAN_POINT('',(18.3,40.3950886666775,3.67544328831136));
#73894=CARTESIAN_POINT('Ctrl Pts',(18.18,40.3950886666775,3.67544328831136));
#73895=CARTESIAN_POINT('Ctrl Pts',(18.18,40.5031377315521,3.67544328831136));
#73896=CARTESIAN_POINT('Ctrl Pts',(18.18,40.5740790307522,3.74856745861471));
#73897=CARTESIAN_POINT('Ctrl Pts',(18.3,40.1931788265705,3.77585252784193));
#73898=CARTESIAN_POINT('Ctrl Pts',(18.1272,40.1931788265705,3.77585252784193));
#73899=CARTESIAN_POINT('Ctrl Pts',(18.3,40.2586630225181,3.67544328831136));
#73900=CARTESIAN_POINT('Ctrl Pts',(18.1272,40.2586630225181,3.67544328831136));
#73901=CARTESIAN_POINT('Ctrl Pts',(18.3,40.3950886666775,3.67544328831136));
#73902=CARTESIAN_POINT('Ctrl Pts',(18.1272,40.3950886666775,3.67544328831136));
#73903=CARTESIAN_POINT('',(18.3,40.1931788265705,3.77585252784193));
#73904=CARTESIAN_POINT('Ctrl Pts',(18.3,40.1931788265705,3.77585252784193));
#73905=CARTESIAN_POINT('Ctrl Pts',(18.3,40.2586630225181,3.67544328831136));
#73906=CARTESIAN_POINT('Ctrl Pts',(18.3,40.3950886666775,3.67544328831136));
#73907=CARTESIAN_POINT('',(18.18,40.1931788265705,3.77585252784193));
#73908=CARTESIAN_POINT('',(18.3,40.1931788265705,3.77585252784193));
#73909=CARTESIAN_POINT('Ctrl Pts',(18.18,40.1931788265705,3.77585252784193));
#73910=CARTESIAN_POINT('Ctrl Pts',(18.18,40.2586630225181,3.67544328831136));
#73911=CARTESIAN_POINT('Ctrl Pts',(18.18,40.3950886666775,3.67544328831136));
#73912=CARTESIAN_POINT('Ctrl Pts',(18.3,40.1276944816112,4.0017734285444));
#73913=CARTESIAN_POINT('Ctrl Pts',(18.1272,40.1276944816112,4.0017734285444));
#73914=CARTESIAN_POINT('Ctrl Pts',(18.3,40.1276944816112,3.87626184187829));
#73915=CARTESIAN_POINT('Ctrl Pts',(18.1272,40.1276944816112,3.87626184187829));
#73916=CARTESIAN_POINT('Ctrl Pts',(18.3,40.1931788265705,3.77585252784193));
#73917=CARTESIAN_POINT('Ctrl Pts',(18.1272,40.1931788265705,3.77585252784193));
#73918=CARTESIAN_POINT('',(18.3,40.1276944816112,4.0017734285444));
#73919=CARTESIAN_POINT('Ctrl Pts',(18.3,40.1276944816112,4.0017734285444));
#73920=CARTESIAN_POINT('Ctrl Pts',(18.3,40.1276944816112,3.87626184187829));
#73921=CARTESIAN_POINT('Ctrl Pts',(18.3,40.1931788265705,3.77585252784193));
#73922=CARTESIAN_POINT('',(18.18,40.1276944816112,4.0017734285444));
#73923=CARTESIAN_POINT('',(18.3,40.1276944816112,4.0017734285444));
#73924=CARTESIAN_POINT('Ctrl Pts',(18.18,40.1276944816112,4.0017734285444));
#73925=CARTESIAN_POINT('Ctrl Pts',(18.18,40.1276944816112,3.87626184187829));
#73926=CARTESIAN_POINT('Ctrl Pts',(18.18,40.1931788265705,3.77585252784193));
#73927=CARTESIAN_POINT('Ctrl Pts',(18.3,40.1298772037029,4.03342416547239));
#73928=CARTESIAN_POINT('Ctrl Pts',(18.1272,40.1298772037029,4.03342416547239));
#73929=CARTESIAN_POINT('Ctrl Pts',(18.3,40.1276944816112,4.01377884708345));
#73930=CARTESIAN_POINT('Ctrl Pts',(18.1272,40.1276944816112,4.01377884708345));
#73931=CARTESIAN_POINT('Ctrl Pts',(18.3,40.1276944816112,4.0017734285444));
#73932=CARTESIAN_POINT('Ctrl Pts',(18.1272,40.1276944816112,4.0017734285444));
#73933=CARTESIAN_POINT('',(18.3,40.1298772037029,4.03342416547239));
#73934=CARTESIAN_POINT('Ctrl Pts',(18.3,40.1298772037029,4.03342416547239));
#73935=CARTESIAN_POINT('Ctrl Pts',(18.3,40.1276944816112,4.01377884708345));
#73936=CARTESIAN_POINT('Ctrl Pts',(18.3,40.1276944816112,4.0017734285444));
#73937=CARTESIAN_POINT('',(18.18,40.1298772037029,4.03342416547239));
#73938=CARTESIAN_POINT('',(18.3,40.1298772037029,4.03342416547239));
#73939=CARTESIAN_POINT('Ctrl Pts',(18.18,40.1298772037029,4.03342416547239));
#73940=CARTESIAN_POINT('Ctrl Pts',(18.18,40.1276944816112,4.01377884708345));
#73941=CARTESIAN_POINT('Ctrl Pts',(18.18,40.1276944816112,4.0017734285444));
#73942=CARTESIAN_POINT('Origin',(18.3,39.9574353039265,4.05525228045881));
#73943=CARTESIAN_POINT('',(18.3,39.9574353039265,4.05525228045881));
#73944=CARTESIAN_POINT('',(18.3,54.6518279137828,2.19520033276317));
#73945=CARTESIAN_POINT('',(18.18,39.9574353039265,4.05525228045881));
#73946=CARTESIAN_POINT('',(18.3,39.9574353039265,4.05525228045881));
#73947=CARTESIAN_POINT('',(18.18,39.9574353039265,4.05525228045881));
#73948=CARTESIAN_POINT('Ctrl Pts',(18.3,39.9792634189129,3.91664383970201));
#73949=CARTESIAN_POINT('Ctrl Pts',(18.1272,39.9792634189129,3.91664383970201));
#73950=CARTESIAN_POINT('Ctrl Pts',(18.3,39.9792634189129,3.9723054882139));
#73951=CARTESIAN_POINT('Ctrl Pts',(18.1272,39.9792634189129,3.9723054882139));
#73952=CARTESIAN_POINT('Ctrl Pts',(18.3,39.9574353039265,4.05525228045881));
#73953=CARTESIAN_POINT('Ctrl Pts',(18.1272,39.9574353039265,4.05525228045881));
#73954=CARTESIAN_POINT('',(18.3,39.9792634189129,3.91664383970201));
#73955=CARTESIAN_POINT('Ctrl Pts',(18.3,39.9792634189129,3.91664383970201));
#73956=CARTESIAN_POINT('Ctrl Pts',(18.3,39.9792634189129,3.9723054882139));
#73957=CARTESIAN_POINT('Ctrl Pts',(18.3,39.9574353039265,4.05525228045881));
#73958=CARTESIAN_POINT('',(18.18,39.9792634189129,3.91664383970201));
#73959=CARTESIAN_POINT('',(18.3,39.9792634189129,3.91664383970201));
#73960=CARTESIAN_POINT('Ctrl Pts',(18.18,39.9792634189129,3.91664383970201));
#73961=CARTESIAN_POINT('Ctrl Pts',(18.18,39.9792634189129,3.9723054882139));
#73962=CARTESIAN_POINT('Ctrl Pts',(18.18,39.9574353039265,4.05525228045881));
#73963=CARTESIAN_POINT('Ctrl Pts',(18.3,39.8914052784443,3.69181437455118));
#73964=CARTESIAN_POINT('Ctrl Pts',(18.1272,39.8914052784443,3.69181437455118));
#73965=CARTESIAN_POINT('Ctrl Pts',(18.3,39.9792634189129,3.78021819554269));
#73966=CARTESIAN_POINT('Ctrl Pts',(18.1272,39.9792634189129,3.78021819554269));
#73967=CARTESIAN_POINT('Ctrl Pts',(18.3,39.9792634189129,3.91664383970201));
#73968=CARTESIAN_POINT('Ctrl Pts',(18.1272,39.9792634189129,3.91664383970201));
#73969=CARTESIAN_POINT('',(18.3,39.8914052784443,3.69181437455118));
#73970=CARTESIAN_POINT('Ctrl Pts',(18.3,39.8914052784443,3.69181437455118));
#73971=CARTESIAN_POINT('Ctrl Pts',(18.3,39.9792634189129,3.78021819554269));
#73972=CARTESIAN_POINT('Ctrl Pts',(18.3,39.9792634189129,3.91664383970201));
#73973=CARTESIAN_POINT('',(18.18,39.8914052784443,3.69181437455118));
#73974=CARTESIAN_POINT('',(18.3,39.8914052784443,3.69181437455118));
#73975=CARTESIAN_POINT('Ctrl Pts',(18.18,39.8914052784443,3.69181437455118));
#73976=CARTESIAN_POINT('Ctrl Pts',(18.18,39.9792634189129,3.78021819554269));
#73977=CARTESIAN_POINT('Ctrl Pts',(18.18,39.9792634189129,3.91664383970201));
#73978=CARTESIAN_POINT('Ctrl Pts',(18.3,39.6682130038738,3.60341055355966));
#73979=CARTESIAN_POINT('Ctrl Pts',(18.1272,39.6682130038738,3.60341055355966));
#73980=CARTESIAN_POINT('Ctrl Pts',(18.3,39.8035471379757,3.60341055355966));
#73981=CARTESIAN_POINT('Ctrl Pts',(18.1272,39.8035471379757,3.60341055355966));
#73982=CARTESIAN_POINT('Ctrl Pts',(18.3,39.8914052784443,3.69181437455118));
#73983=CARTESIAN_POINT('Ctrl Pts',(18.1272,39.8914052784443,3.69181437455118));
#73984=CARTESIAN_POINT('',(18.3,39.6682130038738,3.60341055355966));
#73985=CARTESIAN_POINT('Ctrl Pts',(18.3,39.6682130038738,3.60341055355966));
#73986=CARTESIAN_POINT('Ctrl Pts',(18.3,39.8035471379757,3.60341055355966));
#73987=CARTESIAN_POINT('Ctrl Pts',(18.3,39.8914052784443,3.69181437455118));
#73988=CARTESIAN_POINT('',(18.18,39.6682130038738,3.60341055355966));
#73989=CARTESIAN_POINT('',(18.3,39.6682130038738,3.60341055355966));
#73990=CARTESIAN_POINT('Ctrl Pts',(18.18,39.6682130038738,3.60341055355966));
#73991=CARTESIAN_POINT('Ctrl Pts',(18.18,39.8035471379757,3.60341055355966));
#73992=CARTESIAN_POINT('Ctrl Pts',(18.18,39.8914052784443,3.69181437455118));
#73993=CARTESIAN_POINT('Ctrl Pts',(18.3,39.4302864611149,3.69890851937234));
#73994=CARTESIAN_POINT('Ctrl Pts',(18.1272,39.4302864611149,3.69890851937234));
#73995=CARTESIAN_POINT('Ctrl Pts',(18.3,39.5263301074505,3.60341055355966));
#73996=CARTESIAN_POINT('Ctrl Pts',(18.1272,39.5263301074505,3.60341055355966));
#73997=CARTESIAN_POINT('Ctrl Pts',(18.3,39.6682130038738,3.60341055355966));
#73998=CARTESIAN_POINT('Ctrl Pts',(18.1272,39.6682130038738,3.60341055355966));
#73999=CARTESIAN_POINT('',(18.3,39.4302864611149,3.69890851937234));
#74000=CARTESIAN_POINT('Ctrl Pts',(18.3,39.4302864611149,3.69890851937234));
#74001=CARTESIAN_POINT('Ctrl Pts',(18.3,39.5263301074505,3.60341055355966));
#74002=CARTESIAN_POINT('Ctrl Pts',(18.3,39.6682130038738,3.60341055355966));
#74003=CARTESIAN_POINT('',(18.18,39.4302864611149,3.69890851937234));
#74004=CARTESIAN_POINT('',(18.3,39.4302864611149,3.69890851937234));
#74005=CARTESIAN_POINT('Ctrl Pts',(18.18,39.4302864611149,3.69890851937234));
#74006=CARTESIAN_POINT('Ctrl Pts',(18.18,39.5263301074505,3.60341055355966));
#74007=CARTESIAN_POINT('Ctrl Pts',(18.18,39.6682130038738,3.60341055355966));
#74008=CARTESIAN_POINT('Ctrl Pts',(18.3,39.3342428147793,3.93301485143602));
#74009=CARTESIAN_POINT('Ctrl Pts',(18.1272,39.3342428147793,3.93301485143602));
#74010=CARTESIAN_POINT('Ctrl Pts',(18.3,39.3342428147793,3.79440641067922));
#74011=CARTESIAN_POINT('Ctrl Pts',(18.1272,39.3342428147793,3.79440641067922));
#74012=CARTESIAN_POINT('Ctrl Pts',(18.3,39.4302864611149,3.69890851937234));
#74013=CARTESIAN_POINT('Ctrl Pts',(18.1272,39.4302864611149,3.69890851937234));
#74014=CARTESIAN_POINT('',(18.3,39.3342428147793,3.93301485143602));
#74015=CARTESIAN_POINT('Ctrl Pts',(18.3,39.3342428147793,3.93301485143602));
#74016=CARTESIAN_POINT('Ctrl Pts',(18.3,39.3342428147793,3.79440641067922));
#74017=CARTESIAN_POINT('Ctrl Pts',(18.3,39.4302864611149,3.69890851937234));
#74018=CARTESIAN_POINT('',(18.18,39.3342428147793,3.93301485143602));
#74019=CARTESIAN_POINT('',(18.3,39.3342428147793,3.93301485143602));
#74020=CARTESIAN_POINT('Ctrl Pts',(18.18,39.3342428147793,3.93301485143602));
#74021=CARTESIAN_POINT('Ctrl Pts',(18.18,39.3342428147793,3.79440641067922));
#74022=CARTESIAN_POINT('Ctrl Pts',(18.18,39.4302864611149,3.69890851937234));
#74023=CARTESIAN_POINT('Ctrl Pts',(18.3,39.4079126656055,4.13110492788255));
#74024=CARTESIAN_POINT('Ctrl Pts',(18.1272,39.4079126656055,4.13110492788255));
#74025=CARTESIAN_POINT('Ctrl Pts',(18.3,39.3342428147793,4.0497952517122));
#74026=CARTESIAN_POINT('Ctrl Pts',(18.1272,39.3342428147793,4.0497952517122));
#74027=CARTESIAN_POINT('Ctrl Pts',(18.3,39.3342428147793,3.93301485143602));
#74028=CARTESIAN_POINT('Ctrl Pts',(18.1272,39.3342428147793,3.93301485143602));
#74029=CARTESIAN_POINT('',(18.3,39.4079126656055,4.13110492788255));
#74030=CARTESIAN_POINT('Ctrl Pts',(18.3,39.4079126656055,4.13110492788255));
#74031=CARTESIAN_POINT('Ctrl Pts',(18.3,39.3342428147793,4.0497952517122));
#74032=CARTESIAN_POINT('Ctrl Pts',(18.3,39.3342428147793,3.93301485143602));
#74033=CARTESIAN_POINT('',(18.18,39.4079126656055,4.13110492788255));
#74034=CARTESIAN_POINT('',(18.3,39.4079126656055,4.13110492788255));
#74035=CARTESIAN_POINT('Ctrl Pts',(18.18,39.4079126656055,4.13110492788255));
#74036=CARTESIAN_POINT('Ctrl Pts',(18.18,39.3342428147793,4.0497952517122));
#74037=CARTESIAN_POINT('Ctrl Pts',(18.18,39.3342428147793,3.93301485143602));
#74038=CARTESIAN_POINT('Ctrl Pts',(18.3,39.6485676109791,4.24624817483127));
#74039=CARTESIAN_POINT('Ctrl Pts',(18.1272,39.6485676109791,4.24624817483127));
#74040=CARTESIAN_POINT('Ctrl Pts',(18.3,39.4815825164318,4.2124146413058));
#74041=CARTESIAN_POINT('Ctrl Pts',(18.1272,39.4815825164318,4.2124146413058));
#74042=CARTESIAN_POINT('Ctrl Pts',(18.3,39.4079126656055,4.13110492788255));
#74043=CARTESIAN_POINT('Ctrl Pts',(18.1272,39.4079126656055,4.13110492788255));
#74044=CARTESIAN_POINT('',(18.3,39.6485676109791,4.24624817483127));
#74045=CARTESIAN_POINT('Ctrl Pts',(18.3,39.6485676109791,4.24624817483127));
#74046=CARTESIAN_POINT('Ctrl Pts',(18.3,39.4815825164318,4.2124146413058));
#74047=CARTESIAN_POINT('Ctrl Pts',(18.3,39.4079126656055,4.13110492788255));
#74048=CARTESIAN_POINT('',(18.18,39.6485676109791,4.24624817483127));
#74049=CARTESIAN_POINT('',(18.3,39.6485676109791,4.24624817483127));
#74050=CARTESIAN_POINT('Ctrl Pts',(18.18,39.6485676109791,4.24624817483127));
#74051=CARTESIAN_POINT('Ctrl Pts',(18.18,39.4815825164318,4.2124146413058));
#74052=CARTESIAN_POINT('Ctrl Pts',(18.18,39.4079126656055,4.13110492788255));
#74053=CARTESIAN_POINT('Origin',(18.3,39.6223737537861,4.44270109795034));
#74054=CARTESIAN_POINT('',(18.3,39.6223737537861,4.44270109795034));
#74055=CARTESIAN_POINT('',(18.3,39.818427473701,2.97230572693353));
#74056=CARTESIAN_POINT('',(18.18,39.6223737537861,4.44270109795034));
#74057=CARTESIAN_POINT('',(18.3,39.6223737537861,4.44270109795034));
#74058=CARTESIAN_POINT('',(18.18,39.6223737537861,4.44270109795034));
#74059=CARTESIAN_POINT('Ctrl Pts',(18.3,39.2971350491047,4.28390165828168));
#74060=CARTESIAN_POINT('Ctrl Pts',(18.1272,39.2971350491047,4.28390165828168));
#74061=CARTESIAN_POINT('Ctrl Pts',(18.3,39.4226466357708,4.4230558168143));
#74062=CARTESIAN_POINT('Ctrl Pts',(18.1272,39.4226466357708,4.4230558168143));
#74063=CARTESIAN_POINT('Ctrl Pts',(18.3,39.6223737537861,4.44270109795034));
#74064=CARTESIAN_POINT('Ctrl Pts',(18.1272,39.6223737537861,4.44270109795034));
#74065=CARTESIAN_POINT('Ctrl Pts',(18.3,39.2971350491047,4.28390165828168));
#74066=CARTESIAN_POINT('Ctrl Pts',(18.3,39.4226466357708,4.4230558168143));
#74067=CARTESIAN_POINT('Ctrl Pts',(18.3,39.6223737537861,4.44270109795034));
#74068=CARTESIAN_POINT('Ctrl Pts',(18.18,39.2971350491047,4.28390165828168));
#74069=CARTESIAN_POINT('Ctrl Pts',(18.18,39.4226466357708,4.4230558168143));
#74070=CARTESIAN_POINT('Ctrl Pts',(18.18,39.6223737537861,4.44270109795034));
#74071=CARTESIAN_POINT('Origin',(18.18,39.9890859663486,3.29999992661178));
#74072=CARTESIAN_POINT('Origin',(18.3,70.,5.5));
#74073=CARTESIAN_POINT('Ctrl Pts',(18.3,30.643929117918,2.64843108169734));
#74074=CARTESIAN_POINT('Ctrl Pts',(18.1272,30.643929117918,2.64843108169734));
#74075=CARTESIAN_POINT('Ctrl Pts',(18.3,30.643929117918,2.78376536481082));
#74076=CARTESIAN_POINT('Ctrl Pts',(18.1272,30.643929117918,2.78376536481082));
#74077=CARTESIAN_POINT('Ctrl Pts',(18.3,30.5293315887451,2.86452936045825));
#74078=CARTESIAN_POINT('Ctrl Pts',(18.1272,30.5293315887451,2.86452936045825));
#74079=CARTESIAN_POINT('',(18.3,30.643929117918,2.64843108169734));
#74080=CARTESIAN_POINT('',(18.3,30.5293315887451,2.86452936045825));
#74081=CARTESIAN_POINT('Ctrl Pts',(18.3,30.643929117918,2.64843108169734));
#74082=CARTESIAN_POINT('Ctrl Pts',(18.3,30.643929117918,2.78376536481082));
#74083=CARTESIAN_POINT('Ctrl Pts',(18.3,30.5293315887451,2.86452936045825));
#74084=CARTESIAN_POINT('',(18.18,30.643929117918,2.64843108169734));
#74085=CARTESIAN_POINT('',(18.3,30.643929117918,2.64843108169734));
#74086=CARTESIAN_POINT('',(18.18,30.5293315887451,2.86452936045825));
#74087=CARTESIAN_POINT('Ctrl Pts',(18.18,30.643929117918,2.64843108169734));
#74088=CARTESIAN_POINT('Ctrl Pts',(18.18,30.643929117918,2.78376536481082));
#74089=CARTESIAN_POINT('Ctrl Pts',(18.18,30.5293315887451,2.86452936045825));
#74090=CARTESIAN_POINT('',(18.3,30.5293315887451,2.86452936045825));
#74091=CARTESIAN_POINT('Ctrl Pts',(18.3,30.514051938057,2.41869034282863));
#74092=CARTESIAN_POINT('Ctrl Pts',(18.1272,30.514051938057,2.41869034282863));
#74093=CARTESIAN_POINT('Ctrl Pts',(18.3,30.643929117918,2.51091407649219));
#74094=CARTESIAN_POINT('Ctrl Pts',(18.1272,30.643929117918,2.51091407649219));
#74095=CARTESIAN_POINT('Ctrl Pts',(18.3,30.643929117918,2.64843108169734));
#74096=CARTESIAN_POINT('Ctrl Pts',(18.1272,30.643929117918,2.64843108169734));
#74097=CARTESIAN_POINT('',(18.3,30.514051938057,2.41869034282863));
#74098=CARTESIAN_POINT('Ctrl Pts',(18.3,30.514051938057,2.41869034282863));
#74099=CARTESIAN_POINT('Ctrl Pts',(18.3,30.643929117918,2.51091407649219));
#74100=CARTESIAN_POINT('Ctrl Pts',(18.3,30.643929117918,2.64843108169734));
#74101=CARTESIAN_POINT('',(18.18,30.514051938057,2.41869034282863));
#74102=CARTESIAN_POINT('',(18.3,30.514051938057,2.41869034282863));
#74103=CARTESIAN_POINT('Ctrl Pts',(18.18,30.514051938057,2.41869034282863));
#74104=CARTESIAN_POINT('Ctrl Pts',(18.18,30.643929117918,2.51091407649219));
#74105=CARTESIAN_POINT('Ctrl Pts',(18.18,30.643929117918,2.64843108169734));
#74106=CARTESIAN_POINT('Ctrl Pts',(18.3,29.9890859663487,2.32646660916507));
#74107=CARTESIAN_POINT('Ctrl Pts',(18.1272,29.9890859663487,2.32646660916507));
#74108=CARTESIAN_POINT('Ctrl Pts',(18.3,30.3841746091843,2.32646660916507));
#74109=CARTESIAN_POINT('Ctrl Pts',(18.1272,30.3841746091843,2.32646660916507));
#74110=CARTESIAN_POINT('Ctrl Pts',(18.3,30.514051938057,2.41869034282863));
#74111=CARTESIAN_POINT('Ctrl Pts',(18.1272,30.514051938057,2.41869034282863));
#74112=CARTESIAN_POINT('',(18.3,29.9890859663487,2.32646660916507));
#74113=CARTESIAN_POINT('Ctrl Pts',(18.3,29.9890859663487,2.32646660916507));
#74114=CARTESIAN_POINT('Ctrl Pts',(18.3,30.3841746091843,2.32646660916507));
#74115=CARTESIAN_POINT('Ctrl Pts',(18.3,30.514051938057,2.41869034282863));
#74116=CARTESIAN_POINT('',(18.18,29.9890859663487,2.32646660916507));
#74117=CARTESIAN_POINT('',(18.3,29.9890859663487,2.32646660916507));
#74118=CARTESIAN_POINT('Ctrl Pts',(18.18,29.9890859663487,2.32646660916507));
#74119=CARTESIAN_POINT('Ctrl Pts',(18.18,30.3841746091843,2.32646660916507));
#74120=CARTESIAN_POINT('Ctrl Pts',(18.18,30.514051938057,2.41869034282863));
#74121=CARTESIAN_POINT('Ctrl Pts',(18.3,29.4652115046978,2.41869034282863));
#74122=CARTESIAN_POINT('Ctrl Pts',(18.1272,29.4652115046978,2.41869034282863));
#74123=CARTESIAN_POINT('Ctrl Pts',(18.3,29.5961801946163,2.32646660916507));
#74124=CARTESIAN_POINT('Ctrl Pts',(18.1272,29.5961801946163,2.32646660916507));
#74125=CARTESIAN_POINT('Ctrl Pts',(18.3,29.9890859663487,2.32646660916507));
#74126=CARTESIAN_POINT('Ctrl Pts',(18.1272,29.9890859663487,2.32646660916507));
#74127=CARTESIAN_POINT('',(18.3,29.4652115046978,2.41869034282863));
#74128=CARTESIAN_POINT('Ctrl Pts',(18.3,29.4652115046978,2.41869034282863));
#74129=CARTESIAN_POINT('Ctrl Pts',(18.3,29.5961801946163,2.32646660916507));
#74130=CARTESIAN_POINT('Ctrl Pts',(18.3,29.9890859663487,2.32646660916507));
#74131=CARTESIAN_POINT('',(18.18,29.4652115046978,2.41869034282863));
#74132=CARTESIAN_POINT('',(18.3,29.4652115046978,2.41869034282863));
#74133=CARTESIAN_POINT('Ctrl Pts',(18.18,29.4652115046978,2.41869034282863));
#74134=CARTESIAN_POINT('Ctrl Pts',(18.18,29.5961801946163,2.32646660916507));
#74135=CARTESIAN_POINT('Ctrl Pts',(18.18,29.9890859663487,2.32646660916507));
#74136=CARTESIAN_POINT('Ctrl Pts',(18.3,29.3342428147793,2.64624821059406));
#74137=CARTESIAN_POINT('Ctrl Pts',(18.1272,29.3342428147793,2.64624821059406));
#74138=CARTESIAN_POINT('Ctrl Pts',(18.3,29.3342428147793,2.51091407649219));
#74139=CARTESIAN_POINT('Ctrl Pts',(18.1272,29.3342428147793,2.51091407649219));
#74140=CARTESIAN_POINT('Ctrl Pts',(18.3,29.4652115046978,2.41869034282863));
#74141=CARTESIAN_POINT('Ctrl Pts',(18.1272,29.4652115046978,2.41869034282863));
#74142=CARTESIAN_POINT('',(18.3,29.3342428147793,2.64624821059406));
#74143=CARTESIAN_POINT('Ctrl Pts',(18.3,29.3342428147793,2.64624821059406));
#74144=CARTESIAN_POINT('Ctrl Pts',(18.3,29.3342428147793,2.51091407649219));
#74145=CARTESIAN_POINT('Ctrl Pts',(18.3,29.4652115046978,2.41869034282863));
#74146=CARTESIAN_POINT('',(18.18,29.3342428147793,2.64624821059406));
#74147=CARTESIAN_POINT('',(18.3,29.3342428147793,2.64624821059406));
#74148=CARTESIAN_POINT('Ctrl Pts',(18.18,29.3342428147793,2.64624821059406));
#74149=CARTESIAN_POINT('Ctrl Pts',(18.18,29.3342428147793,2.51091407649219));
#74150=CARTESIAN_POINT('Ctrl Pts',(18.18,29.4652115046978,2.41869034282863));
#74151=CARTESIAN_POINT('Ctrl Pts',(18.3,29.4646658241749,2.8738062273711));
#74152=CARTESIAN_POINT('Ctrl Pts',(18.1272,29.4646658241749,2.8738062273711));
#74153=CARTESIAN_POINT('Ctrl Pts',(18.3,29.3342428147793,2.78158249370754));
#74154=CARTESIAN_POINT('Ctrl Pts',(18.1272,29.3342428147793,2.78158249370754));
#74155=CARTESIAN_POINT('Ctrl Pts',(18.3,29.3342428147793,2.64624821059406));
#74156=CARTESIAN_POINT('Ctrl Pts',(18.1272,29.3342428147793,2.64624821059406));
#74157=CARTESIAN_POINT('',(18.3,29.4646658241749,2.8738062273711));
#74158=CARTESIAN_POINT('Ctrl Pts',(18.3,29.4646658241749,2.8738062273711));
#74159=CARTESIAN_POINT('Ctrl Pts',(18.3,29.3342428147793,2.78158249370754));
#74160=CARTESIAN_POINT('Ctrl Pts',(18.3,29.3342428147793,2.64624821059406));
#74161=CARTESIAN_POINT('',(18.18,29.4646658241749,2.8738062273711));
#74162=CARTESIAN_POINT('',(18.3,29.4646658241749,2.8738062273711));
#74163=CARTESIAN_POINT('Ctrl Pts',(18.18,29.4646658241749,2.8738062273711));
#74164=CARTESIAN_POINT('Ctrl Pts',(18.18,29.3342428147793,2.78158249370754));
#74165=CARTESIAN_POINT('Ctrl Pts',(18.18,29.3342428147793,2.64624821059406));
#74166=CARTESIAN_POINT('Ctrl Pts',(18.3,29.9890859663487,2.96602996103466));
#74167=CARTESIAN_POINT('Ctrl Pts',(18.1272,29.9890859663487,2.96602996103466));
#74168=CARTESIAN_POINT('Ctrl Pts',(18.3,29.5950888335705,2.96602996103466));
#74169=CARTESIAN_POINT('Ctrl Pts',(18.1272,29.5950888335705,2.96602996103466));
#74170=CARTESIAN_POINT('Ctrl Pts',(18.3,29.4646658241749,2.8738062273711));
#74171=CARTESIAN_POINT('Ctrl Pts',(18.1272,29.4646658241749,2.8738062273711));
#74172=CARTESIAN_POINT('',(18.3,29.9890859663487,2.96602996103466));
#74173=CARTESIAN_POINT('Ctrl Pts',(18.3,29.9890859663487,2.96602996103466));
#74174=CARTESIAN_POINT('Ctrl Pts',(18.3,29.5950888335705,2.96602996103466));
#74175=CARTESIAN_POINT('Ctrl Pts',(18.3,29.4646658241749,2.8738062273711));
#74176=CARTESIAN_POINT('',(18.18,29.9890859663487,2.96602996103466));
#74177=CARTESIAN_POINT('',(18.3,29.9890859663487,2.96602996103466));
#74178=CARTESIAN_POINT('Ctrl Pts',(18.18,29.9890859663487,2.96602996103466));
#74179=CARTESIAN_POINT('Ctrl Pts',(18.18,29.5950888335705,2.96602996103466));
#74180=CARTESIAN_POINT('Ctrl Pts',(18.18,29.4646658241749,2.8738062273711));
#74181=CARTESIAN_POINT('Ctrl Pts',(18.3,30.5293315887451,2.86452936045825));
#74182=CARTESIAN_POINT('Ctrl Pts',(18.1272,30.5293315887451,2.86452936045825));
#74183=CARTESIAN_POINT('Ctrl Pts',(18.3,30.3830830991268,2.96602996103466));
#74184=CARTESIAN_POINT('Ctrl Pts',(18.1272,30.3830830991268,2.96602996103466));
#74185=CARTESIAN_POINT('Ctrl Pts',(18.3,29.9890859663487,2.96602996103466));
#74186=CARTESIAN_POINT('Ctrl Pts',(18.1272,29.9890859663487,2.96602996103466));
#74187=CARTESIAN_POINT('Ctrl Pts',(18.3,30.5293315887451,2.86452936045825));
#74188=CARTESIAN_POINT('Ctrl Pts',(18.3,30.3830830991268,2.96602996103466));
#74189=CARTESIAN_POINT('Ctrl Pts',(18.3,29.9890859663487,2.96602996103466));
#74190=CARTESIAN_POINT('Ctrl Pts',(18.18,30.5293315887451,2.86452936045825));
#74191=CARTESIAN_POINT('Ctrl Pts',(18.18,30.3830830991268,2.96602996103466));
#74192=CARTESIAN_POINT('Ctrl Pts',(18.18,29.9890859663487,2.96602996103466));
#74193=CARTESIAN_POINT('Ctrl Pts',(18.3,29.1727148234844,2.64624821059406));
#74194=CARTESIAN_POINT('Ctrl Pts',(18.1272,29.1727148234844,2.64624821059406));
#74195=CARTESIAN_POINT('Ctrl Pts',(18.3,29.1727148234844,2.87762614004314));
#74196=CARTESIAN_POINT('Ctrl Pts',(18.1272,29.1727148234844,2.87762614004314));
#74197=CARTESIAN_POINT('Ctrl Pts',(18.3,29.3386085569859,3.00968619100749));
#74198=CARTESIAN_POINT('Ctrl Pts',(18.1272,29.3386085569859,3.00968619100749));
#74199=CARTESIAN_POINT('',(18.3,29.1727148234844,2.64624821059406));
#74200=CARTESIAN_POINT('',(18.3,29.3386085569859,3.00968619100749));
#74201=CARTESIAN_POINT('Ctrl Pts',(18.3,29.1727148234844,2.64624821059406));
#74202=CARTESIAN_POINT('Ctrl Pts',(18.3,29.1727148234844,2.87762614004314));
#74203=CARTESIAN_POINT('Ctrl Pts',(18.3,29.3386085569859,3.00968619100749));
#74204=CARTESIAN_POINT('',(18.18,29.1727148234844,2.64624821059406));
#74205=CARTESIAN_POINT('',(18.3,29.1727148234844,2.64624821059406));
#74206=CARTESIAN_POINT('',(18.18,29.3386085569859,3.00968619100749));
#74207=CARTESIAN_POINT('Ctrl Pts',(18.18,29.1727148234844,2.64624821059406));
#74208=CARTESIAN_POINT('Ctrl Pts',(18.18,29.1727148234844,2.87762614004314));
#74209=CARTESIAN_POINT('Ctrl Pts',(18.18,29.3386085569859,3.00968619100749));
#74210=CARTESIAN_POINT('',(18.3,29.3386085569859,3.00968619100749));
#74211=CARTESIAN_POINT('Ctrl Pts',(18.3,29.2671214282513,2.35538886897266));
#74212=CARTESIAN_POINT('Ctrl Pts',(18.1272,29.2671214282513,2.35538886897266));
#74213=CARTESIAN_POINT('Ctrl Pts',(18.3,29.1727148234844,2.47053207866847));
#74214=CARTESIAN_POINT('Ctrl Pts',(18.1272,29.1727148234844,2.47053207866847));
#74215=CARTESIAN_POINT('Ctrl Pts',(18.3,29.1727148234844,2.64624821059406));
#74216=CARTESIAN_POINT('Ctrl Pts',(18.1272,29.1727148234844,2.64624821059406));
#74217=CARTESIAN_POINT('',(18.3,29.2671214282513,2.35538886897266));
#74218=CARTESIAN_POINT('Ctrl Pts',(18.3,29.2671214282513,2.35538886897266));
#74219=CARTESIAN_POINT('Ctrl Pts',(18.3,29.1727148234844,2.47053207866847));
#74220=CARTESIAN_POINT('Ctrl Pts',(18.3,29.1727148234844,2.64624821059406));
#74221=CARTESIAN_POINT('',(18.18,29.2671214282513,2.35538886897266));
#74222=CARTESIAN_POINT('',(18.3,29.2671214282513,2.35538886897266));
#74223=CARTESIAN_POINT('Ctrl Pts',(18.18,29.2671214282513,2.35538886897266));
#74224=CARTESIAN_POINT('Ctrl Pts',(18.18,29.1727148234844,2.47053207866847));
#74225=CARTESIAN_POINT('Ctrl Pts',(18.18,29.1727148234844,2.64624821059406));
#74226=CARTESIAN_POINT('Ctrl Pts',(18.3,29.5345156133175,2.18240113966167));
#74227=CARTESIAN_POINT('Ctrl Pts',(18.1272,29.5345156133175,2.18240113966167));
#74228=CARTESIAN_POINT('Ctrl Pts',(18.3,29.3615280330181,2.24024551026523));
#74229=CARTESIAN_POINT('Ctrl Pts',(18.1272,29.3615280330181,2.24024551026523));
#74230=CARTESIAN_POINT('Ctrl Pts',(18.3,29.2671214282513,2.35538886897266));
#74231=CARTESIAN_POINT('Ctrl Pts',(18.1272,29.2671214282513,2.35538886897266));
#74232=CARTESIAN_POINT('',(18.3,29.5345156133175,2.18240113966167));
#74233=CARTESIAN_POINT('Ctrl Pts',(18.3,29.5345156133175,2.18240113966167));
#74234=CARTESIAN_POINT('Ctrl Pts',(18.3,29.3615280330181,2.24024551026523));
#74235=CARTESIAN_POINT('Ctrl Pts',(18.3,29.2671214282513,2.35538886897266));
#74236=CARTESIAN_POINT('',(18.18,29.5345156133175,2.18240113966167));
#74237=CARTESIAN_POINT('',(18.3,29.5345156133175,2.18240113966167));
#74238=CARTESIAN_POINT('Ctrl Pts',(18.18,29.5345156133175,2.18240113966167));
#74239=CARTESIAN_POINT('Ctrl Pts',(18.18,29.3615280330181,2.24024551026523));
#74240=CARTESIAN_POINT('Ctrl Pts',(18.18,29.2671214282513,2.35538886897266));
#74241=CARTESIAN_POINT('Ctrl Pts',(18.3,29.9890859663487,2.12455647103488));
#74242=CARTESIAN_POINT('Ctrl Pts',(18.1272,29.9890859663487,2.12455647103488));
#74243=CARTESIAN_POINT('Ctrl Pts',(18.3,29.7075034916401,2.12455647103488));
#74244=CARTESIAN_POINT('Ctrl Pts',(18.1272,29.7075034916401,2.12455647103488));
#74245=CARTESIAN_POINT('Ctrl Pts',(18.3,29.5345156133175,2.18240113966167));
#74246=CARTESIAN_POINT('Ctrl Pts',(18.1272,29.5345156133175,2.18240113966167));
#74247=CARTESIAN_POINT('',(18.3,29.9890859663487,2.12455647103488));
#74248=CARTESIAN_POINT('Ctrl Pts',(18.3,29.9890859663487,2.12455647103488));
#74249=CARTESIAN_POINT('Ctrl Pts',(18.3,29.7075034916401,2.12455647103488));
#74250=CARTESIAN_POINT('Ctrl Pts',(18.3,29.5345156133175,2.18240113966167));
#74251=CARTESIAN_POINT('',(18.18,29.9890859663487,2.12455647103488));
#74252=CARTESIAN_POINT('',(18.3,29.9890859663487,2.12455647103488));
#74253=CARTESIAN_POINT('Ctrl Pts',(18.18,29.9890859663487,2.12455647103488));
#74254=CARTESIAN_POINT('Ctrl Pts',(18.18,29.7075034916401,2.12455647103488));
#74255=CARTESIAN_POINT('Ctrl Pts',(18.18,29.5345156133175,2.18240113966167));
#74256=CARTESIAN_POINT('Ctrl Pts',(18.3,30.3672577679157,2.16057302467525));
#74257=CARTESIAN_POINT('Ctrl Pts',(18.1272,30.3672577679157,2.16057302467525));
#74258=CARTESIAN_POINT('Ctrl Pts',(18.3,30.2270122110844,2.12455647103488));
#74259=CARTESIAN_POINT('Ctrl Pts',(18.1272,30.2270122110844,2.12455647103488));
#74260=CARTESIAN_POINT('Ctrl Pts',(18.3,29.9890859663487,2.12455647103488));
#74261=CARTESIAN_POINT('Ctrl Pts',(18.1272,29.9890859663487,2.12455647103488));
#74262=CARTESIAN_POINT('',(18.3,30.3672577679157,2.16057302467525));
#74263=CARTESIAN_POINT('Ctrl Pts',(18.3,30.3672577679157,2.16057302467525));
#74264=CARTESIAN_POINT('Ctrl Pts',(18.3,30.2270122110844,2.12455647103488));
#74265=CARTESIAN_POINT('Ctrl Pts',(18.3,29.9890859663487,2.12455647103488));
#74266=CARTESIAN_POINT('',(18.18,30.3672577679157,2.16057302467525));
#74267=CARTESIAN_POINT('',(18.3,30.3672577679157,2.16057302467525));
#74268=CARTESIAN_POINT('Ctrl Pts',(18.18,30.3672577679157,2.16057302467525));
#74269=CARTESIAN_POINT('Ctrl Pts',(18.18,30.2270122110844,2.12455647103488));
#74270=CARTESIAN_POINT('Ctrl Pts',(18.18,29.9890859663487,2.12455647103488));
#74271=CARTESIAN_POINT('Ctrl Pts',(18.3,30.6051841616631,2.25989090315998));
#74272=CARTESIAN_POINT('Ctrl Pts',(18.1272,30.6051841616631,2.25989090315998));
#74273=CARTESIAN_POINT('Ctrl Pts',(18.3,30.5075034737587,2.19658928029239));
#74274=CARTESIAN_POINT('Ctrl Pts',(18.1272,30.5075034737587,2.19658928029239));
#74275=CARTESIAN_POINT('Ctrl Pts',(18.3,30.3672577679157,2.16057302467525));
#74276=CARTESIAN_POINT('Ctrl Pts',(18.1272,30.3672577679157,2.16057302467525));
#74277=CARTESIAN_POINT('',(18.3,30.6051841616631,2.25989090315998));
#74278=CARTESIAN_POINT('Ctrl Pts',(18.3,30.6051841616631,2.25989090315998));
#74279=CARTESIAN_POINT('Ctrl Pts',(18.3,30.5075034737587,2.19658928029239));
#74280=CARTESIAN_POINT('Ctrl Pts',(18.3,30.3672577679157,2.16057302467525));
#74281=CARTESIAN_POINT('',(18.18,30.6051841616631,2.25989090315998));
#74282=CARTESIAN_POINT('',(18.3,30.6051841616631,2.25989090315998));
#74283=CARTESIAN_POINT('Ctrl Pts',(18.18,30.6051841616631,2.25989090315998));
#74284=CARTESIAN_POINT('Ctrl Pts',(18.18,30.5075034737587,2.19658928029239));
#74285=CARTESIAN_POINT('Ctrl Pts',(18.18,30.3672577679157,2.16057302467525));
#74286=CARTESIAN_POINT('Ctrl Pts',(18.3,30.7547067344189,2.420327533409));
#74287=CARTESIAN_POINT('Ctrl Pts',(18.1272,30.7547067344189,2.420327533409));
#74288=CARTESIAN_POINT('Ctrl Pts',(18.3,30.702864998579,2.32319237701595));
#74289=CARTESIAN_POINT('Ctrl Pts',(18.1272,30.702864998579,2.32319237701595));
#74290=CARTESIAN_POINT('Ctrl Pts',(18.3,30.6051841616631,2.25989090315998));
#74291=CARTESIAN_POINT('Ctrl Pts',(18.1272,30.6051841616631,2.25989090315998));
#74292=CARTESIAN_POINT('',(18.3,30.7547067344189,2.420327533409));
#74293=CARTESIAN_POINT('Ctrl Pts',(18.3,30.7547067344189,2.420327533409));
#74294=CARTESIAN_POINT('Ctrl Pts',(18.3,30.702864998579,2.32319237701595));
#74295=CARTESIAN_POINT('Ctrl Pts',(18.3,30.6051841616631,2.25989090315998));
#74296=CARTESIAN_POINT('',(18.18,30.7547067344189,2.420327533409));
#74297=CARTESIAN_POINT('',(18.3,30.7547067344189,2.420327533409));
#74298=CARTESIAN_POINT('Ctrl Pts',(18.18,30.7547067344189,2.420327533409));
#74299=CARTESIAN_POINT('Ctrl Pts',(18.18,30.702864998579,2.32319237701595));
#74300=CARTESIAN_POINT('Ctrl Pts',(18.18,30.6051841616631,2.25989090315998));
#74301=CARTESIAN_POINT('Ctrl Pts',(18.3,30.8065484702587,2.64624821059406));
#74302=CARTESIAN_POINT('Ctrl Pts',(18.1272,30.8065484702587,2.64624821059406));
#74303=CARTESIAN_POINT('Ctrl Pts',(18.3,30.8065484702587,2.51746254079044));
#74304=CARTESIAN_POINT('Ctrl Pts',(18.1272,30.8065484702587,2.51746254079044));
#74305=CARTESIAN_POINT('Ctrl Pts',(18.3,30.7547067344189,2.420327533409));
#74306=CARTESIAN_POINT('Ctrl Pts',(18.1272,30.7547067344189,2.420327533409));
#74307=CARTESIAN_POINT('',(18.3,30.8065484702587,2.64624821059406));
#74308=CARTESIAN_POINT('Ctrl Pts',(18.3,30.8065484702587,2.64624821059406));
#74309=CARTESIAN_POINT('Ctrl Pts',(18.3,30.8065484702587,2.51746254079044));
#74310=CARTESIAN_POINT('Ctrl Pts',(18.3,30.7547067344189,2.420327533409));
#74311=CARTESIAN_POINT('',(18.18,30.8065484702587,2.64624821059406));
#74312=CARTESIAN_POINT('',(18.3,30.8065484702587,2.64624821059406));
#74313=CARTESIAN_POINT('Ctrl Pts',(18.18,30.8065484702587,2.64624821059406));
#74314=CARTESIAN_POINT('Ctrl Pts',(18.18,30.8065484702587,2.51746254079044));
#74315=CARTESIAN_POINT('Ctrl Pts',(18.18,30.7547067344189,2.420327533409));
#74316=CARTESIAN_POINT('Ctrl Pts',(18.3,30.7126876950264,2.93601634018123));
#74317=CARTESIAN_POINT('Ctrl Pts',(18.1272,30.7126876950264,2.93601634018123));
#74318=CARTESIAN_POINT('Ctrl Pts',(18.3,30.8065484702587,2.82087313048542));
#74319=CARTESIAN_POINT('Ctrl Pts',(18.1272,30.8065484702587,2.82087313048542));
#74320=CARTESIAN_POINT('Ctrl Pts',(18.3,30.8065484702587,2.64624821059406));
#74321=CARTESIAN_POINT('Ctrl Pts',(18.1272,30.8065484702587,2.64624821059406));
#74322=CARTESIAN_POINT('',(18.3,30.7126876950264,2.93601634018123));
#74323=CARTESIAN_POINT('Ctrl Pts',(18.3,30.7126876950264,2.93601634018123));
#74324=CARTESIAN_POINT('Ctrl Pts',(18.3,30.8065484702587,2.82087313048542));
#74325=CARTESIAN_POINT('Ctrl Pts',(18.3,30.8065484702587,2.64624821059406));
#74326=CARTESIAN_POINT('',(18.18,30.7126876950264,2.93601634018123));
#74327=CARTESIAN_POINT('',(18.3,30.7126876950264,2.93601634018123));
#74328=CARTESIAN_POINT('Ctrl Pts',(18.18,30.7126876950264,2.93601634018123));
#74329=CARTESIAN_POINT('Ctrl Pts',(18.18,30.8065484702587,2.82087313048542));
#74330=CARTESIAN_POINT('Ctrl Pts',(18.18,30.8065484702587,2.64624821059406));
#74331=CARTESIAN_POINT('Ctrl Pts',(18.3,30.4458390414715,3.10954975001514));
#74332=CARTESIAN_POINT('Ctrl Pts',(18.1272,30.4458390414715,3.10954975001514));
#74333=CARTESIAN_POINT('Ctrl Pts',(18.3,30.6188267707825,3.05115954987705));
#74334=CARTESIAN_POINT('Ctrl Pts',(18.1272,30.6188267707825,3.05115954987705));
#74335=CARTESIAN_POINT('Ctrl Pts',(18.3,30.7126876950264,2.93601634018123));
#74336=CARTESIAN_POINT('Ctrl Pts',(18.1272,30.7126876950264,2.93601634018123));
#74337=CARTESIAN_POINT('',(18.3,30.4458390414715,3.10954975001514));
#74338=CARTESIAN_POINT('Ctrl Pts',(18.3,30.4458390414715,3.10954975001514));
#74339=CARTESIAN_POINT('Ctrl Pts',(18.3,30.6188267707825,3.05115954987705));
#74340=CARTESIAN_POINT('Ctrl Pts',(18.3,30.7126876950264,2.93601634018123));
#74341=CARTESIAN_POINT('',(18.18,30.4458390414715,3.10954975001514));
#74342=CARTESIAN_POINT('',(18.3,30.4458390414715,3.10954975001514));
#74343=CARTESIAN_POINT('Ctrl Pts',(18.18,30.4458390414715,3.10954975001514));
#74344=CARTESIAN_POINT('Ctrl Pts',(18.18,30.6188267707825,3.05115954987705));
#74345=CARTESIAN_POINT('Ctrl Pts',(18.18,30.7126876950264,2.93601634018123));
#74346=CARTESIAN_POINT('Ctrl Pts',(18.3,29.9890859663487,3.16793995015323));
#74347=CARTESIAN_POINT('Ctrl Pts',(18.1272,29.9890859663487,3.16793995015323));
#74348=CARTESIAN_POINT('Ctrl Pts',(18.3,30.2728513121605,3.16793995015323));
#74349=CARTESIAN_POINT('Ctrl Pts',(18.1272,30.2728513121605,3.16793995015323));
#74350=CARTESIAN_POINT('Ctrl Pts',(18.3,30.4458390414715,3.10954975001514));
#74351=CARTESIAN_POINT('Ctrl Pts',(18.1272,30.4458390414715,3.10954975001514));
#74352=CARTESIAN_POINT('',(18.3,29.9890859663487,3.16793995015323));
#74353=CARTESIAN_POINT('Ctrl Pts',(18.3,29.9890859663487,3.16793995015323));
#74354=CARTESIAN_POINT('Ctrl Pts',(18.3,30.2728513121605,3.16793995015323));
#74355=CARTESIAN_POINT('Ctrl Pts',(18.3,30.4458390414715,3.10954975001514));
#74356=CARTESIAN_POINT('',(18.18,29.9890859663487,3.16793995015323));
#74357=CARTESIAN_POINT('',(18.3,29.9890859663487,3.16793995015323));
#74358=CARTESIAN_POINT('Ctrl Pts',(18.18,29.9890859663487,3.16793995015323));
#74359=CARTESIAN_POINT('Ctrl Pts',(18.18,30.2728513121605,3.16793995015323));
#74360=CARTESIAN_POINT('Ctrl Pts',(18.18,30.4458390414715,3.10954975001514));
#74361=CARTESIAN_POINT('Ctrl Pts',(18.3,29.3386085569859,3.00968619100749));
#74362=CARTESIAN_POINT('Ctrl Pts',(18.1272,29.3386085569859,3.00968619100749));
#74363=CARTESIAN_POINT('Ctrl Pts',(18.3,29.5383356750012,3.16793995015323));
#74364=CARTESIAN_POINT('Ctrl Pts',(18.1272,29.5383356750012,3.16793995015323));
#74365=CARTESIAN_POINT('Ctrl Pts',(18.3,29.9890859663487,3.16793995015323));
#74366=CARTESIAN_POINT('Ctrl Pts',(18.1272,29.9890859663487,3.16793995015323));
#74367=CARTESIAN_POINT('Ctrl Pts',(18.3,29.3386085569859,3.00968619100749));
#74368=CARTESIAN_POINT('Ctrl Pts',(18.3,29.5383356750012,3.16793995015323));
#74369=CARTESIAN_POINT('Ctrl Pts',(18.3,29.9890859663487,3.16793995015323));
#74370=CARTESIAN_POINT('Ctrl Pts',(18.18,29.3386085569859,3.00968619100749));
#74371=CARTESIAN_POINT('Ctrl Pts',(18.18,29.5383356750012,3.16793995015323));
#74372=CARTESIAN_POINT('Ctrl Pts',(18.18,29.9890859663487,3.16793995015323));
#74373=CARTESIAN_POINT('Origin',(18.18,29.9896316468716,3.29999987538904));
#74374=CARTESIAN_POINT('Origin',(18.3,30.4845838487148,3.78130966834724));
#74375=CARTESIAN_POINT('',(18.3,30.4845838487148,3.78130966834724));
#74376=CARTESIAN_POINT('',(18.3,29.7631649911404,4.28226457946002));
#74377=CARTESIAN_POINT('',(18.3,43.4120209624511,-5.19553234546084));
#74378=CARTESIAN_POINT('',(18.18,30.4845838487148,3.78130966834724));
#74379=CARTESIAN_POINT('',(18.3,30.4845838487148,3.78130966834724));
#74380=CARTESIAN_POINT('',(18.18,29.7631649911404,4.28226457946002));
#74381=CARTESIAN_POINT('',(18.18,30.4845838487148,3.78130966834724));
#74382=CARTESIAN_POINT('',(18.3,29.7631649911404,4.28226457946002));
#74383=CARTESIAN_POINT('Origin',(18.3,29.7631649911404,3.78130966834724));
#74384=CARTESIAN_POINT('',(18.3,29.7631649911404,3.78130966834724));
#74385=CARTESIAN_POINT('',(18.3,49.8815824955702,3.78130966834724));
#74386=CARTESIAN_POINT('',(18.18,29.7631649911404,3.78130966834724));
#74387=CARTESIAN_POINT('',(18.3,29.7631649911404,3.78130966834724));
#74388=CARTESIAN_POINT('',(18.18,29.7631649911404,3.78130966834724));
#74389=CARTESIAN_POINT('Origin',(18.3,29.7631649911404,4.28226457946002));
#74390=CARTESIAN_POINT('',(18.3,29.7631649911404,4.89113228973001));
#74391=CARTESIAN_POINT('',(18.18,29.7631649911404,4.28226457946002));
#74392=CARTESIAN_POINT('Origin',(18.3,29.5830832660198,3.58485670797527));
#74393=CARTESIAN_POINT('',(18.3,29.5830832660198,3.58485670797527));
#74394=CARTESIAN_POINT('',(18.3,29.2000000417233,3.58485670797527));
#74395=CARTESIAN_POINT('',(18.3,49.7915416330099,3.58485670797527));
#74396=CARTESIAN_POINT('',(18.18,29.5830832660198,3.58485670797527));
#74397=CARTESIAN_POINT('',(18.3,29.5830832660198,3.58485670797527));
#74398=CARTESIAN_POINT('',(18.18,29.2000000417233,3.58485670797527));
#74399=CARTESIAN_POINT('',(18.18,29.5830832660198,3.58485670797527));
#74400=CARTESIAN_POINT('',(18.3,29.2000000417233,3.58485670797527));
#74401=CARTESIAN_POINT('Origin',(18.3,29.5830832660198,3.36875842921436));
#74402=CARTESIAN_POINT('',(18.3,29.5830832660198,3.36875842921436));
#74403=CARTESIAN_POINT('',(18.3,29.5830832660198,4.43437921460718));
#74404=CARTESIAN_POINT('',(18.18,29.5830832660198,3.36875842921436));
#74405=CARTESIAN_POINT('',(18.3,29.5830832660198,3.36875842921436));
#74406=CARTESIAN_POINT('',(18.18,29.5830832660198,3.36875842921436));
#74407=CARTESIAN_POINT('Origin',(18.3,29.7631649911404,3.36875842921436));
#74408=CARTESIAN_POINT('',(18.3,29.7631649911404,3.36875842921436));
#74409=CARTESIAN_POINT('',(18.3,49.8815824955702,3.36875842921436));
#74410=CARTESIAN_POINT('',(18.18,29.7631649911404,3.36875842921436));
#74411=CARTESIAN_POINT('',(18.3,29.7631649911404,3.36875842921436));
#74412=CARTESIAN_POINT('',(18.18,29.7631649911404,3.36875842921436));
#74413=CARTESIAN_POINT('Origin',(18.3,29.7631649911404,3.58485670797527));
#74414=CARTESIAN_POINT('',(18.3,29.7631649911404,3.58485670797527));
#74415=CARTESIAN_POINT('',(18.3,29.7631649911404,4.54242835398763));
#74416=CARTESIAN_POINT('',(18.18,29.7631649911404,3.58485670797527));
#74417=CARTESIAN_POINT('',(18.3,29.7631649911404,3.58485670797527));
#74418=CARTESIAN_POINT('',(18.18,29.7631649911404,3.58485670797527));
#74419=CARTESIAN_POINT('Origin',(18.3,30.8000000059605,3.58485670797527));
#74420=CARTESIAN_POINT('',(18.3,30.8000000059605,3.58485670797527));
#74421=CARTESIAN_POINT('',(18.3,50.4000000029802,3.58485670797527));
#74422=CARTESIAN_POINT('',(18.18,30.8000000059605,3.58485670797527));
#74423=CARTESIAN_POINT('',(18.3,30.8000000059605,3.58485670797527));
#74424=CARTESIAN_POINT('',(18.18,30.8000000059605,3.58485670797527));
#74425=CARTESIAN_POINT('Origin',(18.3,30.8000000059605,3.74529326371849));
#74426=CARTESIAN_POINT('',(18.3,30.8000000059605,3.74529326371849));
#74427=CARTESIAN_POINT('',(18.3,30.8000000059605,4.62264663185924));
#74428=CARTESIAN_POINT('',(18.18,30.8000000059605,3.74529326371849));
#74429=CARTESIAN_POINT('',(18.3,30.8000000059605,3.74529326371849));
#74430=CARTESIAN_POINT('',(18.18,30.8000000059605,3.74529326371849));
#74431=CARTESIAN_POINT('Origin',(18.3,29.7631649911404,4.47544327974319));
#74432=CARTESIAN_POINT('',(18.3,29.7631649911404,4.47544327974319));
#74433=CARTESIAN_POINT('',(18.3,42.9709350156429,-4.8256059298212));
#74434=CARTESIAN_POINT('',(18.18,29.7631649911404,4.47544327974319));
#74435=CARTESIAN_POINT('',(18.3,29.7631649911404,4.47544327974319));
#74436=CARTESIAN_POINT('',(18.18,29.7631649911404,4.47544327974319));
#74437=CARTESIAN_POINT('Origin',(18.3,29.5830832660198,4.47544327974319));
#74438=CARTESIAN_POINT('',(18.3,29.5830832660198,4.47544327974319));
#74439=CARTESIAN_POINT('',(18.3,49.7915416330099,4.47544327974319));
#74440=CARTESIAN_POINT('',(18.18,29.5830832660198,4.47544327974319));
#74441=CARTESIAN_POINT('',(18.3,29.5830832660198,4.47544327974319));
#74442=CARTESIAN_POINT('',(18.18,29.5830832660198,4.47544327974319));
#74443=CARTESIAN_POINT('Origin',(18.3,29.5830832660198,3.78130966834724));
#74444=CARTESIAN_POINT('',(18.3,29.5830832660198,3.78130966834724));
#74445=CARTESIAN_POINT('',(18.3,29.5830832660198,4.64065483417362));
#74446=CARTESIAN_POINT('',(18.18,29.5830832660198,3.78130966834724));
#74447=CARTESIAN_POINT('',(18.3,29.5830832660198,3.78130966834724));
#74448=CARTESIAN_POINT('',(18.18,29.5830832660198,3.78130966834724));
#74449=CARTESIAN_POINT('Origin',(18.3,29.2000000417233,3.78130966834724));
#74450=CARTESIAN_POINT('',(18.3,29.2000000417233,3.78130966834724));
#74451=CARTESIAN_POINT('',(18.3,49.6000000208616,3.78130966834724));
#74452=CARTESIAN_POINT('',(18.18,29.2000000417233,3.78130966834724));
#74453=CARTESIAN_POINT('',(18.3,29.2000000417233,3.78130966834724));
#74454=CARTESIAN_POINT('',(18.18,29.2000000417233,3.78130966834724));
#74455=CARTESIAN_POINT('Origin',(18.3,29.2000000417233,3.58485670797527));
#74456=CARTESIAN_POINT('',(18.3,29.2000000417233,4.54242835398763));
#74457=CARTESIAN_POINT('',(18.18,29.2000000417233,3.58485670797527));
#74458=CARTESIAN_POINT('Origin',(18.18,29.9896316468716,3.29999987538904));
#74459=CARTESIAN_POINT('Origin',(18.3,70.,5.5));
#74460=CARTESIAN_POINT('Origin',(18.3,70.,5.5));
#74461=CARTESIAN_POINT('Origin',(18.3,111.08,8.));
#74462=CARTESIAN_POINT('',(18.3,111.08,8.));
#74463=CARTESIAN_POINT('',(18.3,110.92,8.));
#74464=CARTESIAN_POINT('',(18.3,90.54,8.));
#74465=CARTESIAN_POINT('',(18.18,111.08,8.));
#74466=CARTESIAN_POINT('',(18.3,111.08,8.));
#74467=CARTESIAN_POINT('',(18.18,110.92,8.));
#74468=CARTESIAN_POINT('',(18.18,110.92,8.));
#74469=CARTESIAN_POINT('',(18.3,110.92,8.));
#74470=CARTESIAN_POINT('Origin',(18.3,111.08,9.4));
#74471=CARTESIAN_POINT('',(18.3,111.08,9.4));
#74472=CARTESIAN_POINT('',(18.3,111.08,7.45));
#74473=CARTESIAN_POINT('',(18.18,111.08,9.4));
#74474=CARTESIAN_POINT('',(18.3,111.08,9.4));
#74475=CARTESIAN_POINT('',(18.18,111.08,8.));
#74476=CARTESIAN_POINT('Origin',(18.3,110.92,9.4));
#74477=CARTESIAN_POINT('',(18.3,110.92,9.4));
#74478=CARTESIAN_POINT('',(18.3,90.46,9.4));
#74479=CARTESIAN_POINT('',(18.18,110.92,9.4));
#74480=CARTESIAN_POINT('',(18.3,110.92,9.4));
#74481=CARTESIAN_POINT('',(18.18,111.08,9.4));
#74482=CARTESIAN_POINT('Origin',(18.3,110.92,8.));
#74483=CARTESIAN_POINT('',(18.3,110.92,6.75));
#74484=CARTESIAN_POINT('',(18.18,110.92,9.4));
#74485=CARTESIAN_POINT('Origin',(18.18,111.,8.7));
#74486=CARTESIAN_POINT('Origin',(18.3,109.08,8.));
#74487=CARTESIAN_POINT('',(18.3,109.08,8.));
#74488=CARTESIAN_POINT('',(18.3,108.92,8.));
#74489=CARTESIAN_POINT('',(18.3,89.54,8.));
#74490=CARTESIAN_POINT('',(18.18,109.08,8.));
#74491=CARTESIAN_POINT('',(18.3,109.08,8.));
#74492=CARTESIAN_POINT('',(18.18,108.92,8.));
#74493=CARTESIAN_POINT('',(18.18,108.92,8.));
#74494=CARTESIAN_POINT('',(18.3,108.92,8.));
#74495=CARTESIAN_POINT('Origin',(18.3,109.08,9.4));
#74496=CARTESIAN_POINT('',(18.3,109.08,9.4));
#74497=CARTESIAN_POINT('',(18.3,109.08,7.45));
#74498=CARTESIAN_POINT('',(18.18,109.08,9.4));
#74499=CARTESIAN_POINT('',(18.3,109.08,9.4));
#74500=CARTESIAN_POINT('',(18.18,109.08,8.));
#74501=CARTESIAN_POINT('Origin',(18.3,108.92,9.4));
#74502=CARTESIAN_POINT('',(18.3,108.92,9.4));
#74503=CARTESIAN_POINT('',(18.3,89.46,9.4));
#74504=CARTESIAN_POINT('',(18.18,108.92,9.4));
#74505=CARTESIAN_POINT('',(18.3,108.92,9.4));
#74506=CARTESIAN_POINT('',(18.18,109.08,9.4));
#74507=CARTESIAN_POINT('Origin',(18.3,108.92,8.));
#74508=CARTESIAN_POINT('',(18.3,108.92,6.75));
#74509=CARTESIAN_POINT('',(18.18,108.92,9.4));
#74510=CARTESIAN_POINT('Origin',(18.18,109.,8.7));
#74511=CARTESIAN_POINT('Origin',(18.3,107.08,8.));
#74512=CARTESIAN_POINT('',(18.3,107.08,8.));
#74513=CARTESIAN_POINT('',(18.3,106.92,8.));
#74514=CARTESIAN_POINT('',(18.3,88.54,8.));
#74515=CARTESIAN_POINT('',(18.18,107.08,8.));
#74516=CARTESIAN_POINT('',(18.3,107.08,8.));
#74517=CARTESIAN_POINT('',(18.18,106.92,8.));
#74518=CARTESIAN_POINT('',(18.18,106.92,8.));
#74519=CARTESIAN_POINT('',(18.3,106.92,8.));
#74520=CARTESIAN_POINT('Origin',(18.3,107.08,9.4));
#74521=CARTESIAN_POINT('',(18.3,107.08,9.4));
#74522=CARTESIAN_POINT('',(18.3,107.08,7.45));
#74523=CARTESIAN_POINT('',(18.18,107.08,9.4));
#74524=CARTESIAN_POINT('',(18.3,107.08,9.4));
#74525=CARTESIAN_POINT('',(18.18,107.08,8.));
#74526=CARTESIAN_POINT('Origin',(18.3,106.92,9.4));
#74527=CARTESIAN_POINT('',(18.3,106.92,9.4));
#74528=CARTESIAN_POINT('',(18.3,88.46,9.4));
#74529=CARTESIAN_POINT('',(18.18,106.92,9.4));
#74530=CARTESIAN_POINT('',(18.3,106.92,9.4));
#74531=CARTESIAN_POINT('',(18.18,107.08,9.4));
#74532=CARTESIAN_POINT('Origin',(18.3,106.92,8.));
#74533=CARTESIAN_POINT('',(18.3,106.92,6.75));
#74534=CARTESIAN_POINT('',(18.18,106.92,9.4));
#74535=CARTESIAN_POINT('Origin',(18.18,107.,8.7));
#74536=CARTESIAN_POINT('Origin',(18.3,105.08,7.2));
#74537=CARTESIAN_POINT('',(18.3,105.08,7.2));
#74538=CARTESIAN_POINT('',(18.3,104.92,7.2));
#74539=CARTESIAN_POINT('',(18.3,87.54,7.2));
#74540=CARTESIAN_POINT('',(18.18,105.08,7.2));
#74541=CARTESIAN_POINT('',(18.3,105.08,7.2));
#74542=CARTESIAN_POINT('',(18.18,104.92,7.2));
#74543=CARTESIAN_POINT('',(18.18,104.92,7.2));
#74544=CARTESIAN_POINT('',(18.3,104.92,7.2));
#74545=CARTESIAN_POINT('Origin',(18.3,105.08,9.4));
#74546=CARTESIAN_POINT('',(18.3,105.08,9.4));
#74547=CARTESIAN_POINT('',(18.3,105.08,7.45));
#74548=CARTESIAN_POINT('',(18.18,105.08,9.4));
#74549=CARTESIAN_POINT('',(18.3,105.08,9.4));
#74550=CARTESIAN_POINT('',(18.18,105.08,7.2));
#74551=CARTESIAN_POINT('Origin',(18.3,104.92,9.4));
#74552=CARTESIAN_POINT('',(18.3,104.92,9.4));
#74553=CARTESIAN_POINT('',(18.3,87.46,9.4));
#74554=CARTESIAN_POINT('',(18.18,104.92,9.4));
#74555=CARTESIAN_POINT('',(18.3,104.92,9.4));
#74556=CARTESIAN_POINT('',(18.18,105.08,9.4));
#74557=CARTESIAN_POINT('Origin',(18.3,104.92,7.2));
#74558=CARTESIAN_POINT('',(18.3,104.92,6.35));
#74559=CARTESIAN_POINT('',(18.18,104.92,9.4));
#74560=CARTESIAN_POINT('Origin',(18.18,105.,8.3));
#74561=CARTESIAN_POINT('Origin',(18.3,103.08,8.));
#74562=CARTESIAN_POINT('',(18.3,103.08,8.));
#74563=CARTESIAN_POINT('',(18.3,102.92,8.));
#74564=CARTESIAN_POINT('',(18.3,86.54,8.));
#74565=CARTESIAN_POINT('',(18.18,103.08,8.));
#74566=CARTESIAN_POINT('',(18.3,103.08,8.));
#74567=CARTESIAN_POINT('',(18.18,102.92,8.));
#74568=CARTESIAN_POINT('',(18.18,102.92,8.));
#74569=CARTESIAN_POINT('',(18.3,102.92,8.));
#74570=CARTESIAN_POINT('Origin',(18.3,103.08,9.4));
#74571=CARTESIAN_POINT('',(18.3,103.08,9.4));
#74572=CARTESIAN_POINT('',(18.3,103.08,7.45));
#74573=CARTESIAN_POINT('',(18.18,103.08,9.4));
#74574=CARTESIAN_POINT('',(18.3,103.08,9.4));
#74575=CARTESIAN_POINT('',(18.18,103.08,8.));
#74576=CARTESIAN_POINT('Origin',(18.3,102.92,9.4));
#74577=CARTESIAN_POINT('',(18.3,102.92,9.4));
#74578=CARTESIAN_POINT('',(18.3,86.46,9.4));
#74579=CARTESIAN_POINT('',(18.18,102.92,9.4));
#74580=CARTESIAN_POINT('',(18.3,102.92,9.4));
#74581=CARTESIAN_POINT('',(18.18,103.08,9.4));
#74582=CARTESIAN_POINT('Origin',(18.3,102.92,8.));
#74583=CARTESIAN_POINT('',(18.3,102.92,6.75));
#74584=CARTESIAN_POINT('',(18.18,102.92,9.4));
#74585=CARTESIAN_POINT('Origin',(18.18,103.,8.7));
#74586=CARTESIAN_POINT('Origin',(18.3,101.08,8.));
#74587=CARTESIAN_POINT('',(18.3,101.08,8.));
#74588=CARTESIAN_POINT('',(18.3,100.92,8.));
#74589=CARTESIAN_POINT('',(18.3,85.54,8.));
#74590=CARTESIAN_POINT('',(18.18,101.08,8.));
#74591=CARTESIAN_POINT('',(18.3,101.08,8.));
#74592=CARTESIAN_POINT('',(18.18,100.92,8.));
#74593=CARTESIAN_POINT('',(18.18,100.92,8.));
#74594=CARTESIAN_POINT('',(18.3,100.92,8.));
#74595=CARTESIAN_POINT('Origin',(18.3,101.08,9.4));
#74596=CARTESIAN_POINT('',(18.3,101.08,9.4));
#74597=CARTESIAN_POINT('',(18.3,101.08,7.45));
#74598=CARTESIAN_POINT('',(18.18,101.08,9.4));
#74599=CARTESIAN_POINT('',(18.3,101.08,9.4));
#74600=CARTESIAN_POINT('',(18.18,101.08,8.));
#74601=CARTESIAN_POINT('Origin',(18.3,100.92,9.4));
#74602=CARTESIAN_POINT('',(18.3,100.92,9.4));
#74603=CARTESIAN_POINT('',(18.3,85.46,9.4));
#74604=CARTESIAN_POINT('',(18.18,100.92,9.4));
#74605=CARTESIAN_POINT('',(18.3,100.92,9.4));
#74606=CARTESIAN_POINT('',(18.18,101.08,9.4));
#74607=CARTESIAN_POINT('Origin',(18.3,100.92,8.));
#74608=CARTESIAN_POINT('',(18.3,100.92,6.75));
#74609=CARTESIAN_POINT('',(18.18,100.92,9.4));
#74610=CARTESIAN_POINT('Origin',(18.18,101.,8.7));
#74611=CARTESIAN_POINT('Origin',(18.3,99.08,8.));
#74612=CARTESIAN_POINT('',(18.3,99.08,8.));
#74613=CARTESIAN_POINT('',(18.3,98.92,8.));
#74614=CARTESIAN_POINT('',(18.3,84.54,8.));
#74615=CARTESIAN_POINT('',(18.18,99.08,8.));
#74616=CARTESIAN_POINT('',(18.3,99.08,8.));
#74617=CARTESIAN_POINT('',(18.18,98.92,8.));
#74618=CARTESIAN_POINT('',(18.18,98.92,8.));
#74619=CARTESIAN_POINT('',(18.3,98.92,8.));
#74620=CARTESIAN_POINT('Origin',(18.3,99.08,9.4));
#74621=CARTESIAN_POINT('',(18.3,99.08,9.4));
#74622=CARTESIAN_POINT('',(18.3,99.08,7.45));
#74623=CARTESIAN_POINT('',(18.18,99.08,9.4));
#74624=CARTESIAN_POINT('',(18.3,99.08,9.4));
#74625=CARTESIAN_POINT('',(18.18,99.08,8.));
#74626=CARTESIAN_POINT('Origin',(18.3,98.92,9.4));
#74627=CARTESIAN_POINT('',(18.3,98.92,9.4));
#74628=CARTESIAN_POINT('',(18.3,84.46,9.4));
#74629=CARTESIAN_POINT('',(18.18,98.92,9.4));
#74630=CARTESIAN_POINT('',(18.3,98.92,9.4));
#74631=CARTESIAN_POINT('',(18.18,99.08,9.4));
#74632=CARTESIAN_POINT('Origin',(18.3,98.92,8.));
#74633=CARTESIAN_POINT('',(18.3,98.92,6.75));
#74634=CARTESIAN_POINT('',(18.18,98.92,9.4));
#74635=CARTESIAN_POINT('Origin',(18.18,99.,8.7));
#74636=CARTESIAN_POINT('Origin',(18.3,97.08,8.));
#74637=CARTESIAN_POINT('',(18.3,97.08,8.));
#74638=CARTESIAN_POINT('',(18.3,96.92,8.));
#74639=CARTESIAN_POINT('',(18.3,83.54,8.));
#74640=CARTESIAN_POINT('',(18.18,97.08,8.));
#74641=CARTESIAN_POINT('',(18.3,97.08,8.));
#74642=CARTESIAN_POINT('',(18.18,96.92,8.));
#74643=CARTESIAN_POINT('',(18.18,96.92,8.));
#74644=CARTESIAN_POINT('',(18.3,96.92,8.));
#74645=CARTESIAN_POINT('Origin',(18.3,97.08,9.4));
#74646=CARTESIAN_POINT('',(18.3,97.08,9.4));
#74647=CARTESIAN_POINT('',(18.3,97.08,7.45));
#74648=CARTESIAN_POINT('',(18.18,97.08,9.4));
#74649=CARTESIAN_POINT('',(18.3,97.08,9.4));
#74650=CARTESIAN_POINT('',(18.18,97.08,8.));
#74651=CARTESIAN_POINT('Origin',(18.3,96.92,9.4));
#74652=CARTESIAN_POINT('',(18.3,96.92,9.4));
#74653=CARTESIAN_POINT('',(18.3,83.46,9.4));
#74654=CARTESIAN_POINT('',(18.18,96.92,9.4));
#74655=CARTESIAN_POINT('',(18.3,96.92,9.4));
#74656=CARTESIAN_POINT('',(18.18,97.08,9.4));
#74657=CARTESIAN_POINT('Origin',(18.3,96.92,8.));
#74658=CARTESIAN_POINT('',(18.3,96.92,6.75));
#74659=CARTESIAN_POINT('',(18.18,96.92,9.4));
#74660=CARTESIAN_POINT('Origin',(18.18,97.,8.7));
#74661=CARTESIAN_POINT('Origin',(18.3,95.08,7.2));
#74662=CARTESIAN_POINT('',(18.3,95.08,7.2));
#74663=CARTESIAN_POINT('',(18.3,94.92,7.2));
#74664=CARTESIAN_POINT('',(18.3,82.54,7.2));
#74665=CARTESIAN_POINT('',(18.18,95.08,7.2));
#74666=CARTESIAN_POINT('',(18.3,95.08,7.2));
#74667=CARTESIAN_POINT('',(18.18,94.92,7.2));
#74668=CARTESIAN_POINT('',(18.18,94.92,7.2));
#74669=CARTESIAN_POINT('',(18.3,94.92,7.2));
#74670=CARTESIAN_POINT('Origin',(18.3,95.08,9.4));
#74671=CARTESIAN_POINT('',(18.3,95.08,9.4));
#74672=CARTESIAN_POINT('',(18.3,95.08,7.45));
#74673=CARTESIAN_POINT('',(18.18,95.08,9.4));
#74674=CARTESIAN_POINT('',(18.3,95.08,9.4));
#74675=CARTESIAN_POINT('',(18.18,95.08,7.2));
#74676=CARTESIAN_POINT('Origin',(18.3,94.92,9.4));
#74677=CARTESIAN_POINT('',(18.3,94.92,9.4));
#74678=CARTESIAN_POINT('',(18.3,82.46,9.4));
#74679=CARTESIAN_POINT('',(18.18,94.92,9.4));
#74680=CARTESIAN_POINT('',(18.3,94.92,9.4));
#74681=CARTESIAN_POINT('',(18.18,95.08,9.4));
#74682=CARTESIAN_POINT('Origin',(18.3,94.92,7.2));
#74683=CARTESIAN_POINT('',(18.3,94.92,6.35));
#74684=CARTESIAN_POINT('',(18.18,94.92,9.4));
#74685=CARTESIAN_POINT('Origin',(18.18,95.,8.3));
#74686=CARTESIAN_POINT('Origin',(18.3,93.08,8.));
#74687=CARTESIAN_POINT('',(18.3,93.08,8.));
#74688=CARTESIAN_POINT('',(18.3,92.92,8.));
#74689=CARTESIAN_POINT('',(18.3,81.54,8.));
#74690=CARTESIAN_POINT('',(18.18,93.08,8.));
#74691=CARTESIAN_POINT('',(18.3,93.08,8.));
#74692=CARTESIAN_POINT('',(18.18,92.92,8.));
#74693=CARTESIAN_POINT('',(18.18,92.92,8.));
#74694=CARTESIAN_POINT('',(18.3,92.92,8.));
#74695=CARTESIAN_POINT('Origin',(18.3,93.08,9.4));
#74696=CARTESIAN_POINT('',(18.3,93.08,9.4));
#74697=CARTESIAN_POINT('',(18.3,93.08,7.45));
#74698=CARTESIAN_POINT('',(18.18,93.08,9.4));
#74699=CARTESIAN_POINT('',(18.3,93.08,9.4));
#74700=CARTESIAN_POINT('',(18.18,93.08,8.));
#74701=CARTESIAN_POINT('Origin',(18.3,92.92,9.4));
#74702=CARTESIAN_POINT('',(18.3,92.92,9.4));
#74703=CARTESIAN_POINT('',(18.3,81.46,9.4));
#74704=CARTESIAN_POINT('',(18.18,92.92,9.4));
#74705=CARTESIAN_POINT('',(18.3,92.92,9.4));
#74706=CARTESIAN_POINT('',(18.18,93.08,9.4));
#74707=CARTESIAN_POINT('Origin',(18.3,92.92,8.));
#74708=CARTESIAN_POINT('',(18.3,92.92,6.75));
#74709=CARTESIAN_POINT('',(18.18,92.92,9.4));
#74710=CARTESIAN_POINT('Origin',(18.18,93.,8.7));
#74711=CARTESIAN_POINT('Origin',(18.3,91.08,8.));
#74712=CARTESIAN_POINT('',(18.3,91.08,8.));
#74713=CARTESIAN_POINT('',(18.3,90.92,8.));
#74714=CARTESIAN_POINT('',(18.3,80.54,8.));
#74715=CARTESIAN_POINT('',(18.18,91.08,8.));
#74716=CARTESIAN_POINT('',(18.3,91.08,8.));
#74717=CARTESIAN_POINT('',(18.18,90.92,8.));
#74718=CARTESIAN_POINT('',(18.18,90.92,8.));
#74719=CARTESIAN_POINT('',(18.3,90.92,8.));
#74720=CARTESIAN_POINT('Origin',(18.3,91.08,9.4));
#74721=CARTESIAN_POINT('',(18.3,91.08,9.4));
#74722=CARTESIAN_POINT('',(18.3,91.08,7.45));
#74723=CARTESIAN_POINT('',(18.18,91.08,9.4));
#74724=CARTESIAN_POINT('',(18.3,91.08,9.4));
#74725=CARTESIAN_POINT('',(18.18,91.08,8.));
#74726=CARTESIAN_POINT('Origin',(18.3,90.92,9.4));
#74727=CARTESIAN_POINT('',(18.3,90.92,9.4));
#74728=CARTESIAN_POINT('',(18.3,80.46,9.4));
#74729=CARTESIAN_POINT('',(18.18,90.92,9.4));
#74730=CARTESIAN_POINT('',(18.3,90.92,9.4));
#74731=CARTESIAN_POINT('',(18.18,91.08,9.4));
#74732=CARTESIAN_POINT('Origin',(18.3,90.92,8.));
#74733=CARTESIAN_POINT('',(18.3,90.92,6.75));
#74734=CARTESIAN_POINT('',(18.18,90.92,9.4));
#74735=CARTESIAN_POINT('Origin',(18.18,91.,8.7));
#74736=CARTESIAN_POINT('Origin',(18.3,89.08,8.));
#74737=CARTESIAN_POINT('',(18.3,89.08,8.));
#74738=CARTESIAN_POINT('',(18.3,88.92,8.));
#74739=CARTESIAN_POINT('',(18.3,79.54,8.));
#74740=CARTESIAN_POINT('',(18.18,89.08,8.));
#74741=CARTESIAN_POINT('',(18.3,89.08,8.));
#74742=CARTESIAN_POINT('',(18.18,88.92,8.));
#74743=CARTESIAN_POINT('',(18.18,88.92,8.));
#74744=CARTESIAN_POINT('',(18.3,88.92,8.));
#74745=CARTESIAN_POINT('Origin',(18.3,89.08,9.4));
#74746=CARTESIAN_POINT('',(18.3,89.08,9.4));
#74747=CARTESIAN_POINT('',(18.3,89.08,7.45));
#74748=CARTESIAN_POINT('',(18.18,89.08,9.4));
#74749=CARTESIAN_POINT('',(18.3,89.08,9.4));
#74750=CARTESIAN_POINT('',(18.18,89.08,8.));
#74751=CARTESIAN_POINT('Origin',(18.3,88.92,9.4));
#74752=CARTESIAN_POINT('',(18.3,88.92,9.4));
#74753=CARTESIAN_POINT('',(18.3,79.46,9.4));
#74754=CARTESIAN_POINT('',(18.18,88.92,9.4));
#74755=CARTESIAN_POINT('',(18.3,88.92,9.4));
#74756=CARTESIAN_POINT('',(18.18,89.08,9.4));
#74757=CARTESIAN_POINT('Origin',(18.3,88.92,8.));
#74758=CARTESIAN_POINT('',(18.3,88.92,6.75));
#74759=CARTESIAN_POINT('',(18.18,88.92,9.4));
#74760=CARTESIAN_POINT('Origin',(18.18,89.,8.7));
#74761=CARTESIAN_POINT('Origin',(18.3,87.08,8.));
#74762=CARTESIAN_POINT('',(18.3,87.08,8.));
#74763=CARTESIAN_POINT('',(18.3,86.92,8.));
#74764=CARTESIAN_POINT('',(18.3,78.54,8.));
#74765=CARTESIAN_POINT('',(18.18,87.08,8.));
#74766=CARTESIAN_POINT('',(18.3,87.08,8.));
#74767=CARTESIAN_POINT('',(18.18,86.92,8.));
#74768=CARTESIAN_POINT('',(18.18,86.92,8.));
#74769=CARTESIAN_POINT('',(18.3,86.92,8.));
#74770=CARTESIAN_POINT('Origin',(18.3,87.08,9.4));
#74771=CARTESIAN_POINT('',(18.3,87.08,9.4));
#74772=CARTESIAN_POINT('',(18.3,87.08,7.45));
#74773=CARTESIAN_POINT('',(18.18,87.08,9.4));
#74774=CARTESIAN_POINT('',(18.3,87.08,9.4));
#74775=CARTESIAN_POINT('',(18.18,87.08,8.));
#74776=CARTESIAN_POINT('Origin',(18.3,86.92,9.4));
#74777=CARTESIAN_POINT('',(18.3,86.92,9.4));
#74778=CARTESIAN_POINT('',(18.3,78.46,9.4));
#74779=CARTESIAN_POINT('',(18.18,86.92,9.4));
#74780=CARTESIAN_POINT('',(18.3,86.92,9.4));
#74781=CARTESIAN_POINT('',(18.18,87.08,9.4));
#74782=CARTESIAN_POINT('Origin',(18.3,86.92,8.));
#74783=CARTESIAN_POINT('',(18.3,86.92,6.75));
#74784=CARTESIAN_POINT('',(18.18,86.92,9.4));
#74785=CARTESIAN_POINT('Origin',(18.18,87.,8.7));
#74786=CARTESIAN_POINT('Origin',(18.3,85.08,7.2));
#74787=CARTESIAN_POINT('',(18.3,85.08,7.2));
#74788=CARTESIAN_POINT('',(18.3,84.92,7.2));
#74789=CARTESIAN_POINT('',(18.3,77.54,7.2));
#74790=CARTESIAN_POINT('',(18.18,85.08,7.2));
#74791=CARTESIAN_POINT('',(18.3,85.08,7.2));
#74792=CARTESIAN_POINT('',(18.18,84.92,7.2));
#74793=CARTESIAN_POINT('',(18.18,84.92,7.2));
#74794=CARTESIAN_POINT('',(18.3,84.92,7.2));
#74795=CARTESIAN_POINT('Origin',(18.3,85.08,9.4));
#74796=CARTESIAN_POINT('',(18.3,85.08,9.4));
#74797=CARTESIAN_POINT('',(18.3,85.08,7.45));
#74798=CARTESIAN_POINT('',(18.18,85.08,9.4));
#74799=CARTESIAN_POINT('',(18.3,85.08,9.4));
#74800=CARTESIAN_POINT('',(18.18,85.08,7.2));
#74801=CARTESIAN_POINT('Origin',(18.3,84.92,9.4));
#74802=CARTESIAN_POINT('',(18.3,84.92,9.4));
#74803=CARTESIAN_POINT('',(18.3,77.46,9.4));
#74804=CARTESIAN_POINT('',(18.18,84.92,9.4));
#74805=CARTESIAN_POINT('',(18.3,84.92,9.4));
#74806=CARTESIAN_POINT('',(18.18,85.08,9.4));
#74807=CARTESIAN_POINT('Origin',(18.3,84.92,7.2));
#74808=CARTESIAN_POINT('',(18.3,84.92,6.35));
#74809=CARTESIAN_POINT('',(18.18,84.92,9.4));
#74810=CARTESIAN_POINT('Origin',(18.18,85.,8.3));
#74811=CARTESIAN_POINT('Origin',(18.3,83.08,8.));
#74812=CARTESIAN_POINT('',(18.3,83.08,8.));
#74813=CARTESIAN_POINT('',(18.3,82.92,8.));
#74814=CARTESIAN_POINT('',(18.3,76.54,8.));
#74815=CARTESIAN_POINT('',(18.18,83.08,8.));
#74816=CARTESIAN_POINT('',(18.3,83.08,8.));
#74817=CARTESIAN_POINT('',(18.18,82.92,8.));
#74818=CARTESIAN_POINT('',(18.18,82.92,8.));
#74819=CARTESIAN_POINT('',(18.3,82.92,8.));
#74820=CARTESIAN_POINT('Origin',(18.3,83.08,9.4));
#74821=CARTESIAN_POINT('',(18.3,83.08,9.4));
#74822=CARTESIAN_POINT('',(18.3,83.08,7.45));
#74823=CARTESIAN_POINT('',(18.18,83.08,9.4));
#74824=CARTESIAN_POINT('',(18.3,83.08,9.4));
#74825=CARTESIAN_POINT('',(18.18,83.08,8.));
#74826=CARTESIAN_POINT('Origin',(18.3,82.92,9.4));
#74827=CARTESIAN_POINT('',(18.3,82.92,9.4));
#74828=CARTESIAN_POINT('',(18.3,76.46,9.4));
#74829=CARTESIAN_POINT('',(18.18,82.92,9.4));
#74830=CARTESIAN_POINT('',(18.3,82.92,9.4));
#74831=CARTESIAN_POINT('',(18.18,83.08,9.4));
#74832=CARTESIAN_POINT('Origin',(18.3,82.92,8.));
#74833=CARTESIAN_POINT('',(18.3,82.92,6.75));
#74834=CARTESIAN_POINT('',(18.18,82.92,9.4));
#74835=CARTESIAN_POINT('Origin',(18.18,83.,8.7));
#74836=CARTESIAN_POINT('Origin',(18.3,81.08,8.));
#74837=CARTESIAN_POINT('',(18.3,81.08,8.));
#74838=CARTESIAN_POINT('',(18.3,80.92,8.));
#74839=CARTESIAN_POINT('',(18.3,75.54,8.));
#74840=CARTESIAN_POINT('',(18.18,81.08,8.));
#74841=CARTESIAN_POINT('',(18.3,81.08,8.));
#74842=CARTESIAN_POINT('',(18.18,80.92,8.));
#74843=CARTESIAN_POINT('',(18.18,80.92,8.));
#74844=CARTESIAN_POINT('',(18.3,80.92,8.));
#74845=CARTESIAN_POINT('Origin',(18.3,81.08,9.4));
#74846=CARTESIAN_POINT('',(18.3,81.08,9.4));
#74847=CARTESIAN_POINT('',(18.3,81.08,7.45));
#74848=CARTESIAN_POINT('',(18.18,81.08,9.4));
#74849=CARTESIAN_POINT('',(18.3,81.08,9.4));
#74850=CARTESIAN_POINT('',(18.18,81.08,8.));
#74851=CARTESIAN_POINT('Origin',(18.3,80.92,9.4));
#74852=CARTESIAN_POINT('',(18.3,80.92,9.4));
#74853=CARTESIAN_POINT('',(18.3,75.46,9.4));
#74854=CARTESIAN_POINT('',(18.18,80.92,9.4));
#74855=CARTESIAN_POINT('',(18.3,80.92,9.4));
#74856=CARTESIAN_POINT('',(18.18,81.08,9.4));
#74857=CARTESIAN_POINT('Origin',(18.3,80.92,8.));
#74858=CARTESIAN_POINT('',(18.3,80.92,6.75));
#74859=CARTESIAN_POINT('',(18.18,80.92,9.4));
#74860=CARTESIAN_POINT('Origin',(18.18,81.,8.7));
#74861=CARTESIAN_POINT('Origin',(18.3,79.08,8.));
#74862=CARTESIAN_POINT('',(18.3,79.08,8.));
#74863=CARTESIAN_POINT('',(18.3,78.92,8.));
#74864=CARTESIAN_POINT('',(18.3,74.54,8.));
#74865=CARTESIAN_POINT('',(18.18,79.08,8.));
#74866=CARTESIAN_POINT('',(18.3,79.08,8.));
#74867=CARTESIAN_POINT('',(18.18,78.92,8.));
#74868=CARTESIAN_POINT('',(18.18,78.92,8.));
#74869=CARTESIAN_POINT('',(18.3,78.92,8.));
#74870=CARTESIAN_POINT('Origin',(18.3,79.08,9.4));
#74871=CARTESIAN_POINT('',(18.3,79.08,9.4));
#74872=CARTESIAN_POINT('',(18.3,79.08,7.45));
#74873=CARTESIAN_POINT('',(18.18,79.08,9.4));
#74874=CARTESIAN_POINT('',(18.3,79.08,9.4));
#74875=CARTESIAN_POINT('',(18.18,79.08,8.));
#74876=CARTESIAN_POINT('Origin',(18.3,78.92,9.4));
#74877=CARTESIAN_POINT('',(18.3,78.92,9.4));
#74878=CARTESIAN_POINT('',(18.3,74.46,9.4));
#74879=CARTESIAN_POINT('',(18.18,78.92,9.4));
#74880=CARTESIAN_POINT('',(18.3,78.92,9.4));
#74881=CARTESIAN_POINT('',(18.18,79.08,9.4));
#74882=CARTESIAN_POINT('Origin',(18.3,78.92,8.));
#74883=CARTESIAN_POINT('',(18.3,78.92,6.75));
#74884=CARTESIAN_POINT('',(18.18,78.92,9.4));
#74885=CARTESIAN_POINT('Origin',(18.18,79.,8.7));
#74886=CARTESIAN_POINT('Origin',(18.3,77.08,8.));
#74887=CARTESIAN_POINT('',(18.3,77.08,8.));
#74888=CARTESIAN_POINT('',(18.3,76.92,8.));
#74889=CARTESIAN_POINT('',(18.3,73.54,8.));
#74890=CARTESIAN_POINT('',(18.18,77.08,8.));
#74891=CARTESIAN_POINT('',(18.3,77.08,8.));
#74892=CARTESIAN_POINT('',(18.18,76.92,8.));
#74893=CARTESIAN_POINT('',(18.18,76.92,8.));
#74894=CARTESIAN_POINT('',(18.3,76.92,8.));
#74895=CARTESIAN_POINT('Origin',(18.3,77.08,9.4));
#74896=CARTESIAN_POINT('',(18.3,77.08,9.4));
#74897=CARTESIAN_POINT('',(18.3,77.08,7.45));
#74898=CARTESIAN_POINT('',(18.18,77.08,9.4));
#74899=CARTESIAN_POINT('',(18.3,77.08,9.4));
#74900=CARTESIAN_POINT('',(18.18,77.08,8.));
#74901=CARTESIAN_POINT('Origin',(18.3,76.92,9.4));
#74902=CARTESIAN_POINT('',(18.3,76.92,9.4));
#74903=CARTESIAN_POINT('',(18.3,73.46,9.4));
#74904=CARTESIAN_POINT('',(18.18,76.92,9.4));
#74905=CARTESIAN_POINT('',(18.3,76.92,9.4));
#74906=CARTESIAN_POINT('',(18.18,77.08,9.4));
#74907=CARTESIAN_POINT('Origin',(18.3,76.92,8.));
#74908=CARTESIAN_POINT('',(18.3,76.92,6.75));
#74909=CARTESIAN_POINT('',(18.18,76.92,9.4));
#74910=CARTESIAN_POINT('Origin',(18.18,77.,8.7));
#74911=CARTESIAN_POINT('Origin',(18.3,75.08,7.2));
#74912=CARTESIAN_POINT('',(18.3,75.08,7.2));
#74913=CARTESIAN_POINT('',(18.3,74.92,7.2));
#74914=CARTESIAN_POINT('',(18.3,72.54,7.2));
#74915=CARTESIAN_POINT('',(18.18,75.08,7.2));
#74916=CARTESIAN_POINT('',(18.3,75.08,7.2));
#74917=CARTESIAN_POINT('',(18.18,74.92,7.2));
#74918=CARTESIAN_POINT('',(18.18,74.92,7.2));
#74919=CARTESIAN_POINT('',(18.3,74.92,7.2));
#74920=CARTESIAN_POINT('Origin',(18.3,75.08,9.4));
#74921=CARTESIAN_POINT('',(18.3,75.08,9.4));
#74922=CARTESIAN_POINT('',(18.3,75.08,7.45));
#74923=CARTESIAN_POINT('',(18.18,75.08,9.4));
#74924=CARTESIAN_POINT('',(18.3,75.08,9.4));
#74925=CARTESIAN_POINT('',(18.18,75.08,7.2));
#74926=CARTESIAN_POINT('Origin',(18.3,74.92,9.4));
#74927=CARTESIAN_POINT('',(18.3,74.92,9.4));
#74928=CARTESIAN_POINT('',(18.3,72.46,9.4));
#74929=CARTESIAN_POINT('',(18.18,74.92,9.4));
#74930=CARTESIAN_POINT('',(18.3,74.92,9.4));
#74931=CARTESIAN_POINT('',(18.18,75.08,9.4));
#74932=CARTESIAN_POINT('Origin',(18.3,74.92,7.2));
#74933=CARTESIAN_POINT('',(18.3,74.92,6.35));
#74934=CARTESIAN_POINT('',(18.18,74.92,9.4));
#74935=CARTESIAN_POINT('Origin',(18.18,75.,8.3));
#74936=CARTESIAN_POINT('Origin',(18.3,73.08,8.));
#74937=CARTESIAN_POINT('',(18.3,73.08,8.));
#74938=CARTESIAN_POINT('',(18.3,72.92,8.));
#74939=CARTESIAN_POINT('',(18.3,71.54,8.));
#74940=CARTESIAN_POINT('',(18.18,73.08,8.));
#74941=CARTESIAN_POINT('',(18.3,73.08,8.));
#74942=CARTESIAN_POINT('',(18.18,72.92,8.));
#74943=CARTESIAN_POINT('',(18.18,72.92,8.));
#74944=CARTESIAN_POINT('',(18.3,72.92,8.));
#74945=CARTESIAN_POINT('Origin',(18.3,73.08,9.4));
#74946=CARTESIAN_POINT('',(18.3,73.08,9.4));
#74947=CARTESIAN_POINT('',(18.3,73.08,7.45));
#74948=CARTESIAN_POINT('',(18.18,73.08,9.4));
#74949=CARTESIAN_POINT('',(18.3,73.08,9.4));
#74950=CARTESIAN_POINT('',(18.18,73.08,8.));
#74951=CARTESIAN_POINT('Origin',(18.3,72.92,9.4));
#74952=CARTESIAN_POINT('',(18.3,72.92,9.4));
#74953=CARTESIAN_POINT('',(18.3,71.46,9.4));
#74954=CARTESIAN_POINT('',(18.18,72.92,9.4));
#74955=CARTESIAN_POINT('',(18.3,72.92,9.4));
#74956=CARTESIAN_POINT('',(18.18,73.08,9.4));
#74957=CARTESIAN_POINT('Origin',(18.3,72.92,8.));
#74958=CARTESIAN_POINT('',(18.3,72.92,6.75));
#74959=CARTESIAN_POINT('',(18.18,72.92,9.4));
#74960=CARTESIAN_POINT('Origin',(18.18,73.,8.7));
#74961=CARTESIAN_POINT('Origin',(18.3,71.08,8.));
#74962=CARTESIAN_POINT('',(18.3,71.08,8.));
#74963=CARTESIAN_POINT('',(18.3,70.92,8.));
#74964=CARTESIAN_POINT('',(18.3,70.54,8.));
#74965=CARTESIAN_POINT('',(18.18,71.08,8.));
#74966=CARTESIAN_POINT('',(18.3,71.08,8.));
#74967=CARTESIAN_POINT('',(18.18,70.92,8.));
#74968=CARTESIAN_POINT('',(18.18,70.92,8.));
#74969=CARTESIAN_POINT('',(18.3,70.92,8.));
#74970=CARTESIAN_POINT('Origin',(18.3,71.08,9.4));
#74971=CARTESIAN_POINT('',(18.3,71.08,9.4));
#74972=CARTESIAN_POINT('',(18.3,71.08,7.45));
#74973=CARTESIAN_POINT('',(18.18,71.08,9.4));
#74974=CARTESIAN_POINT('',(18.3,71.08,9.4));
#74975=CARTESIAN_POINT('',(18.18,71.08,8.));
#74976=CARTESIAN_POINT('Origin',(18.3,70.92,9.4));
#74977=CARTESIAN_POINT('',(18.3,70.92,9.4));
#74978=CARTESIAN_POINT('',(18.3,70.46,9.4));
#74979=CARTESIAN_POINT('',(18.18,70.92,9.4));
#74980=CARTESIAN_POINT('',(18.3,70.92,9.4));
#74981=CARTESIAN_POINT('',(18.18,71.08,9.4));
#74982=CARTESIAN_POINT('Origin',(18.3,70.92,8.));
#74983=CARTESIAN_POINT('',(18.3,70.92,6.75));
#74984=CARTESIAN_POINT('',(18.18,70.92,9.4));
#74985=CARTESIAN_POINT('Origin',(18.18,71.,8.7));
#74986=CARTESIAN_POINT('Origin',(18.3,70.08,6.4));
#74987=CARTESIAN_POINT('',(18.3,70.08,6.4));
#74988=CARTESIAN_POINT('',(18.3,69.92,6.4));
#74989=CARTESIAN_POINT('',(18.3,70.04,6.4));
#74990=CARTESIAN_POINT('',(18.18,70.08,6.4));
#74991=CARTESIAN_POINT('',(18.3,70.08,6.4));
#74992=CARTESIAN_POINT('',(18.18,69.92,6.4));
#74993=CARTESIAN_POINT('',(18.18,69.92,6.4));
#74994=CARTESIAN_POINT('',(18.3,69.92,6.4));
#74995=CARTESIAN_POINT('Origin',(18.3,70.08,9.4));
#74996=CARTESIAN_POINT('',(18.3,70.08,9.4));
#74997=CARTESIAN_POINT('',(18.3,70.08,7.45));
#74998=CARTESIAN_POINT('',(18.18,70.08,9.4));
#74999=CARTESIAN_POINT('',(18.3,70.08,9.4));
#75000=CARTESIAN_POINT('',(18.18,70.08,6.4));
#75001=CARTESIAN_POINT('Origin',(18.3,69.92,9.4));
#75002=CARTESIAN_POINT('',(18.3,69.92,9.4));
#75003=CARTESIAN_POINT('',(18.3,69.96,9.4));
#75004=CARTESIAN_POINT('',(18.18,69.92,9.4));
#75005=CARTESIAN_POINT('',(18.3,69.92,9.4));
#75006=CARTESIAN_POINT('',(18.18,70.08,9.4));
#75007=CARTESIAN_POINT('Origin',(18.3,69.92,6.4));
#75008=CARTESIAN_POINT('',(18.3,69.92,5.95));
#75009=CARTESIAN_POINT('',(18.18,69.92,9.4));
#75010=CARTESIAN_POINT('Origin',(18.18,70.,7.9));
#75011=CARTESIAN_POINT('Origin',(18.3,68.08,8.));
#75012=CARTESIAN_POINT('',(18.3,68.08,8.));
#75013=CARTESIAN_POINT('',(18.3,67.92,8.));
#75014=CARTESIAN_POINT('',(18.3,69.04,8.));
#75015=CARTESIAN_POINT('',(18.18,68.08,8.));
#75016=CARTESIAN_POINT('',(18.3,68.08,8.));
#75017=CARTESIAN_POINT('',(18.18,67.92,8.));
#75018=CARTESIAN_POINT('',(18.18,67.92,8.));
#75019=CARTESIAN_POINT('',(18.3,67.92,8.));
#75020=CARTESIAN_POINT('Origin',(18.3,68.08,9.4));
#75021=CARTESIAN_POINT('',(18.3,68.08,9.4));
#75022=CARTESIAN_POINT('',(18.3,68.08,7.45));
#75023=CARTESIAN_POINT('',(18.18,68.08,9.4));
#75024=CARTESIAN_POINT('',(18.3,68.08,9.4));
#75025=CARTESIAN_POINT('',(18.18,68.08,8.));
#75026=CARTESIAN_POINT('Origin',(18.3,67.92,9.4));
#75027=CARTESIAN_POINT('',(18.3,67.92,9.4));
#75028=CARTESIAN_POINT('',(18.3,68.96,9.4));
#75029=CARTESIAN_POINT('',(18.18,67.92,9.4));
#75030=CARTESIAN_POINT('',(18.3,67.92,9.4));
#75031=CARTESIAN_POINT('',(18.18,68.08,9.4));
#75032=CARTESIAN_POINT('Origin',(18.3,67.92,8.));
#75033=CARTESIAN_POINT('',(18.3,67.92,6.75));
#75034=CARTESIAN_POINT('',(18.18,67.92,9.4));
#75035=CARTESIAN_POINT('Origin',(18.18,68.,8.7));
#75036=CARTESIAN_POINT('Origin',(18.3,66.08,8.));
#75037=CARTESIAN_POINT('',(18.3,66.08,8.));
#75038=CARTESIAN_POINT('',(18.3,65.92,8.));
#75039=CARTESIAN_POINT('',(18.3,68.04,8.));
#75040=CARTESIAN_POINT('',(18.18,66.08,8.));
#75041=CARTESIAN_POINT('',(18.3,66.08,8.));
#75042=CARTESIAN_POINT('',(18.18,65.92,8.));
#75043=CARTESIAN_POINT('',(18.18,65.92,8.));
#75044=CARTESIAN_POINT('',(18.3,65.92,8.));
#75045=CARTESIAN_POINT('Origin',(18.3,66.08,9.4));
#75046=CARTESIAN_POINT('',(18.3,66.08,9.4));
#75047=CARTESIAN_POINT('',(18.3,66.08,7.45));
#75048=CARTESIAN_POINT('',(18.18,66.08,9.4));
#75049=CARTESIAN_POINT('',(18.3,66.08,9.4));
#75050=CARTESIAN_POINT('',(18.18,66.08,8.));
#75051=CARTESIAN_POINT('Origin',(18.3,65.92,9.4));
#75052=CARTESIAN_POINT('',(18.3,65.92,9.4));
#75053=CARTESIAN_POINT('',(18.3,67.96,9.4));
#75054=CARTESIAN_POINT('',(18.18,65.92,9.4));
#75055=CARTESIAN_POINT('',(18.3,65.92,9.4));
#75056=CARTESIAN_POINT('',(18.18,66.08,9.4));
#75057=CARTESIAN_POINT('Origin',(18.3,65.92,8.));
#75058=CARTESIAN_POINT('',(18.3,65.92,6.75));
#75059=CARTESIAN_POINT('',(18.18,65.92,9.4));
#75060=CARTESIAN_POINT('Origin',(18.18,66.,8.7));
#75061=CARTESIAN_POINT('Origin',(18.3,64.08,8.));
#75062=CARTESIAN_POINT('',(18.3,64.08,8.));
#75063=CARTESIAN_POINT('',(18.3,63.92,8.));
#75064=CARTESIAN_POINT('',(18.3,67.04,8.));
#75065=CARTESIAN_POINT('',(18.18,64.08,8.));
#75066=CARTESIAN_POINT('',(18.3,64.08,8.));
#75067=CARTESIAN_POINT('',(18.18,63.92,8.));
#75068=CARTESIAN_POINT('',(18.18,63.92,8.));
#75069=CARTESIAN_POINT('',(18.3,63.92,8.));
#75070=CARTESIAN_POINT('Origin',(18.3,64.08,9.4));
#75071=CARTESIAN_POINT('',(18.3,64.08,9.4));
#75072=CARTESIAN_POINT('',(18.3,64.08,7.45));
#75073=CARTESIAN_POINT('',(18.18,64.08,9.4));
#75074=CARTESIAN_POINT('',(18.3,64.08,9.4));
#75075=CARTESIAN_POINT('',(18.18,64.08,8.));
#75076=CARTESIAN_POINT('Origin',(18.3,63.92,9.4));
#75077=CARTESIAN_POINT('',(18.3,63.92,9.4));
#75078=CARTESIAN_POINT('',(18.3,66.96,9.4));
#75079=CARTESIAN_POINT('',(18.18,63.92,9.4));
#75080=CARTESIAN_POINT('',(18.3,63.92,9.4));
#75081=CARTESIAN_POINT('',(18.18,64.08,9.4));
#75082=CARTESIAN_POINT('Origin',(18.3,63.92,8.));
#75083=CARTESIAN_POINT('',(18.3,63.92,6.75));
#75084=CARTESIAN_POINT('',(18.18,63.92,9.4));
#75085=CARTESIAN_POINT('Origin',(18.18,64.,8.7));
#75086=CARTESIAN_POINT('Origin',(18.3,62.08,8.));
#75087=CARTESIAN_POINT('',(18.3,62.08,8.));
#75088=CARTESIAN_POINT('',(18.3,61.92,8.));
#75089=CARTESIAN_POINT('',(18.3,66.04,8.));
#75090=CARTESIAN_POINT('',(18.18,62.08,8.));
#75091=CARTESIAN_POINT('',(18.3,62.08,8.));
#75092=CARTESIAN_POINT('',(18.18,61.92,8.));
#75093=CARTESIAN_POINT('',(18.18,61.92,8.));
#75094=CARTESIAN_POINT('',(18.3,61.92,8.));
#75095=CARTESIAN_POINT('Origin',(18.3,62.08,9.4));
#75096=CARTESIAN_POINT('',(18.3,62.08,9.4));
#75097=CARTESIAN_POINT('',(18.3,62.08,7.45));
#75098=CARTESIAN_POINT('',(18.18,62.08,9.4));
#75099=CARTESIAN_POINT('',(18.3,62.08,9.4));
#75100=CARTESIAN_POINT('',(18.18,62.08,8.));
#75101=CARTESIAN_POINT('Origin',(18.3,61.92,9.4));
#75102=CARTESIAN_POINT('',(18.3,61.92,9.4));
#75103=CARTESIAN_POINT('',(18.3,65.96,9.4));
#75104=CARTESIAN_POINT('',(18.18,61.92,9.4));
#75105=CARTESIAN_POINT('',(18.3,61.92,9.4));
#75106=CARTESIAN_POINT('',(18.18,62.08,9.4));
#75107=CARTESIAN_POINT('Origin',(18.3,61.92,8.));
#75108=CARTESIAN_POINT('',(18.3,61.92,6.75));
#75109=CARTESIAN_POINT('',(18.18,61.92,9.4));
#75110=CARTESIAN_POINT('Origin',(18.18,62.,8.7));
#75111=CARTESIAN_POINT('Origin',(18.3,60.08,6.4));
#75112=CARTESIAN_POINT('',(18.3,60.08,6.4));
#75113=CARTESIAN_POINT('',(18.3,59.92,6.4));
#75114=CARTESIAN_POINT('',(18.3,65.04,6.4));
#75115=CARTESIAN_POINT('',(18.18,60.08,6.4));
#75116=CARTESIAN_POINT('',(18.3,60.08,6.4));
#75117=CARTESIAN_POINT('',(18.18,59.92,6.4));
#75118=CARTESIAN_POINT('',(18.18,59.92,6.4));
#75119=CARTESIAN_POINT('',(18.3,59.92,6.4));
#75120=CARTESIAN_POINT('Origin',(18.3,60.08,9.4));
#75121=CARTESIAN_POINT('',(18.3,60.08,9.4));
#75122=CARTESIAN_POINT('',(18.3,60.08,7.45));
#75123=CARTESIAN_POINT('',(18.18,60.08,9.4));
#75124=CARTESIAN_POINT('',(18.3,60.08,9.4));
#75125=CARTESIAN_POINT('',(18.18,60.08,6.4));
#75126=CARTESIAN_POINT('Origin',(18.3,59.92,9.4));
#75127=CARTESIAN_POINT('',(18.3,59.92,9.4));
#75128=CARTESIAN_POINT('',(18.3,64.96,9.4));
#75129=CARTESIAN_POINT('',(18.18,59.92,9.4));
#75130=CARTESIAN_POINT('',(18.3,59.92,9.4));
#75131=CARTESIAN_POINT('',(18.18,60.08,9.4));
#75132=CARTESIAN_POINT('Origin',(18.3,59.92,6.4));
#75133=CARTESIAN_POINT('',(18.3,59.92,5.95));
#75134=CARTESIAN_POINT('',(18.18,59.92,9.4));
#75135=CARTESIAN_POINT('Origin',(18.18,60.,7.9));
#75136=CARTESIAN_POINT('Origin',(18.3,58.08,8.));
#75137=CARTESIAN_POINT('',(18.3,58.08,8.));
#75138=CARTESIAN_POINT('',(18.3,57.92,8.));
#75139=CARTESIAN_POINT('',(18.3,64.04,8.));
#75140=CARTESIAN_POINT('',(18.18,58.08,8.));
#75141=CARTESIAN_POINT('',(18.3,58.08,8.));
#75142=CARTESIAN_POINT('',(18.18,57.92,8.));
#75143=CARTESIAN_POINT('',(18.18,57.92,8.));
#75144=CARTESIAN_POINT('',(18.3,57.92,8.));
#75145=CARTESIAN_POINT('Origin',(18.3,58.08,9.4));
#75146=CARTESIAN_POINT('',(18.3,58.08,9.4));
#75147=CARTESIAN_POINT('',(18.3,58.08,7.45));
#75148=CARTESIAN_POINT('',(18.18,58.08,9.4));
#75149=CARTESIAN_POINT('',(18.3,58.08,9.4));
#75150=CARTESIAN_POINT('',(18.18,58.08,8.));
#75151=CARTESIAN_POINT('Origin',(18.3,57.92,9.4));
#75152=CARTESIAN_POINT('',(18.3,57.92,9.4));
#75153=CARTESIAN_POINT('',(18.3,63.96,9.4));
#75154=CARTESIAN_POINT('',(18.18,57.92,9.4));
#75155=CARTESIAN_POINT('',(18.3,57.92,9.4));
#75156=CARTESIAN_POINT('',(18.18,58.08,9.4));
#75157=CARTESIAN_POINT('Origin',(18.3,57.92,8.));
#75158=CARTESIAN_POINT('',(18.3,57.92,6.75));
#75159=CARTESIAN_POINT('',(18.18,57.92,9.4));
#75160=CARTESIAN_POINT('Origin',(18.18,58.,8.7));
#75161=CARTESIAN_POINT('Origin',(18.3,56.08,8.));
#75162=CARTESIAN_POINT('',(18.3,56.08,8.));
#75163=CARTESIAN_POINT('',(18.3,55.92,8.));
#75164=CARTESIAN_POINT('',(18.3,63.04,8.));
#75165=CARTESIAN_POINT('',(18.18,56.08,8.));
#75166=CARTESIAN_POINT('',(18.3,56.08,8.));
#75167=CARTESIAN_POINT('',(18.18,55.92,8.));
#75168=CARTESIAN_POINT('',(18.18,55.92,8.));
#75169=CARTESIAN_POINT('',(18.3,55.92,8.));
#75170=CARTESIAN_POINT('Origin',(18.3,56.08,9.4));
#75171=CARTESIAN_POINT('',(18.3,56.08,9.4));
#75172=CARTESIAN_POINT('',(18.3,56.08,7.45));
#75173=CARTESIAN_POINT('',(18.18,56.08,9.4));
#75174=CARTESIAN_POINT('',(18.3,56.08,9.4));
#75175=CARTESIAN_POINT('',(18.18,56.08,8.));
#75176=CARTESIAN_POINT('Origin',(18.3,55.92,9.4));
#75177=CARTESIAN_POINT('',(18.3,55.92,9.4));
#75178=CARTESIAN_POINT('',(18.3,62.96,9.4));
#75179=CARTESIAN_POINT('',(18.18,55.92,9.4));
#75180=CARTESIAN_POINT('',(18.3,55.92,9.4));
#75181=CARTESIAN_POINT('',(18.18,56.08,9.4));
#75182=CARTESIAN_POINT('Origin',(18.3,55.92,8.));
#75183=CARTESIAN_POINT('',(18.3,55.92,6.75));
#75184=CARTESIAN_POINT('',(18.18,55.92,9.4));
#75185=CARTESIAN_POINT('Origin',(18.18,56.,8.7));
#75186=CARTESIAN_POINT('Origin',(18.3,54.08,8.));
#75187=CARTESIAN_POINT('',(18.3,54.08,8.));
#75188=CARTESIAN_POINT('',(18.3,53.92,8.));
#75189=CARTESIAN_POINT('',(18.3,62.04,8.));
#75190=CARTESIAN_POINT('',(18.18,54.08,8.));
#75191=CARTESIAN_POINT('',(18.3,54.08,8.));
#75192=CARTESIAN_POINT('',(18.18,53.92,8.));
#75193=CARTESIAN_POINT('',(18.18,53.92,8.));
#75194=CARTESIAN_POINT('',(18.3,53.92,8.));
#75195=CARTESIAN_POINT('Origin',(18.3,54.08,9.4));
#75196=CARTESIAN_POINT('',(18.3,54.08,9.4));
#75197=CARTESIAN_POINT('',(18.3,54.08,7.45));
#75198=CARTESIAN_POINT('',(18.18,54.08,9.4));
#75199=CARTESIAN_POINT('',(18.3,54.08,9.4));
#75200=CARTESIAN_POINT('',(18.18,54.08,8.));
#75201=CARTESIAN_POINT('Origin',(18.3,53.92,9.4));
#75202=CARTESIAN_POINT('',(18.3,53.92,9.4));
#75203=CARTESIAN_POINT('',(18.3,61.96,9.4));
#75204=CARTESIAN_POINT('',(18.18,53.92,9.4));
#75205=CARTESIAN_POINT('',(18.3,53.92,9.4));
#75206=CARTESIAN_POINT('',(18.18,54.08,9.4));
#75207=CARTESIAN_POINT('Origin',(18.3,53.92,8.));
#75208=CARTESIAN_POINT('',(18.3,53.92,6.75));
#75209=CARTESIAN_POINT('',(18.18,53.92,9.4));
#75210=CARTESIAN_POINT('Origin',(18.18,54.,8.7));
#75211=CARTESIAN_POINT('Origin',(18.3,52.08,8.));
#75212=CARTESIAN_POINT('',(18.3,52.08,8.));
#75213=CARTESIAN_POINT('',(18.3,51.92,8.));
#75214=CARTESIAN_POINT('',(18.3,61.04,8.));
#75215=CARTESIAN_POINT('',(18.18,52.08,8.));
#75216=CARTESIAN_POINT('',(18.3,52.08,8.));
#75217=CARTESIAN_POINT('',(18.18,51.92,8.));
#75218=CARTESIAN_POINT('',(18.18,51.92,8.));
#75219=CARTESIAN_POINT('',(18.3,51.92,8.));
#75220=CARTESIAN_POINT('Origin',(18.3,52.08,9.4));
#75221=CARTESIAN_POINT('',(18.3,52.08,9.4));
#75222=CARTESIAN_POINT('',(18.3,52.08,7.45));
#75223=CARTESIAN_POINT('',(18.18,52.08,9.4));
#75224=CARTESIAN_POINT('',(18.3,52.08,9.4));
#75225=CARTESIAN_POINT('',(18.18,52.08,8.));
#75226=CARTESIAN_POINT('Origin',(18.3,51.92,9.4));
#75227=CARTESIAN_POINT('',(18.3,51.92,9.4));
#75228=CARTESIAN_POINT('',(18.3,60.96,9.4));
#75229=CARTESIAN_POINT('',(18.18,51.92,9.4));
#75230=CARTESIAN_POINT('',(18.3,51.92,9.4));
#75231=CARTESIAN_POINT('',(18.18,52.08,9.4));
#75232=CARTESIAN_POINT('Origin',(18.3,51.92,8.));
#75233=CARTESIAN_POINT('',(18.3,51.92,6.75));
#75234=CARTESIAN_POINT('',(18.18,51.92,9.4));
#75235=CARTESIAN_POINT('Origin',(18.18,52.,8.7));
#75236=CARTESIAN_POINT('Origin',(18.3,50.08,6.4));
#75237=CARTESIAN_POINT('',(18.3,50.08,6.4));
#75238=CARTESIAN_POINT('',(18.3,49.92,6.4));
#75239=CARTESIAN_POINT('',(18.3,60.04,6.4));
#75240=CARTESIAN_POINT('',(18.18,50.08,6.4));
#75241=CARTESIAN_POINT('',(18.3,50.08,6.4));
#75242=CARTESIAN_POINT('',(18.18,49.92,6.4));
#75243=CARTESIAN_POINT('',(18.18,49.92,6.4));
#75244=CARTESIAN_POINT('',(18.3,49.92,6.4));
#75245=CARTESIAN_POINT('Origin',(18.3,50.08,9.4));
#75246=CARTESIAN_POINT('',(18.3,50.08,9.4));
#75247=CARTESIAN_POINT('',(18.3,50.08,7.45));
#75248=CARTESIAN_POINT('',(18.18,50.08,9.4));
#75249=CARTESIAN_POINT('',(18.3,50.08,9.4));
#75250=CARTESIAN_POINT('',(18.18,50.08,6.4));
#75251=CARTESIAN_POINT('Origin',(18.3,49.92,9.4));
#75252=CARTESIAN_POINT('',(18.3,49.92,9.4));
#75253=CARTESIAN_POINT('',(18.3,59.96,9.4));
#75254=CARTESIAN_POINT('',(18.18,49.92,9.4));
#75255=CARTESIAN_POINT('',(18.3,49.92,9.4));
#75256=CARTESIAN_POINT('',(18.18,50.08,9.4));
#75257=CARTESIAN_POINT('Origin',(18.3,49.92,6.4));
#75258=CARTESIAN_POINT('',(18.3,49.92,5.95));
#75259=CARTESIAN_POINT('',(18.18,49.92,9.4));
#75260=CARTESIAN_POINT('Origin',(18.18,50.,7.9));
#75261=CARTESIAN_POINT('Origin',(18.3,48.08,8.));
#75262=CARTESIAN_POINT('',(18.3,48.08,8.));
#75263=CARTESIAN_POINT('',(18.3,47.92,8.));
#75264=CARTESIAN_POINT('',(18.3,59.04,8.));
#75265=CARTESIAN_POINT('',(18.18,48.08,8.));
#75266=CARTESIAN_POINT('',(18.3,48.08,8.));
#75267=CARTESIAN_POINT('',(18.18,47.92,8.));
#75268=CARTESIAN_POINT('',(18.18,47.92,8.));
#75269=CARTESIAN_POINT('',(18.3,47.92,8.));
#75270=CARTESIAN_POINT('Origin',(18.3,48.08,9.4));
#75271=CARTESIAN_POINT('',(18.3,48.08,9.4));
#75272=CARTESIAN_POINT('',(18.3,48.08,7.45));
#75273=CARTESIAN_POINT('',(18.18,48.08,9.4));
#75274=CARTESIAN_POINT('',(18.3,48.08,9.4));
#75275=CARTESIAN_POINT('',(18.18,48.08,8.));
#75276=CARTESIAN_POINT('Origin',(18.3,47.92,9.4));
#75277=CARTESIAN_POINT('',(18.3,47.92,9.4));
#75278=CARTESIAN_POINT('',(18.3,58.96,9.4));
#75279=CARTESIAN_POINT('',(18.18,47.92,9.4));
#75280=CARTESIAN_POINT('',(18.3,47.92,9.4));
#75281=CARTESIAN_POINT('',(18.18,48.08,9.4));
#75282=CARTESIAN_POINT('Origin',(18.3,47.92,8.));
#75283=CARTESIAN_POINT('',(18.3,47.92,6.75));
#75284=CARTESIAN_POINT('',(18.18,47.92,9.4));
#75285=CARTESIAN_POINT('Origin',(18.18,48.,8.7));
#75286=CARTESIAN_POINT('Origin',(18.3,46.08,8.));
#75287=CARTESIAN_POINT('',(18.3,46.08,8.));
#75288=CARTESIAN_POINT('',(18.3,45.92,8.));
#75289=CARTESIAN_POINT('',(18.3,58.04,8.));
#75290=CARTESIAN_POINT('',(18.18,46.08,8.));
#75291=CARTESIAN_POINT('',(18.3,46.08,8.));
#75292=CARTESIAN_POINT('',(18.18,45.92,8.));
#75293=CARTESIAN_POINT('',(18.18,45.92,8.));
#75294=CARTESIAN_POINT('',(18.3,45.92,8.));
#75295=CARTESIAN_POINT('Origin',(18.3,46.08,9.4));
#75296=CARTESIAN_POINT('',(18.3,46.08,9.4));
#75297=CARTESIAN_POINT('',(18.3,46.08,7.45));
#75298=CARTESIAN_POINT('',(18.18,46.08,9.4));
#75299=CARTESIAN_POINT('',(18.3,46.08,9.4));
#75300=CARTESIAN_POINT('',(18.18,46.08,8.));
#75301=CARTESIAN_POINT('Origin',(18.3,45.92,9.4));
#75302=CARTESIAN_POINT('',(18.3,45.92,9.4));
#75303=CARTESIAN_POINT('',(18.3,57.96,9.4));
#75304=CARTESIAN_POINT('',(18.18,45.92,9.4));
#75305=CARTESIAN_POINT('',(18.3,45.92,9.4));
#75306=CARTESIAN_POINT('',(18.18,46.08,9.4));
#75307=CARTESIAN_POINT('Origin',(18.3,45.92,8.));
#75308=CARTESIAN_POINT('',(18.3,45.92,6.75));
#75309=CARTESIAN_POINT('',(18.18,45.92,9.4));
#75310=CARTESIAN_POINT('Origin',(18.18,46.,8.7));
#75311=CARTESIAN_POINT('Origin',(18.3,44.08,8.));
#75312=CARTESIAN_POINT('',(18.3,44.08,8.));
#75313=CARTESIAN_POINT('',(18.3,43.92,8.));
#75314=CARTESIAN_POINT('',(18.3,57.04,8.));
#75315=CARTESIAN_POINT('',(18.18,44.08,8.));
#75316=CARTESIAN_POINT('',(18.3,44.08,8.));
#75317=CARTESIAN_POINT('',(18.18,43.92,8.));
#75318=CARTESIAN_POINT('',(18.18,43.92,8.));
#75319=CARTESIAN_POINT('',(18.3,43.92,8.));
#75320=CARTESIAN_POINT('Origin',(18.3,44.08,9.4));
#75321=CARTESIAN_POINT('',(18.3,44.08,9.4));
#75322=CARTESIAN_POINT('',(18.3,44.08,7.45));
#75323=CARTESIAN_POINT('',(18.18,44.08,9.4));
#75324=CARTESIAN_POINT('',(18.3,44.08,9.4));
#75325=CARTESIAN_POINT('',(18.18,44.08,8.));
#75326=CARTESIAN_POINT('Origin',(18.3,43.92,9.4));
#75327=CARTESIAN_POINT('',(18.3,43.92,9.4));
#75328=CARTESIAN_POINT('',(18.3,56.96,9.4));
#75329=CARTESIAN_POINT('',(18.18,43.92,9.4));
#75330=CARTESIAN_POINT('',(18.3,43.92,9.4));
#75331=CARTESIAN_POINT('',(18.18,44.08,9.4));
#75332=CARTESIAN_POINT('Origin',(18.3,43.92,8.));
#75333=CARTESIAN_POINT('',(18.3,43.92,6.75));
#75334=CARTESIAN_POINT('',(18.18,43.92,9.4));
#75335=CARTESIAN_POINT('Origin',(18.18,44.,8.7));
#75336=CARTESIAN_POINT('Origin',(18.3,42.08,8.));
#75337=CARTESIAN_POINT('',(18.3,42.08,8.));
#75338=CARTESIAN_POINT('',(18.3,41.92,8.));
#75339=CARTESIAN_POINT('',(18.3,56.04,8.));
#75340=CARTESIAN_POINT('',(18.18,42.08,8.));
#75341=CARTESIAN_POINT('',(18.3,42.08,8.));
#75342=CARTESIAN_POINT('',(18.18,41.92,8.));
#75343=CARTESIAN_POINT('',(18.18,41.92,8.));
#75344=CARTESIAN_POINT('',(18.3,41.92,8.));
#75345=CARTESIAN_POINT('Origin',(18.3,42.08,9.4));
#75346=CARTESIAN_POINT('',(18.3,42.08,9.4));
#75347=CARTESIAN_POINT('',(18.3,42.08,7.45));
#75348=CARTESIAN_POINT('',(18.18,42.08,9.4));
#75349=CARTESIAN_POINT('',(18.3,42.08,9.4));
#75350=CARTESIAN_POINT('',(18.18,42.08,8.));
#75351=CARTESIAN_POINT('Origin',(18.3,41.92,9.4));
#75352=CARTESIAN_POINT('',(18.3,41.92,9.4));
#75353=CARTESIAN_POINT('',(18.3,55.96,9.4));
#75354=CARTESIAN_POINT('',(18.18,41.92,9.4));
#75355=CARTESIAN_POINT('',(18.3,41.92,9.4));
#75356=CARTESIAN_POINT('',(18.18,42.08,9.4));
#75357=CARTESIAN_POINT('Origin',(18.3,41.92,8.));
#75358=CARTESIAN_POINT('',(18.3,41.92,6.75));
#75359=CARTESIAN_POINT('',(18.18,41.92,9.4));
#75360=CARTESIAN_POINT('Origin',(18.18,42.,8.7));
#75361=CARTESIAN_POINT('Origin',(18.3,40.08,6.4));
#75362=CARTESIAN_POINT('',(18.3,40.08,6.4));
#75363=CARTESIAN_POINT('',(18.3,39.92,6.4));
#75364=CARTESIAN_POINT('',(18.3,55.04,6.4));
#75365=CARTESIAN_POINT('',(18.18,40.08,6.4));
#75366=CARTESIAN_POINT('',(18.3,40.08,6.4));
#75367=CARTESIAN_POINT('',(18.18,39.92,6.4));
#75368=CARTESIAN_POINT('',(18.18,39.92,6.4));
#75369=CARTESIAN_POINT('',(18.3,39.92,6.4));
#75370=CARTESIAN_POINT('Origin',(18.3,40.08,9.4));
#75371=CARTESIAN_POINT('',(18.3,40.08,9.4));
#75372=CARTESIAN_POINT('',(18.3,40.08,7.45));
#75373=CARTESIAN_POINT('',(18.18,40.08,9.4));
#75374=CARTESIAN_POINT('',(18.3,40.08,9.4));
#75375=CARTESIAN_POINT('',(18.18,40.08,6.4));
#75376=CARTESIAN_POINT('Origin',(18.3,39.92,9.4));
#75377=CARTESIAN_POINT('',(18.3,39.92,9.4));
#75378=CARTESIAN_POINT('',(18.3,54.96,9.4));
#75379=CARTESIAN_POINT('',(18.18,39.92,9.4));
#75380=CARTESIAN_POINT('',(18.3,39.92,9.4));
#75381=CARTESIAN_POINT('',(18.18,40.08,9.4));
#75382=CARTESIAN_POINT('Origin',(18.3,39.92,6.4));
#75383=CARTESIAN_POINT('',(18.3,39.92,5.95));
#75384=CARTESIAN_POINT('',(18.18,39.92,9.4));
#75385=CARTESIAN_POINT('Origin',(18.18,40.,7.9));
#75386=CARTESIAN_POINT('Origin',(18.3,38.08,8.));
#75387=CARTESIAN_POINT('',(18.3,38.08,8.));
#75388=CARTESIAN_POINT('',(18.3,37.92,8.));
#75389=CARTESIAN_POINT('',(18.3,54.04,8.));
#75390=CARTESIAN_POINT('',(18.18,38.08,8.));
#75391=CARTESIAN_POINT('',(18.3,38.08,8.));
#75392=CARTESIAN_POINT('',(18.18,37.92,8.));
#75393=CARTESIAN_POINT('',(18.18,37.92,8.));
#75394=CARTESIAN_POINT('',(18.3,37.92,8.));
#75395=CARTESIAN_POINT('Origin',(18.3,38.08,9.4));
#75396=CARTESIAN_POINT('',(18.3,38.08,9.4));
#75397=CARTESIAN_POINT('',(18.3,38.08,7.45));
#75398=CARTESIAN_POINT('',(18.18,38.08,9.4));
#75399=CARTESIAN_POINT('',(18.3,38.08,9.4));
#75400=CARTESIAN_POINT('',(18.18,38.08,8.));
#75401=CARTESIAN_POINT('Origin',(18.3,37.92,9.4));
#75402=CARTESIAN_POINT('',(18.3,37.92,9.4));
#75403=CARTESIAN_POINT('',(18.3,53.96,9.4));
#75404=CARTESIAN_POINT('',(18.18,37.92,9.4));
#75405=CARTESIAN_POINT('',(18.3,37.92,9.4));
#75406=CARTESIAN_POINT('',(18.18,38.08,9.4));
#75407=CARTESIAN_POINT('Origin',(18.3,37.92,8.));
#75408=CARTESIAN_POINT('',(18.3,37.92,6.75));
#75409=CARTESIAN_POINT('',(18.18,37.92,9.4));
#75410=CARTESIAN_POINT('Origin',(18.18,38.,8.7));
#75411=CARTESIAN_POINT('Origin',(18.3,36.08,8.));
#75412=CARTESIAN_POINT('',(18.3,36.08,8.));
#75413=CARTESIAN_POINT('',(18.3,35.92,8.));
#75414=CARTESIAN_POINT('',(18.3,53.04,8.));
#75415=CARTESIAN_POINT('',(18.18,36.08,8.));
#75416=CARTESIAN_POINT('',(18.3,36.08,8.));
#75417=CARTESIAN_POINT('',(18.18,35.92,8.));
#75418=CARTESIAN_POINT('',(18.18,35.92,8.));
#75419=CARTESIAN_POINT('',(18.3,35.92,8.));
#75420=CARTESIAN_POINT('Origin',(18.3,36.08,9.4));
#75421=CARTESIAN_POINT('',(18.3,36.08,9.4));
#75422=CARTESIAN_POINT('',(18.3,36.08,7.45));
#75423=CARTESIAN_POINT('',(18.18,36.08,9.4));
#75424=CARTESIAN_POINT('',(18.3,36.08,9.4));
#75425=CARTESIAN_POINT('',(18.18,36.08,8.));
#75426=CARTESIAN_POINT('Origin',(18.3,35.92,9.4));
#75427=CARTESIAN_POINT('',(18.3,35.92,9.4));
#75428=CARTESIAN_POINT('',(18.3,52.96,9.4));
#75429=CARTESIAN_POINT('',(18.18,35.92,9.4));
#75430=CARTESIAN_POINT('',(18.3,35.92,9.4));
#75431=CARTESIAN_POINT('',(18.18,36.08,9.4));
#75432=CARTESIAN_POINT('Origin',(18.3,35.92,8.));
#75433=CARTESIAN_POINT('',(18.3,35.92,6.75));
#75434=CARTESIAN_POINT('',(18.18,35.92,9.4));
#75435=CARTESIAN_POINT('Origin',(18.18,36.,8.7));
#75436=CARTESIAN_POINT('Origin',(18.3,34.08,8.));
#75437=CARTESIAN_POINT('',(18.3,34.08,8.));
#75438=CARTESIAN_POINT('',(18.3,33.92,8.));
#75439=CARTESIAN_POINT('',(18.3,52.04,8.));
#75440=CARTESIAN_POINT('',(18.18,34.08,8.));
#75441=CARTESIAN_POINT('',(18.3,34.08,8.));
#75442=CARTESIAN_POINT('',(18.18,33.92,8.));
#75443=CARTESIAN_POINT('',(18.18,33.92,8.));
#75444=CARTESIAN_POINT('',(18.3,33.92,8.));
#75445=CARTESIAN_POINT('Origin',(18.3,34.08,9.4));
#75446=CARTESIAN_POINT('',(18.3,34.08,9.4));
#75447=CARTESIAN_POINT('',(18.3,34.08,7.45));
#75448=CARTESIAN_POINT('',(18.18,34.08,9.4));
#75449=CARTESIAN_POINT('',(18.3,34.08,9.4));
#75450=CARTESIAN_POINT('',(18.18,34.08,8.));
#75451=CARTESIAN_POINT('Origin',(18.3,33.92,9.4));
#75452=CARTESIAN_POINT('',(18.3,33.92,9.4));
#75453=CARTESIAN_POINT('',(18.3,51.96,9.4));
#75454=CARTESIAN_POINT('',(18.18,33.92,9.4));
#75455=CARTESIAN_POINT('',(18.3,33.92,9.4));
#75456=CARTESIAN_POINT('',(18.18,34.08,9.4));
#75457=CARTESIAN_POINT('Origin',(18.3,33.92,8.));
#75458=CARTESIAN_POINT('',(18.3,33.92,6.75));
#75459=CARTESIAN_POINT('',(18.18,33.92,9.4));
#75460=CARTESIAN_POINT('Origin',(18.18,34.,8.7));
#75461=CARTESIAN_POINT('Origin',(18.3,32.08,8.));
#75462=CARTESIAN_POINT('',(18.3,32.08,8.));
#75463=CARTESIAN_POINT('',(18.3,31.92,8.));
#75464=CARTESIAN_POINT('',(18.3,51.04,8.));
#75465=CARTESIAN_POINT('',(18.18,32.08,8.));
#75466=CARTESIAN_POINT('',(18.3,32.08,8.));
#75467=CARTESIAN_POINT('',(18.18,31.92,8.));
#75468=CARTESIAN_POINT('',(18.18,31.92,8.));
#75469=CARTESIAN_POINT('',(18.3,31.92,8.));
#75470=CARTESIAN_POINT('Origin',(18.3,32.08,9.4));
#75471=CARTESIAN_POINT('',(18.3,32.08,9.4));
#75472=CARTESIAN_POINT('',(18.3,32.08,7.45));
#75473=CARTESIAN_POINT('',(18.18,32.08,9.4));
#75474=CARTESIAN_POINT('',(18.3,32.08,9.4));
#75475=CARTESIAN_POINT('',(18.18,32.08,8.));
#75476=CARTESIAN_POINT('Origin',(18.3,31.92,9.4));
#75477=CARTESIAN_POINT('',(18.3,31.92,9.4));
#75478=CARTESIAN_POINT('',(18.3,50.96,9.4));
#75479=CARTESIAN_POINT('',(18.18,31.92,9.4));
#75480=CARTESIAN_POINT('',(18.3,31.92,9.4));
#75481=CARTESIAN_POINT('',(18.18,32.08,9.4));
#75482=CARTESIAN_POINT('Origin',(18.3,31.92,8.));
#75483=CARTESIAN_POINT('',(18.3,31.92,6.75));
#75484=CARTESIAN_POINT('',(18.18,31.92,9.4));
#75485=CARTESIAN_POINT('Origin',(18.18,32.,8.7));
#75486=CARTESIAN_POINT('Origin',(18.3,30.08,6.4));
#75487=CARTESIAN_POINT('',(18.3,30.08,6.4));
#75488=CARTESIAN_POINT('',(18.3,29.92,6.4));
#75489=CARTESIAN_POINT('',(18.3,50.04,6.4));
#75490=CARTESIAN_POINT('',(18.18,30.08,6.4));
#75491=CARTESIAN_POINT('',(18.3,30.08,6.4));
#75492=CARTESIAN_POINT('',(18.18,29.92,6.4));
#75493=CARTESIAN_POINT('',(18.18,29.92,6.4));
#75494=CARTESIAN_POINT('',(18.3,29.92,6.4));
#75495=CARTESIAN_POINT('Origin',(18.3,30.08,9.4));
#75496=CARTESIAN_POINT('',(18.3,30.08,9.4));
#75497=CARTESIAN_POINT('',(18.3,30.08,7.45));
#75498=CARTESIAN_POINT('',(18.18,30.08,9.4));
#75499=CARTESIAN_POINT('',(18.3,30.08,9.4));
#75500=CARTESIAN_POINT('',(18.18,30.08,6.4));
#75501=CARTESIAN_POINT('Origin',(18.3,29.92,9.4));
#75502=CARTESIAN_POINT('',(18.3,29.92,9.4));
#75503=CARTESIAN_POINT('',(18.3,49.96,9.4));
#75504=CARTESIAN_POINT('',(18.18,29.92,9.4));
#75505=CARTESIAN_POINT('',(18.3,29.92,9.4));
#75506=CARTESIAN_POINT('',(18.18,30.08,9.4));
#75507=CARTESIAN_POINT('Origin',(18.3,29.92,6.4));
#75508=CARTESIAN_POINT('',(18.3,29.92,5.95));
#75509=CARTESIAN_POINT('',(18.18,29.92,9.4));
#75510=CARTESIAN_POINT('Origin',(18.18,30.,7.9));
#75511=CARTESIAN_POINT('Origin',(18.3,29.08,8.));
#75512=CARTESIAN_POINT('',(18.3,29.08,8.));
#75513=CARTESIAN_POINT('',(18.3,28.92,8.));
#75514=CARTESIAN_POINT('',(18.3,49.54,8.));
#75515=CARTESIAN_POINT('',(18.18,29.08,8.));
#75516=CARTESIAN_POINT('',(18.3,29.08,8.));
#75517=CARTESIAN_POINT('',(18.18,28.92,8.));
#75518=CARTESIAN_POINT('',(18.18,28.92,8.));
#75519=CARTESIAN_POINT('',(18.3,28.92,8.));
#75520=CARTESIAN_POINT('Origin',(18.3,29.08,9.4));
#75521=CARTESIAN_POINT('',(18.3,29.08,9.4));
#75522=CARTESIAN_POINT('',(18.3,29.08,7.45));
#75523=CARTESIAN_POINT('',(18.18,29.08,9.4));
#75524=CARTESIAN_POINT('',(18.3,29.08,9.4));
#75525=CARTESIAN_POINT('',(18.18,29.08,8.));
#75526=CARTESIAN_POINT('Origin',(18.3,28.92,9.4));
#75527=CARTESIAN_POINT('',(18.3,28.92,9.4));
#75528=CARTESIAN_POINT('',(18.3,49.46,9.4));
#75529=CARTESIAN_POINT('',(18.18,28.92,9.4));
#75530=CARTESIAN_POINT('',(18.3,28.92,9.4));
#75531=CARTESIAN_POINT('',(18.18,29.08,9.4));
#75532=CARTESIAN_POINT('Origin',(18.3,28.92,8.));
#75533=CARTESIAN_POINT('',(18.3,28.92,6.75));
#75534=CARTESIAN_POINT('',(18.18,28.92,9.4));
#75535=CARTESIAN_POINT('Origin',(18.18,29.,8.7));
#75536=CARTESIAN_POINT('Origin',(18.3,31.08,8.));
#75537=CARTESIAN_POINT('',(18.3,31.08,8.));
#75538=CARTESIAN_POINT('',(18.3,30.92,8.));
#75539=CARTESIAN_POINT('',(18.3,50.54,8.));
#75540=CARTESIAN_POINT('',(18.18,31.08,8.));
#75541=CARTESIAN_POINT('',(18.3,31.08,8.));
#75542=CARTESIAN_POINT('',(18.18,30.92,8.));
#75543=CARTESIAN_POINT('',(18.18,30.92,8.));
#75544=CARTESIAN_POINT('',(18.3,30.92,8.));
#75545=CARTESIAN_POINT('Origin',(18.3,31.08,9.4));
#75546=CARTESIAN_POINT('',(18.3,31.08,9.4));
#75547=CARTESIAN_POINT('',(18.3,31.08,7.45));
#75548=CARTESIAN_POINT('',(18.18,31.08,9.4));
#75549=CARTESIAN_POINT('',(18.3,31.08,9.4));
#75550=CARTESIAN_POINT('',(18.18,31.08,8.));
#75551=CARTESIAN_POINT('Origin',(18.3,30.92,9.4));
#75552=CARTESIAN_POINT('',(18.3,30.92,9.4));
#75553=CARTESIAN_POINT('',(18.3,50.46,9.4));
#75554=CARTESIAN_POINT('',(18.18,30.92,9.4));
#75555=CARTESIAN_POINT('',(18.3,30.92,9.4));
#75556=CARTESIAN_POINT('',(18.18,31.08,9.4));
#75557=CARTESIAN_POINT('Origin',(18.3,30.92,8.));
#75558=CARTESIAN_POINT('',(18.3,30.92,6.75));
#75559=CARTESIAN_POINT('',(18.18,30.92,9.4));
#75560=CARTESIAN_POINT('Origin',(18.18,31.,8.7));
#75561=CARTESIAN_POINT('Origin',(18.3,33.08,8.));
#75562=CARTESIAN_POINT('',(18.3,33.08,8.));
#75563=CARTESIAN_POINT('',(18.3,32.92,8.));
#75564=CARTESIAN_POINT('',(18.3,51.54,8.));
#75565=CARTESIAN_POINT('',(18.18,33.08,8.));
#75566=CARTESIAN_POINT('',(18.3,33.08,8.));
#75567=CARTESIAN_POINT('',(18.18,32.92,8.));
#75568=CARTESIAN_POINT('',(18.18,32.92,8.));
#75569=CARTESIAN_POINT('',(18.3,32.92,8.));
#75570=CARTESIAN_POINT('Origin',(18.3,33.08,9.4));
#75571=CARTESIAN_POINT('',(18.3,33.08,9.4));
#75572=CARTESIAN_POINT('',(18.3,33.08,7.45));
#75573=CARTESIAN_POINT('',(18.18,33.08,9.4));
#75574=CARTESIAN_POINT('',(18.3,33.08,9.4));
#75575=CARTESIAN_POINT('',(18.18,33.08,8.));
#75576=CARTESIAN_POINT('Origin',(18.3,32.92,9.4));
#75577=CARTESIAN_POINT('',(18.3,32.92,9.4));
#75578=CARTESIAN_POINT('',(18.3,51.46,9.4));
#75579=CARTESIAN_POINT('',(18.18,32.92,9.4));
#75580=CARTESIAN_POINT('',(18.3,32.92,9.4));
#75581=CARTESIAN_POINT('',(18.18,33.08,9.4));
#75582=CARTESIAN_POINT('Origin',(18.3,32.92,8.));
#75583=CARTESIAN_POINT('',(18.3,32.92,6.75));
#75584=CARTESIAN_POINT('',(18.18,32.92,9.4));
#75585=CARTESIAN_POINT('Origin',(18.18,33.,8.7));
#75586=CARTESIAN_POINT('Origin',(18.3,35.08,7.2));
#75587=CARTESIAN_POINT('',(18.3,35.08,7.2));
#75588=CARTESIAN_POINT('',(18.3,34.92,7.2));
#75589=CARTESIAN_POINT('',(18.3,52.54,7.2));
#75590=CARTESIAN_POINT('',(18.18,35.08,7.2));
#75591=CARTESIAN_POINT('',(18.3,35.08,7.2));
#75592=CARTESIAN_POINT('',(18.18,34.92,7.2));
#75593=CARTESIAN_POINT('',(18.18,34.92,7.2));
#75594=CARTESIAN_POINT('',(18.3,34.92,7.2));
#75595=CARTESIAN_POINT('Origin',(18.3,35.08,9.4));
#75596=CARTESIAN_POINT('',(18.3,35.08,9.4));
#75597=CARTESIAN_POINT('',(18.3,35.08,7.45));
#75598=CARTESIAN_POINT('',(18.18,35.08,9.4));
#75599=CARTESIAN_POINT('',(18.3,35.08,9.4));
#75600=CARTESIAN_POINT('',(18.18,35.08,7.2));
#75601=CARTESIAN_POINT('Origin',(18.3,34.92,9.4));
#75602=CARTESIAN_POINT('',(18.3,34.92,9.4));
#75603=CARTESIAN_POINT('',(18.3,52.46,9.4));
#75604=CARTESIAN_POINT('',(18.18,34.92,9.4));
#75605=CARTESIAN_POINT('',(18.3,34.92,9.4));
#75606=CARTESIAN_POINT('',(18.18,35.08,9.4));
#75607=CARTESIAN_POINT('Origin',(18.3,34.92,7.2));
#75608=CARTESIAN_POINT('',(18.3,34.92,6.35));
#75609=CARTESIAN_POINT('',(18.18,34.92,9.4));
#75610=CARTESIAN_POINT('Origin',(18.18,35.,8.3));
#75611=CARTESIAN_POINT('Origin',(18.3,37.08,8.));
#75612=CARTESIAN_POINT('',(18.3,37.08,8.));
#75613=CARTESIAN_POINT('',(18.3,36.92,8.));
#75614=CARTESIAN_POINT('',(18.3,53.54,8.));
#75615=CARTESIAN_POINT('',(18.18,37.08,8.));
#75616=CARTESIAN_POINT('',(18.3,37.08,8.));
#75617=CARTESIAN_POINT('',(18.18,36.92,8.));
#75618=CARTESIAN_POINT('',(18.18,36.92,8.));
#75619=CARTESIAN_POINT('',(18.3,36.92,8.));
#75620=CARTESIAN_POINT('Origin',(18.3,37.08,9.4));
#75621=CARTESIAN_POINT('',(18.3,37.08,9.4));
#75622=CARTESIAN_POINT('',(18.3,37.08,7.45));
#75623=CARTESIAN_POINT('',(18.18,37.08,9.4));
#75624=CARTESIAN_POINT('',(18.3,37.08,9.4));
#75625=CARTESIAN_POINT('',(18.18,37.08,8.));
#75626=CARTESIAN_POINT('Origin',(18.3,36.92,9.4));
#75627=CARTESIAN_POINT('',(18.3,36.92,9.4));
#75628=CARTESIAN_POINT('',(18.3,53.46,9.4));
#75629=CARTESIAN_POINT('',(18.18,36.92,9.4));
#75630=CARTESIAN_POINT('',(18.3,36.92,9.4));
#75631=CARTESIAN_POINT('',(18.18,37.08,9.4));
#75632=CARTESIAN_POINT('Origin',(18.3,36.92,8.));
#75633=CARTESIAN_POINT('',(18.3,36.92,6.75));
#75634=CARTESIAN_POINT('',(18.18,36.92,9.4));
#75635=CARTESIAN_POINT('Origin',(18.18,37.,8.7));
#75636=CARTESIAN_POINT('Origin',(18.3,39.08,8.));
#75637=CARTESIAN_POINT('',(18.3,39.08,8.));
#75638=CARTESIAN_POINT('',(18.3,38.92,8.));
#75639=CARTESIAN_POINT('',(18.3,54.54,8.));
#75640=CARTESIAN_POINT('',(18.18,39.08,8.));
#75641=CARTESIAN_POINT('',(18.3,39.08,8.));
#75642=CARTESIAN_POINT('',(18.18,38.92,8.));
#75643=CARTESIAN_POINT('',(18.18,38.92,8.));
#75644=CARTESIAN_POINT('',(18.3,38.92,8.));
#75645=CARTESIAN_POINT('Origin',(18.3,39.08,9.4));
#75646=CARTESIAN_POINT('',(18.3,39.08,9.4));
#75647=CARTESIAN_POINT('',(18.3,39.08,7.45));
#75648=CARTESIAN_POINT('',(18.18,39.08,9.4));
#75649=CARTESIAN_POINT('',(18.3,39.08,9.4));
#75650=CARTESIAN_POINT('',(18.18,39.08,8.));
#75651=CARTESIAN_POINT('Origin',(18.3,38.92,9.4));
#75652=CARTESIAN_POINT('',(18.3,38.92,9.4));
#75653=CARTESIAN_POINT('',(18.3,54.46,9.4));
#75654=CARTESIAN_POINT('',(18.18,38.92,9.4));
#75655=CARTESIAN_POINT('',(18.3,38.92,9.4));
#75656=CARTESIAN_POINT('',(18.18,39.08,9.4));
#75657=CARTESIAN_POINT('Origin',(18.3,38.92,8.));
#75658=CARTESIAN_POINT('',(18.3,38.92,6.75));
#75659=CARTESIAN_POINT('',(18.18,38.92,9.4));
#75660=CARTESIAN_POINT('Origin',(18.18,39.,8.7));
#75661=CARTESIAN_POINT('Origin',(18.3,41.08,8.));
#75662=CARTESIAN_POINT('',(18.3,41.08,8.));
#75663=CARTESIAN_POINT('',(18.3,40.92,8.));
#75664=CARTESIAN_POINT('',(18.3,55.54,8.));
#75665=CARTESIAN_POINT('',(18.18,41.08,8.));
#75666=CARTESIAN_POINT('',(18.3,41.08,8.));
#75667=CARTESIAN_POINT('',(18.18,40.92,8.));
#75668=CARTESIAN_POINT('',(18.18,40.92,8.));
#75669=CARTESIAN_POINT('',(18.3,40.92,8.));
#75670=CARTESIAN_POINT('Origin',(18.3,41.08,9.4));
#75671=CARTESIAN_POINT('',(18.3,41.08,9.4));
#75672=CARTESIAN_POINT('',(18.3,41.08,7.45));
#75673=CARTESIAN_POINT('',(18.18,41.08,9.4));
#75674=CARTESIAN_POINT('',(18.3,41.08,9.4));
#75675=CARTESIAN_POINT('',(18.18,41.08,8.));
#75676=CARTESIAN_POINT('Origin',(18.3,40.92,9.4));
#75677=CARTESIAN_POINT('',(18.3,40.92,9.4));
#75678=CARTESIAN_POINT('',(18.3,55.46,9.4));
#75679=CARTESIAN_POINT('',(18.18,40.92,9.4));
#75680=CARTESIAN_POINT('',(18.3,40.92,9.4));
#75681=CARTESIAN_POINT('',(18.18,41.08,9.4));
#75682=CARTESIAN_POINT('Origin',(18.3,40.92,8.));
#75683=CARTESIAN_POINT('',(18.3,40.92,6.75));
#75684=CARTESIAN_POINT('',(18.18,40.92,9.4));
#75685=CARTESIAN_POINT('Origin',(18.18,41.,8.7));
#75686=CARTESIAN_POINT('Origin',(18.3,43.08,8.));
#75687=CARTESIAN_POINT('',(18.3,43.08,8.));
#75688=CARTESIAN_POINT('',(18.3,42.92,8.));
#75689=CARTESIAN_POINT('',(18.3,56.54,8.));
#75690=CARTESIAN_POINT('',(18.18,43.08,8.));
#75691=CARTESIAN_POINT('',(18.3,43.08,8.));
#75692=CARTESIAN_POINT('',(18.18,42.92,8.));
#75693=CARTESIAN_POINT('',(18.18,42.92,8.));
#75694=CARTESIAN_POINT('',(18.3,42.92,8.));
#75695=CARTESIAN_POINT('Origin',(18.3,43.08,9.4));
#75696=CARTESIAN_POINT('',(18.3,43.08,9.4));
#75697=CARTESIAN_POINT('',(18.3,43.08,7.45));
#75698=CARTESIAN_POINT('',(18.18,43.08,9.4));
#75699=CARTESIAN_POINT('',(18.3,43.08,9.4));
#75700=CARTESIAN_POINT('',(18.18,43.08,8.));
#75701=CARTESIAN_POINT('Origin',(18.3,42.92,9.4));
#75702=CARTESIAN_POINT('',(18.3,42.92,9.4));
#75703=CARTESIAN_POINT('',(18.3,56.46,9.4));
#75704=CARTESIAN_POINT('',(18.18,42.92,9.4));
#75705=CARTESIAN_POINT('',(18.3,42.92,9.4));
#75706=CARTESIAN_POINT('',(18.18,43.08,9.4));
#75707=CARTESIAN_POINT('Origin',(18.3,42.92,8.));
#75708=CARTESIAN_POINT('',(18.3,42.92,6.75));
#75709=CARTESIAN_POINT('',(18.18,42.92,9.4));
#75710=CARTESIAN_POINT('Origin',(18.18,43.,8.7));
#75711=CARTESIAN_POINT('Origin',(18.3,45.08,7.2));
#75712=CARTESIAN_POINT('',(18.3,45.08,7.2));
#75713=CARTESIAN_POINT('',(18.3,44.92,7.2));
#75714=CARTESIAN_POINT('',(18.3,57.54,7.2));
#75715=CARTESIAN_POINT('',(18.18,45.08,7.2));
#75716=CARTESIAN_POINT('',(18.3,45.08,7.2));
#75717=CARTESIAN_POINT('',(18.18,44.92,7.2));
#75718=CARTESIAN_POINT('',(18.18,44.92,7.2));
#75719=CARTESIAN_POINT('',(18.3,44.92,7.2));
#75720=CARTESIAN_POINT('Origin',(18.3,45.08,9.4));
#75721=CARTESIAN_POINT('',(18.3,45.08,9.4));
#75722=CARTESIAN_POINT('',(18.3,45.08,7.45));
#75723=CARTESIAN_POINT('',(18.18,45.08,9.4));
#75724=CARTESIAN_POINT('',(18.3,45.08,9.4));
#75725=CARTESIAN_POINT('',(18.18,45.08,7.2));
#75726=CARTESIAN_POINT('Origin',(18.3,44.92,9.4));
#75727=CARTESIAN_POINT('',(18.3,44.92,9.4));
#75728=CARTESIAN_POINT('',(18.3,57.46,9.4));
#75729=CARTESIAN_POINT('',(18.18,44.92,9.4));
#75730=CARTESIAN_POINT('',(18.3,44.92,9.4));
#75731=CARTESIAN_POINT('',(18.18,45.08,9.4));
#75732=CARTESIAN_POINT('Origin',(18.3,44.92,7.2));
#75733=CARTESIAN_POINT('',(18.3,44.92,6.35));
#75734=CARTESIAN_POINT('',(18.18,44.92,9.4));
#75735=CARTESIAN_POINT('Origin',(18.18,45.,8.3));
#75736=CARTESIAN_POINT('Origin',(18.3,47.08,8.));
#75737=CARTESIAN_POINT('',(18.3,47.08,8.));
#75738=CARTESIAN_POINT('',(18.3,46.92,8.));
#75739=CARTESIAN_POINT('',(18.3,58.54,8.));
#75740=CARTESIAN_POINT('',(18.18,47.08,8.));
#75741=CARTESIAN_POINT('',(18.3,47.08,8.));
#75742=CARTESIAN_POINT('',(18.18,46.92,8.));
#75743=CARTESIAN_POINT('',(18.18,46.92,8.));
#75744=CARTESIAN_POINT('',(18.3,46.92,8.));
#75745=CARTESIAN_POINT('Origin',(18.3,47.08,9.4));
#75746=CARTESIAN_POINT('',(18.3,47.08,9.4));
#75747=CARTESIAN_POINT('',(18.3,47.08,7.45));
#75748=CARTESIAN_POINT('',(18.18,47.08,9.4));
#75749=CARTESIAN_POINT('',(18.3,47.08,9.4));
#75750=CARTESIAN_POINT('',(18.18,47.08,8.));
#75751=CARTESIAN_POINT('Origin',(18.3,46.92,9.4));
#75752=CARTESIAN_POINT('',(18.3,46.92,9.4));
#75753=CARTESIAN_POINT('',(18.3,58.46,9.4));
#75754=CARTESIAN_POINT('',(18.18,46.92,9.4));
#75755=CARTESIAN_POINT('',(18.3,46.92,9.4));
#75756=CARTESIAN_POINT('',(18.18,47.08,9.4));
#75757=CARTESIAN_POINT('Origin',(18.3,46.92,8.));
#75758=CARTESIAN_POINT('',(18.3,46.92,6.75));
#75759=CARTESIAN_POINT('',(18.18,46.92,9.4));
#75760=CARTESIAN_POINT('Origin',(18.18,47.,8.7));
#75761=CARTESIAN_POINT('Origin',(18.3,49.08,8.));
#75762=CARTESIAN_POINT('',(18.3,49.08,8.));
#75763=CARTESIAN_POINT('',(18.3,48.92,8.));
#75764=CARTESIAN_POINT('',(18.3,59.54,8.));
#75765=CARTESIAN_POINT('',(18.18,49.08,8.));
#75766=CARTESIAN_POINT('',(18.3,49.08,8.));
#75767=CARTESIAN_POINT('',(18.18,48.92,8.));
#75768=CARTESIAN_POINT('',(18.18,48.92,8.));
#75769=CARTESIAN_POINT('',(18.3,48.92,8.));
#75770=CARTESIAN_POINT('Origin',(18.3,49.08,9.4));
#75771=CARTESIAN_POINT('',(18.3,49.08,9.4));
#75772=CARTESIAN_POINT('',(18.3,49.08,7.45));
#75773=CARTESIAN_POINT('',(18.18,49.08,9.4));
#75774=CARTESIAN_POINT('',(18.3,49.08,9.4));
#75775=CARTESIAN_POINT('',(18.18,49.08,8.));
#75776=CARTESIAN_POINT('Origin',(18.3,48.92,9.4));
#75777=CARTESIAN_POINT('',(18.3,48.92,9.4));
#75778=CARTESIAN_POINT('',(18.3,59.46,9.4));
#75779=CARTESIAN_POINT('',(18.18,48.92,9.4));
#75780=CARTESIAN_POINT('',(18.3,48.92,9.4));
#75781=CARTESIAN_POINT('',(18.18,49.08,9.4));
#75782=CARTESIAN_POINT('Origin',(18.3,48.92,8.));
#75783=CARTESIAN_POINT('',(18.3,48.92,6.75));
#75784=CARTESIAN_POINT('',(18.18,48.92,9.4));
#75785=CARTESIAN_POINT('Origin',(18.18,49.,8.7));
#75786=CARTESIAN_POINT('Origin',(18.3,51.08,8.));
#75787=CARTESIAN_POINT('',(18.3,51.08,8.));
#75788=CARTESIAN_POINT('',(18.3,50.92,8.));
#75789=CARTESIAN_POINT('',(18.3,60.54,8.));
#75790=CARTESIAN_POINT('',(18.18,51.08,8.));
#75791=CARTESIAN_POINT('',(18.3,51.08,8.));
#75792=CARTESIAN_POINT('',(18.18,50.92,8.));
#75793=CARTESIAN_POINT('',(18.18,50.92,8.));
#75794=CARTESIAN_POINT('',(18.3,50.92,8.));
#75795=CARTESIAN_POINT('Origin',(18.3,51.08,9.4));
#75796=CARTESIAN_POINT('',(18.3,51.08,9.4));
#75797=CARTESIAN_POINT('',(18.3,51.08,7.45));
#75798=CARTESIAN_POINT('',(18.18,51.08,9.4));
#75799=CARTESIAN_POINT('',(18.3,51.08,9.4));
#75800=CARTESIAN_POINT('',(18.18,51.08,8.));
#75801=CARTESIAN_POINT('Origin',(18.3,50.92,9.4));
#75802=CARTESIAN_POINT('',(18.3,50.92,9.4));
#75803=CARTESIAN_POINT('',(18.3,60.46,9.4));
#75804=CARTESIAN_POINT('',(18.18,50.92,9.4));
#75805=CARTESIAN_POINT('',(18.3,50.92,9.4));
#75806=CARTESIAN_POINT('',(18.18,51.08,9.4));
#75807=CARTESIAN_POINT('Origin',(18.3,50.92,8.));
#75808=CARTESIAN_POINT('',(18.3,50.92,6.75));
#75809=CARTESIAN_POINT('',(18.18,50.92,9.4));
#75810=CARTESIAN_POINT('Origin',(18.18,51.,8.7));
#75811=CARTESIAN_POINT('Origin',(18.3,53.08,8.));
#75812=CARTESIAN_POINT('',(18.3,53.08,8.));
#75813=CARTESIAN_POINT('',(18.3,52.92,8.));
#75814=CARTESIAN_POINT('',(18.3,61.54,8.));
#75815=CARTESIAN_POINT('',(18.18,53.08,8.));
#75816=CARTESIAN_POINT('',(18.3,53.08,8.));
#75817=CARTESIAN_POINT('',(18.18,52.92,8.));
#75818=CARTESIAN_POINT('',(18.18,52.92,8.));
#75819=CARTESIAN_POINT('',(18.3,52.92,8.));
#75820=CARTESIAN_POINT('Origin',(18.3,53.08,9.4));
#75821=CARTESIAN_POINT('',(18.3,53.08,9.4));
#75822=CARTESIAN_POINT('',(18.3,53.08,7.45));
#75823=CARTESIAN_POINT('',(18.18,53.08,9.4));
#75824=CARTESIAN_POINT('',(18.3,53.08,9.4));
#75825=CARTESIAN_POINT('',(18.18,53.08,8.));
#75826=CARTESIAN_POINT('Origin',(18.3,52.92,9.4));
#75827=CARTESIAN_POINT('',(18.3,52.92,9.4));
#75828=CARTESIAN_POINT('',(18.3,61.46,9.4));
#75829=CARTESIAN_POINT('',(18.18,52.92,9.4));
#75830=CARTESIAN_POINT('',(18.3,52.92,9.4));
#75831=CARTESIAN_POINT('',(18.18,53.08,9.4));
#75832=CARTESIAN_POINT('Origin',(18.3,52.92,8.));
#75833=CARTESIAN_POINT('',(18.3,52.92,6.75));
#75834=CARTESIAN_POINT('',(18.18,52.92,9.4));
#75835=CARTESIAN_POINT('Origin',(18.18,53.,8.7));
#75836=CARTESIAN_POINT('Origin',(18.3,55.08,7.2));
#75837=CARTESIAN_POINT('',(18.3,55.08,7.2));
#75838=CARTESIAN_POINT('',(18.3,54.92,7.2));
#75839=CARTESIAN_POINT('',(18.3,62.54,7.2));
#75840=CARTESIAN_POINT('',(18.18,55.08,7.2));
#75841=CARTESIAN_POINT('',(18.3,55.08,7.2));
#75842=CARTESIAN_POINT('',(18.18,54.92,7.2));
#75843=CARTESIAN_POINT('',(18.18,54.92,7.2));
#75844=CARTESIAN_POINT('',(18.3,54.92,7.2));
#75845=CARTESIAN_POINT('Origin',(18.3,55.08,9.4));
#75846=CARTESIAN_POINT('',(18.3,55.08,9.4));
#75847=CARTESIAN_POINT('',(18.3,55.08,7.45));
#75848=CARTESIAN_POINT('',(18.18,55.08,9.4));
#75849=CARTESIAN_POINT('',(18.3,55.08,9.4));
#75850=CARTESIAN_POINT('',(18.18,55.08,7.2));
#75851=CARTESIAN_POINT('Origin',(18.3,54.92,9.4));
#75852=CARTESIAN_POINT('',(18.3,54.92,9.4));
#75853=CARTESIAN_POINT('',(18.3,62.46,9.4));
#75854=CARTESIAN_POINT('',(18.18,54.92,9.4));
#75855=CARTESIAN_POINT('',(18.3,54.92,9.4));
#75856=CARTESIAN_POINT('',(18.18,55.08,9.4));
#75857=CARTESIAN_POINT('Origin',(18.3,54.92,7.2));
#75858=CARTESIAN_POINT('',(18.3,54.92,6.35));
#75859=CARTESIAN_POINT('',(18.18,54.92,9.4));
#75860=CARTESIAN_POINT('Origin',(18.18,55.,8.3));
#75861=CARTESIAN_POINT('Origin',(18.3,57.08,8.));
#75862=CARTESIAN_POINT('',(18.3,57.08,8.));
#75863=CARTESIAN_POINT('',(18.3,56.92,8.));
#75864=CARTESIAN_POINT('',(18.3,63.54,8.));
#75865=CARTESIAN_POINT('',(18.18,57.08,8.));
#75866=CARTESIAN_POINT('',(18.3,57.08,8.));
#75867=CARTESIAN_POINT('',(18.18,56.92,8.));
#75868=CARTESIAN_POINT('',(18.18,56.92,8.));
#75869=CARTESIAN_POINT('',(18.3,56.92,8.));
#75870=CARTESIAN_POINT('Origin',(18.3,57.08,9.4));
#75871=CARTESIAN_POINT('',(18.3,57.08,9.4));
#75872=CARTESIAN_POINT('',(18.3,57.08,7.45));
#75873=CARTESIAN_POINT('',(18.18,57.08,9.4));
#75874=CARTESIAN_POINT('',(18.3,57.08,9.4));
#75875=CARTESIAN_POINT('',(18.18,57.08,8.));
#75876=CARTESIAN_POINT('Origin',(18.3,56.92,9.4));
#75877=CARTESIAN_POINT('',(18.3,56.92,9.4));
#75878=CARTESIAN_POINT('',(18.3,63.46,9.4));
#75879=CARTESIAN_POINT('',(18.18,56.92,9.4));
#75880=CARTESIAN_POINT('',(18.3,56.92,9.4));
#75881=CARTESIAN_POINT('',(18.18,57.08,9.4));
#75882=CARTESIAN_POINT('Origin',(18.3,56.92,8.));
#75883=CARTESIAN_POINT('',(18.3,56.92,6.75));
#75884=CARTESIAN_POINT('',(18.18,56.92,9.4));
#75885=CARTESIAN_POINT('Origin',(18.18,57.,8.7));
#75886=CARTESIAN_POINT('Origin',(18.3,59.08,8.));
#75887=CARTESIAN_POINT('',(18.3,59.08,8.));
#75888=CARTESIAN_POINT('',(18.3,58.92,8.));
#75889=CARTESIAN_POINT('',(18.3,64.54,8.));
#75890=CARTESIAN_POINT('',(18.18,59.08,8.));
#75891=CARTESIAN_POINT('',(18.3,59.08,8.));
#75892=CARTESIAN_POINT('',(18.18,58.92,8.));
#75893=CARTESIAN_POINT('',(18.18,58.92,8.));
#75894=CARTESIAN_POINT('',(18.3,58.92,8.));
#75895=CARTESIAN_POINT('Origin',(18.3,59.08,9.4));
#75896=CARTESIAN_POINT('',(18.3,59.08,9.4));
#75897=CARTESIAN_POINT('',(18.3,59.08,7.45));
#75898=CARTESIAN_POINT('',(18.18,59.08,9.4));
#75899=CARTESIAN_POINT('',(18.3,59.08,9.4));
#75900=CARTESIAN_POINT('',(18.18,59.08,8.));
#75901=CARTESIAN_POINT('Origin',(18.3,58.92,9.4));
#75902=CARTESIAN_POINT('',(18.3,58.92,9.4));
#75903=CARTESIAN_POINT('',(18.3,64.46,9.4));
#75904=CARTESIAN_POINT('',(18.18,58.92,9.4));
#75905=CARTESIAN_POINT('',(18.3,58.92,9.4));
#75906=CARTESIAN_POINT('',(18.18,59.08,9.4));
#75907=CARTESIAN_POINT('Origin',(18.3,58.92,8.));
#75908=CARTESIAN_POINT('',(18.3,58.92,6.75));
#75909=CARTESIAN_POINT('',(18.18,58.92,9.4));
#75910=CARTESIAN_POINT('Origin',(18.18,59.,8.7));
#75911=CARTESIAN_POINT('Origin',(18.3,61.08,8.));
#75912=CARTESIAN_POINT('',(18.3,61.08,8.));
#75913=CARTESIAN_POINT('',(18.3,60.92,8.));
#75914=CARTESIAN_POINT('',(18.3,65.54,8.));
#75915=CARTESIAN_POINT('',(18.18,61.08,8.));
#75916=CARTESIAN_POINT('',(18.3,61.08,8.));
#75917=CARTESIAN_POINT('',(18.18,60.92,8.));
#75918=CARTESIAN_POINT('',(18.18,60.92,8.));
#75919=CARTESIAN_POINT('',(18.3,60.92,8.));
#75920=CARTESIAN_POINT('Origin',(18.3,61.08,9.4));
#75921=CARTESIAN_POINT('',(18.3,61.08,9.4));
#75922=CARTESIAN_POINT('',(18.3,61.08,7.45));
#75923=CARTESIAN_POINT('',(18.18,61.08,9.4));
#75924=CARTESIAN_POINT('',(18.3,61.08,9.4));
#75925=CARTESIAN_POINT('',(18.18,61.08,8.));
#75926=CARTESIAN_POINT('Origin',(18.3,60.92,9.4));
#75927=CARTESIAN_POINT('',(18.3,60.92,9.4));
#75928=CARTESIAN_POINT('',(18.3,65.46,9.4));
#75929=CARTESIAN_POINT('',(18.18,60.92,9.4));
#75930=CARTESIAN_POINT('',(18.3,60.92,9.4));
#75931=CARTESIAN_POINT('',(18.18,61.08,9.4));
#75932=CARTESIAN_POINT('Origin',(18.3,60.92,8.));
#75933=CARTESIAN_POINT('',(18.3,60.92,6.75));
#75934=CARTESIAN_POINT('',(18.18,60.92,9.4));
#75935=CARTESIAN_POINT('Origin',(18.18,61.,8.7));
#75936=CARTESIAN_POINT('Origin',(18.3,63.08,8.));
#75937=CARTESIAN_POINT('',(18.3,63.08,8.));
#75938=CARTESIAN_POINT('',(18.3,62.92,8.));
#75939=CARTESIAN_POINT('',(18.3,66.54,8.));
#75940=CARTESIAN_POINT('',(18.18,63.08,8.));
#75941=CARTESIAN_POINT('',(18.3,63.08,8.));
#75942=CARTESIAN_POINT('',(18.18,62.92,8.));
#75943=CARTESIAN_POINT('',(18.18,62.92,8.));
#75944=CARTESIAN_POINT('',(18.3,62.92,8.));
#75945=CARTESIAN_POINT('Origin',(18.3,63.08,9.4));
#75946=CARTESIAN_POINT('',(18.3,63.08,9.4));
#75947=CARTESIAN_POINT('',(18.3,63.08,7.45));
#75948=CARTESIAN_POINT('',(18.18,63.08,9.4));
#75949=CARTESIAN_POINT('',(18.3,63.08,9.4));
#75950=CARTESIAN_POINT('',(18.18,63.08,8.));
#75951=CARTESIAN_POINT('Origin',(18.3,62.92,9.4));
#75952=CARTESIAN_POINT('',(18.3,62.92,9.4));
#75953=CARTESIAN_POINT('',(18.3,66.46,9.4));
#75954=CARTESIAN_POINT('',(18.18,62.92,9.4));
#75955=CARTESIAN_POINT('',(18.3,62.92,9.4));
#75956=CARTESIAN_POINT('',(18.18,63.08,9.4));
#75957=CARTESIAN_POINT('Origin',(18.3,62.92,8.));
#75958=CARTESIAN_POINT('',(18.3,62.92,6.75));
#75959=CARTESIAN_POINT('',(18.18,62.92,9.4));
#75960=CARTESIAN_POINT('Origin',(18.18,63.,8.7));
#75961=CARTESIAN_POINT('Origin',(18.3,65.08,7.2));
#75962=CARTESIAN_POINT('',(18.3,65.08,7.2));
#75963=CARTESIAN_POINT('',(18.3,64.92,7.2));
#75964=CARTESIAN_POINT('',(18.3,67.54,7.2));
#75965=CARTESIAN_POINT('',(18.18,65.08,7.2));
#75966=CARTESIAN_POINT('',(18.3,65.08,7.2));
#75967=CARTESIAN_POINT('',(18.18,64.92,7.2));
#75968=CARTESIAN_POINT('',(18.18,64.92,7.2));
#75969=CARTESIAN_POINT('',(18.3,64.92,7.2));
#75970=CARTESIAN_POINT('Origin',(18.3,65.08,9.4));
#75971=CARTESIAN_POINT('',(18.3,65.08,9.4));
#75972=CARTESIAN_POINT('',(18.3,65.08,7.45));
#75973=CARTESIAN_POINT('',(18.18,65.08,9.4));
#75974=CARTESIAN_POINT('',(18.3,65.08,9.4));
#75975=CARTESIAN_POINT('',(18.18,65.08,7.2));
#75976=CARTESIAN_POINT('Origin',(18.3,64.92,9.4));
#75977=CARTESIAN_POINT('',(18.3,64.92,9.4));
#75978=CARTESIAN_POINT('',(18.3,67.46,9.4));
#75979=CARTESIAN_POINT('',(18.18,64.92,9.4));
#75980=CARTESIAN_POINT('',(18.3,64.92,9.4));
#75981=CARTESIAN_POINT('',(18.18,65.08,9.4));
#75982=CARTESIAN_POINT('Origin',(18.3,64.92,7.2));
#75983=CARTESIAN_POINT('',(18.3,64.92,6.35));
#75984=CARTESIAN_POINT('',(18.18,64.92,9.4));
#75985=CARTESIAN_POINT('Origin',(18.18,65.,8.3));
#75986=CARTESIAN_POINT('Origin',(18.3,67.08,8.));
#75987=CARTESIAN_POINT('',(18.3,67.08,8.));
#75988=CARTESIAN_POINT('',(18.3,66.92,8.));
#75989=CARTESIAN_POINT('',(18.3,68.54,8.));
#75990=CARTESIAN_POINT('',(18.18,67.08,8.));
#75991=CARTESIAN_POINT('',(18.3,67.08,8.));
#75992=CARTESIAN_POINT('',(18.18,66.92,8.));
#75993=CARTESIAN_POINT('',(18.18,66.92,8.));
#75994=CARTESIAN_POINT('',(18.3,66.92,8.));
#75995=CARTESIAN_POINT('Origin',(18.3,67.08,9.4));
#75996=CARTESIAN_POINT('',(18.3,67.08,9.4));
#75997=CARTESIAN_POINT('',(18.3,67.08,7.45));
#75998=CARTESIAN_POINT('',(18.18,67.08,9.4));
#75999=CARTESIAN_POINT('',(18.3,67.08,9.4));
#76000=CARTESIAN_POINT('',(18.18,67.08,8.));
#76001=CARTESIAN_POINT('Origin',(18.3,66.92,9.4));
#76002=CARTESIAN_POINT('',(18.3,66.92,9.4));
#76003=CARTESIAN_POINT('',(18.3,68.46,9.4));
#76004=CARTESIAN_POINT('',(18.18,66.92,9.4));
#76005=CARTESIAN_POINT('',(18.3,66.92,9.4));
#76006=CARTESIAN_POINT('',(18.18,67.08,9.4));
#76007=CARTESIAN_POINT('Origin',(18.3,66.92,8.));
#76008=CARTESIAN_POINT('',(18.3,66.92,6.75));
#76009=CARTESIAN_POINT('',(18.18,66.92,9.4));
#76010=CARTESIAN_POINT('Origin',(18.18,67.,8.7));
#76011=CARTESIAN_POINT('Origin',(18.3,69.08,8.));
#76012=CARTESIAN_POINT('',(18.3,69.08,8.));
#76013=CARTESIAN_POINT('',(18.3,68.92,8.));
#76014=CARTESIAN_POINT('',(18.3,69.54,8.));
#76015=CARTESIAN_POINT('',(18.18,69.08,8.));
#76016=CARTESIAN_POINT('',(18.3,69.08,8.));
#76017=CARTESIAN_POINT('',(18.18,68.92,8.));
#76018=CARTESIAN_POINT('',(18.18,68.92,8.));
#76019=CARTESIAN_POINT('',(18.3,68.92,8.));
#76020=CARTESIAN_POINT('Origin',(18.3,69.08,9.4));
#76021=CARTESIAN_POINT('',(18.3,69.08,9.4));
#76022=CARTESIAN_POINT('',(18.3,69.08,7.45));
#76023=CARTESIAN_POINT('',(18.18,69.08,9.4));
#76024=CARTESIAN_POINT('',(18.3,69.08,9.4));
#76025=CARTESIAN_POINT('',(18.18,69.08,8.));
#76026=CARTESIAN_POINT('Origin',(18.3,68.92,9.4));
#76027=CARTESIAN_POINT('',(18.3,68.92,9.4));
#76028=CARTESIAN_POINT('',(18.3,69.46,9.4));
#76029=CARTESIAN_POINT('',(18.18,68.92,9.4));
#76030=CARTESIAN_POINT('',(18.3,68.92,9.4));
#76031=CARTESIAN_POINT('',(18.18,69.08,9.4));
#76032=CARTESIAN_POINT('Origin',(18.3,68.92,8.));
#76033=CARTESIAN_POINT('',(18.3,68.92,6.75));
#76034=CARTESIAN_POINT('',(18.18,68.92,9.4));
#76035=CARTESIAN_POINT('Origin',(18.18,69.,8.7));
#76036=CARTESIAN_POINT('Origin',(18.3,28.08,8.));
#76037=CARTESIAN_POINT('',(18.3,28.08,8.));
#76038=CARTESIAN_POINT('',(18.3,27.92,8.));
#76039=CARTESIAN_POINT('',(18.3,49.04,8.));
#76040=CARTESIAN_POINT('',(18.18,28.08,8.));
#76041=CARTESIAN_POINT('',(18.3,28.08,8.));
#76042=CARTESIAN_POINT('',(18.18,27.92,8.));
#76043=CARTESIAN_POINT('',(18.18,27.92,8.));
#76044=CARTESIAN_POINT('',(18.3,27.92,8.));
#76045=CARTESIAN_POINT('Origin',(18.3,28.08,9.4));
#76046=CARTESIAN_POINT('',(18.3,28.08,9.4));
#76047=CARTESIAN_POINT('',(18.3,28.08,7.45));
#76048=CARTESIAN_POINT('',(18.18,28.08,9.4));
#76049=CARTESIAN_POINT('',(18.3,28.08,9.4));
#76050=CARTESIAN_POINT('',(18.18,28.08,8.));
#76051=CARTESIAN_POINT('Origin',(18.3,27.92,9.4));
#76052=CARTESIAN_POINT('',(18.3,27.92,9.4));
#76053=CARTESIAN_POINT('',(18.3,48.96,9.4));
#76054=CARTESIAN_POINT('',(18.18,27.92,9.4));
#76055=CARTESIAN_POINT('',(18.3,27.92,9.4));
#76056=CARTESIAN_POINT('',(18.18,28.08,9.4));
#76057=CARTESIAN_POINT('Origin',(18.3,27.92,8.));
#76058=CARTESIAN_POINT('',(18.3,27.92,6.75));
#76059=CARTESIAN_POINT('',(18.18,27.92,9.4));
#76060=CARTESIAN_POINT('Origin',(18.18,28.,8.7));
#76061=CARTESIAN_POINT('Origin',(18.3,72.08,8.));
#76062=CARTESIAN_POINT('',(18.3,72.08,8.));
#76063=CARTESIAN_POINT('',(18.3,71.92,8.));
#76064=CARTESIAN_POINT('',(18.3,71.04,8.));
#76065=CARTESIAN_POINT('',(18.18,72.08,8.));
#76066=CARTESIAN_POINT('',(18.3,72.08,8.));
#76067=CARTESIAN_POINT('',(18.18,71.92,8.));
#76068=CARTESIAN_POINT('',(18.18,71.92,8.));
#76069=CARTESIAN_POINT('',(18.3,71.92,8.));
#76070=CARTESIAN_POINT('Origin',(18.3,72.08,9.4));
#76071=CARTESIAN_POINT('',(18.3,72.08,9.4));
#76072=CARTESIAN_POINT('',(18.3,72.08,7.45));
#76073=CARTESIAN_POINT('',(18.18,72.08,9.4));
#76074=CARTESIAN_POINT('',(18.3,72.08,9.4));
#76075=CARTESIAN_POINT('',(18.18,72.08,8.));
#76076=CARTESIAN_POINT('Origin',(18.3,71.92,9.4));
#76077=CARTESIAN_POINT('',(18.3,71.92,9.4));
#76078=CARTESIAN_POINT('',(18.3,70.96,9.4));
#76079=CARTESIAN_POINT('',(18.18,71.92,9.4));
#76080=CARTESIAN_POINT('',(18.3,71.92,9.4));
#76081=CARTESIAN_POINT('',(18.18,72.08,9.4));
#76082=CARTESIAN_POINT('Origin',(18.3,71.92,8.));
#76083=CARTESIAN_POINT('',(18.3,71.92,6.75));
#76084=CARTESIAN_POINT('',(18.18,71.92,9.4));
#76085=CARTESIAN_POINT('Origin',(18.18,72.,8.7));
#76086=CARTESIAN_POINT('Origin',(18.3,74.08,8.));
#76087=CARTESIAN_POINT('',(18.3,74.08,8.));
#76088=CARTESIAN_POINT('',(18.3,73.92,8.));
#76089=CARTESIAN_POINT('',(18.3,72.04,8.));
#76090=CARTESIAN_POINT('',(18.18,74.08,8.));
#76091=CARTESIAN_POINT('',(18.3,74.08,8.));
#76092=CARTESIAN_POINT('',(18.18,73.92,8.));
#76093=CARTESIAN_POINT('',(18.18,73.92,8.));
#76094=CARTESIAN_POINT('',(18.3,73.92,8.));
#76095=CARTESIAN_POINT('Origin',(18.3,74.08,9.4));
#76096=CARTESIAN_POINT('',(18.3,74.08,9.4));
#76097=CARTESIAN_POINT('',(18.3,74.08,7.45));
#76098=CARTESIAN_POINT('',(18.18,74.08,9.4));
#76099=CARTESIAN_POINT('',(18.3,74.08,9.4));
#76100=CARTESIAN_POINT('',(18.18,74.08,8.));
#76101=CARTESIAN_POINT('Origin',(18.3,73.92,9.4));
#76102=CARTESIAN_POINT('',(18.3,73.92,9.4));
#76103=CARTESIAN_POINT('',(18.3,71.96,9.4));
#76104=CARTESIAN_POINT('',(18.18,73.92,9.4));
#76105=CARTESIAN_POINT('',(18.3,73.92,9.4));
#76106=CARTESIAN_POINT('',(18.18,74.08,9.4));
#76107=CARTESIAN_POINT('Origin',(18.3,73.92,8.));
#76108=CARTESIAN_POINT('',(18.3,73.92,6.75));
#76109=CARTESIAN_POINT('',(18.18,73.92,9.4));
#76110=CARTESIAN_POINT('Origin',(18.18,74.,8.7));
#76111=CARTESIAN_POINT('Origin',(18.3,76.08,8.));
#76112=CARTESIAN_POINT('',(18.3,76.08,8.));
#76113=CARTESIAN_POINT('',(18.3,75.92,8.));
#76114=CARTESIAN_POINT('',(18.3,73.04,8.));
#76115=CARTESIAN_POINT('',(18.18,76.08,8.));
#76116=CARTESIAN_POINT('',(18.3,76.08,8.));
#76117=CARTESIAN_POINT('',(18.18,75.92,8.));
#76118=CARTESIAN_POINT('',(18.18,75.92,8.));
#76119=CARTESIAN_POINT('',(18.3,75.92,8.));
#76120=CARTESIAN_POINT('Origin',(18.3,76.08,9.4));
#76121=CARTESIAN_POINT('',(18.3,76.08,9.4));
#76122=CARTESIAN_POINT('',(18.3,76.08,7.45));
#76123=CARTESIAN_POINT('',(18.18,76.08,9.4));
#76124=CARTESIAN_POINT('',(18.3,76.08,9.4));
#76125=CARTESIAN_POINT('',(18.18,76.08,8.));
#76126=CARTESIAN_POINT('Origin',(18.3,75.92,9.4));
#76127=CARTESIAN_POINT('',(18.3,75.92,9.4));
#76128=CARTESIAN_POINT('',(18.3,72.96,9.4));
#76129=CARTESIAN_POINT('',(18.18,75.92,9.4));
#76130=CARTESIAN_POINT('',(18.3,75.92,9.4));
#76131=CARTESIAN_POINT('',(18.18,76.08,9.4));
#76132=CARTESIAN_POINT('Origin',(18.3,75.92,8.));
#76133=CARTESIAN_POINT('',(18.3,75.92,6.75));
#76134=CARTESIAN_POINT('',(18.18,75.92,9.4));
#76135=CARTESIAN_POINT('Origin',(18.18,76.,8.7));
#76136=CARTESIAN_POINT('Origin',(18.3,78.08,8.));
#76137=CARTESIAN_POINT('',(18.3,78.08,8.));
#76138=CARTESIAN_POINT('',(18.3,77.92,8.));
#76139=CARTESIAN_POINT('',(18.3,74.04,8.));
#76140=CARTESIAN_POINT('',(18.18,78.08,8.));
#76141=CARTESIAN_POINT('',(18.3,78.08,8.));
#76142=CARTESIAN_POINT('',(18.18,77.92,8.));
#76143=CARTESIAN_POINT('',(18.18,77.92,8.));
#76144=CARTESIAN_POINT('',(18.3,77.92,8.));
#76145=CARTESIAN_POINT('Origin',(18.3,78.08,9.4));
#76146=CARTESIAN_POINT('',(18.3,78.08,9.4));
#76147=CARTESIAN_POINT('',(18.3,78.08,7.45));
#76148=CARTESIAN_POINT('',(18.18,78.08,9.4));
#76149=CARTESIAN_POINT('',(18.3,78.08,9.4));
#76150=CARTESIAN_POINT('',(18.18,78.08,8.));
#76151=CARTESIAN_POINT('Origin',(18.3,77.92,9.4));
#76152=CARTESIAN_POINT('',(18.3,77.92,9.4));
#76153=CARTESIAN_POINT('',(18.3,73.96,9.4));
#76154=CARTESIAN_POINT('',(18.18,77.92,9.4));
#76155=CARTESIAN_POINT('',(18.3,77.92,9.4));
#76156=CARTESIAN_POINT('',(18.18,78.08,9.4));
#76157=CARTESIAN_POINT('Origin',(18.3,77.92,8.));
#76158=CARTESIAN_POINT('',(18.3,77.92,6.75));
#76159=CARTESIAN_POINT('',(18.18,77.92,9.4));
#76160=CARTESIAN_POINT('Origin',(18.18,78.,8.7));
#76161=CARTESIAN_POINT('Origin',(18.3,80.08,6.4));
#76162=CARTESIAN_POINT('',(18.3,80.08,6.4));
#76163=CARTESIAN_POINT('',(18.3,79.92,6.4));
#76164=CARTESIAN_POINT('',(18.3,75.04,6.4));
#76165=CARTESIAN_POINT('',(18.18,80.08,6.4));
#76166=CARTESIAN_POINT('',(18.3,80.08,6.4));
#76167=CARTESIAN_POINT('',(18.18,79.92,6.4));
#76168=CARTESIAN_POINT('',(18.18,79.92,6.4));
#76169=CARTESIAN_POINT('',(18.3,79.92,6.4));
#76170=CARTESIAN_POINT('Origin',(18.3,80.08,9.4));
#76171=CARTESIAN_POINT('',(18.3,80.08,9.4));
#76172=CARTESIAN_POINT('',(18.3,80.08,7.45));
#76173=CARTESIAN_POINT('',(18.18,80.08,9.4));
#76174=CARTESIAN_POINT('',(18.3,80.08,9.4));
#76175=CARTESIAN_POINT('',(18.18,80.08,6.4));
#76176=CARTESIAN_POINT('Origin',(18.3,79.92,9.4));
#76177=CARTESIAN_POINT('',(18.3,79.92,9.4));
#76178=CARTESIAN_POINT('',(18.3,74.96,9.4));
#76179=CARTESIAN_POINT('',(18.18,79.92,9.4));
#76180=CARTESIAN_POINT('',(18.3,79.92,9.4));
#76181=CARTESIAN_POINT('',(18.18,80.08,9.4));
#76182=CARTESIAN_POINT('Origin',(18.3,79.92,6.4));
#76183=CARTESIAN_POINT('',(18.3,79.92,5.95));
#76184=CARTESIAN_POINT('',(18.18,79.92,9.4));
#76185=CARTESIAN_POINT('Origin',(18.18,80.,7.9));
#76186=CARTESIAN_POINT('Origin',(18.3,82.08,8.));
#76187=CARTESIAN_POINT('',(18.3,82.08,8.));
#76188=CARTESIAN_POINT('',(18.3,81.92,8.));
#76189=CARTESIAN_POINT('',(18.3,76.04,8.));
#76190=CARTESIAN_POINT('',(18.18,82.08,8.));
#76191=CARTESIAN_POINT('',(18.3,82.08,8.));
#76192=CARTESIAN_POINT('',(18.18,81.92,8.));
#76193=CARTESIAN_POINT('',(18.18,81.92,8.));
#76194=CARTESIAN_POINT('',(18.3,81.92,8.));
#76195=CARTESIAN_POINT('Origin',(18.3,82.08,9.4));
#76196=CARTESIAN_POINT('',(18.3,82.08,9.4));
#76197=CARTESIAN_POINT('',(18.3,82.08,7.45));
#76198=CARTESIAN_POINT('',(18.18,82.08,9.4));
#76199=CARTESIAN_POINT('',(18.3,82.08,9.4));
#76200=CARTESIAN_POINT('',(18.18,82.08,8.));
#76201=CARTESIAN_POINT('Origin',(18.3,81.92,9.4));
#76202=CARTESIAN_POINT('',(18.3,81.92,9.4));
#76203=CARTESIAN_POINT('',(18.3,75.96,9.4));
#76204=CARTESIAN_POINT('',(18.18,81.92,9.4));
#76205=CARTESIAN_POINT('',(18.3,81.92,9.4));
#76206=CARTESIAN_POINT('',(18.18,82.08,9.4));
#76207=CARTESIAN_POINT('Origin',(18.3,81.92,8.));
#76208=CARTESIAN_POINT('',(18.3,81.92,6.75));
#76209=CARTESIAN_POINT('',(18.18,81.92,9.4));
#76210=CARTESIAN_POINT('Origin',(18.18,82.,8.7));
#76211=CARTESIAN_POINT('Origin',(18.3,84.08,8.));
#76212=CARTESIAN_POINT('',(18.3,84.08,8.));
#76213=CARTESIAN_POINT('',(18.3,83.92,8.));
#76214=CARTESIAN_POINT('',(18.3,77.04,8.));
#76215=CARTESIAN_POINT('',(18.18,84.08,8.));
#76216=CARTESIAN_POINT('',(18.3,84.08,8.));
#76217=CARTESIAN_POINT('',(18.18,83.92,8.));
#76218=CARTESIAN_POINT('',(18.18,83.92,8.));
#76219=CARTESIAN_POINT('',(18.3,83.92,8.));
#76220=CARTESIAN_POINT('Origin',(18.3,84.08,9.4));
#76221=CARTESIAN_POINT('',(18.3,84.08,9.4));
#76222=CARTESIAN_POINT('',(18.3,84.08,7.45));
#76223=CARTESIAN_POINT('',(18.18,84.08,9.4));
#76224=CARTESIAN_POINT('',(18.3,84.08,9.4));
#76225=CARTESIAN_POINT('',(18.18,84.08,8.));
#76226=CARTESIAN_POINT('Origin',(18.3,83.92,9.4));
#76227=CARTESIAN_POINT('',(18.3,83.92,9.4));
#76228=CARTESIAN_POINT('',(18.3,76.96,9.4));
#76229=CARTESIAN_POINT('',(18.18,83.92,9.4));
#76230=CARTESIAN_POINT('',(18.3,83.92,9.4));
#76231=CARTESIAN_POINT('',(18.18,84.08,9.4));
#76232=CARTESIAN_POINT('Origin',(18.3,83.92,8.));
#76233=CARTESIAN_POINT('',(18.3,83.92,6.75));
#76234=CARTESIAN_POINT('',(18.18,83.92,9.4));
#76235=CARTESIAN_POINT('Origin',(18.18,84.,8.7));
#76236=CARTESIAN_POINT('Origin',(18.3,86.08,8.));
#76237=CARTESIAN_POINT('',(18.3,86.08,8.));
#76238=CARTESIAN_POINT('',(18.3,85.92,8.));
#76239=CARTESIAN_POINT('',(18.3,78.04,8.));
#76240=CARTESIAN_POINT('',(18.18,86.08,8.));
#76241=CARTESIAN_POINT('',(18.3,86.08,8.));
#76242=CARTESIAN_POINT('',(18.18,85.92,8.));
#76243=CARTESIAN_POINT('',(18.18,85.92,8.));
#76244=CARTESIAN_POINT('',(18.3,85.92,8.));
#76245=CARTESIAN_POINT('Origin',(18.3,86.08,9.4));
#76246=CARTESIAN_POINT('',(18.3,86.08,9.4));
#76247=CARTESIAN_POINT('',(18.3,86.08,7.45));
#76248=CARTESIAN_POINT('',(18.18,86.08,9.4));
#76249=CARTESIAN_POINT('',(18.3,86.08,9.4));
#76250=CARTESIAN_POINT('',(18.18,86.08,8.));
#76251=CARTESIAN_POINT('Origin',(18.3,85.92,9.4));
#76252=CARTESIAN_POINT('',(18.3,85.92,9.4));
#76253=CARTESIAN_POINT('',(18.3,77.96,9.4));
#76254=CARTESIAN_POINT('',(18.18,85.92,9.4));
#76255=CARTESIAN_POINT('',(18.3,85.92,9.4));
#76256=CARTESIAN_POINT('',(18.18,86.08,9.4));
#76257=CARTESIAN_POINT('Origin',(18.3,85.92,8.));
#76258=CARTESIAN_POINT('',(18.3,85.92,6.75));
#76259=CARTESIAN_POINT('',(18.18,85.92,9.4));
#76260=CARTESIAN_POINT('Origin',(18.18,86.,8.7));
#76261=CARTESIAN_POINT('Origin',(18.3,88.08,8.));
#76262=CARTESIAN_POINT('',(18.3,88.08,8.));
#76263=CARTESIAN_POINT('',(18.3,87.92,8.));
#76264=CARTESIAN_POINT('',(18.3,79.04,8.));
#76265=CARTESIAN_POINT('',(18.18,88.08,8.));
#76266=CARTESIAN_POINT('',(18.3,88.08,8.));
#76267=CARTESIAN_POINT('',(18.18,87.92,8.));
#76268=CARTESIAN_POINT('',(18.18,87.92,8.));
#76269=CARTESIAN_POINT('',(18.3,87.92,8.));
#76270=CARTESIAN_POINT('Origin',(18.3,88.08,9.4));
#76271=CARTESIAN_POINT('',(18.3,88.08,9.4));
#76272=CARTESIAN_POINT('',(18.3,88.08,7.45));
#76273=CARTESIAN_POINT('',(18.18,88.08,9.4));
#76274=CARTESIAN_POINT('',(18.3,88.08,9.4));
#76275=CARTESIAN_POINT('',(18.18,88.08,8.));
#76276=CARTESIAN_POINT('Origin',(18.3,87.92,9.4));
#76277=CARTESIAN_POINT('',(18.3,87.92,9.4));
#76278=CARTESIAN_POINT('',(18.3,78.96,9.4));
#76279=CARTESIAN_POINT('',(18.18,87.92,9.4));
#76280=CARTESIAN_POINT('',(18.3,87.92,9.4));
#76281=CARTESIAN_POINT('',(18.18,88.08,9.4));
#76282=CARTESIAN_POINT('Origin',(18.3,87.92,8.));
#76283=CARTESIAN_POINT('',(18.3,87.92,6.75));
#76284=CARTESIAN_POINT('',(18.18,87.92,9.4));
#76285=CARTESIAN_POINT('Origin',(18.18,88.,8.7));
#76286=CARTESIAN_POINT('Origin',(18.3,90.08,6.4));
#76287=CARTESIAN_POINT('',(18.3,90.08,6.4));
#76288=CARTESIAN_POINT('',(18.3,89.92,6.4));
#76289=CARTESIAN_POINT('',(18.3,80.04,6.4));
#76290=CARTESIAN_POINT('',(18.18,90.08,6.4));
#76291=CARTESIAN_POINT('',(18.3,90.08,6.4));
#76292=CARTESIAN_POINT('',(18.18,89.92,6.4));
#76293=CARTESIAN_POINT('',(18.18,89.92,6.4));
#76294=CARTESIAN_POINT('',(18.3,89.92,6.4));
#76295=CARTESIAN_POINT('Origin',(18.3,90.08,9.4));
#76296=CARTESIAN_POINT('',(18.3,90.08,9.4));
#76297=CARTESIAN_POINT('',(18.3,90.08,7.45));
#76298=CARTESIAN_POINT('',(18.18,90.08,9.4));
#76299=CARTESIAN_POINT('',(18.3,90.08,9.4));
#76300=CARTESIAN_POINT('',(18.18,90.08,6.4));
#76301=CARTESIAN_POINT('Origin',(18.3,89.92,9.4));
#76302=CARTESIAN_POINT('',(18.3,89.92,9.4));
#76303=CARTESIAN_POINT('',(18.3,79.96,9.4));
#76304=CARTESIAN_POINT('',(18.18,89.92,9.4));
#76305=CARTESIAN_POINT('',(18.3,89.92,9.4));
#76306=CARTESIAN_POINT('',(18.18,90.08,9.4));
#76307=CARTESIAN_POINT('Origin',(18.3,89.92,6.4));
#76308=CARTESIAN_POINT('',(18.3,89.92,5.95));
#76309=CARTESIAN_POINT('',(18.18,89.92,9.4));
#76310=CARTESIAN_POINT('Origin',(18.18,90.,7.9));
#76311=CARTESIAN_POINT('Origin',(18.3,92.08,8.));
#76312=CARTESIAN_POINT('',(18.3,92.08,8.));
#76313=CARTESIAN_POINT('',(18.3,91.92,8.));
#76314=CARTESIAN_POINT('',(18.3,81.04,8.));
#76315=CARTESIAN_POINT('',(18.18,92.08,8.));
#76316=CARTESIAN_POINT('',(18.3,92.08,8.));
#76317=CARTESIAN_POINT('',(18.18,91.92,8.));
#76318=CARTESIAN_POINT('',(18.18,91.92,8.));
#76319=CARTESIAN_POINT('',(18.3,91.92,8.));
#76320=CARTESIAN_POINT('Origin',(18.3,92.08,9.4));
#76321=CARTESIAN_POINT('',(18.3,92.08,9.4));
#76322=CARTESIAN_POINT('',(18.3,92.08,7.45));
#76323=CARTESIAN_POINT('',(18.18,92.08,9.4));
#76324=CARTESIAN_POINT('',(18.3,92.08,9.4));
#76325=CARTESIAN_POINT('',(18.18,92.08,8.));
#76326=CARTESIAN_POINT('Origin',(18.3,91.92,9.4));
#76327=CARTESIAN_POINT('',(18.3,91.92,9.4));
#76328=CARTESIAN_POINT('',(18.3,80.96,9.4));
#76329=CARTESIAN_POINT('',(18.18,91.92,9.4));
#76330=CARTESIAN_POINT('',(18.3,91.92,9.4));
#76331=CARTESIAN_POINT('',(18.18,92.08,9.4));
#76332=CARTESIAN_POINT('Origin',(18.3,91.92,8.));
#76333=CARTESIAN_POINT('',(18.3,91.92,6.75));
#76334=CARTESIAN_POINT('',(18.18,91.92,9.4));
#76335=CARTESIAN_POINT('Origin',(18.18,92.,8.7));
#76336=CARTESIAN_POINT('Origin',(18.3,94.08,8.));
#76337=CARTESIAN_POINT('',(18.3,94.08,8.));
#76338=CARTESIAN_POINT('',(18.3,93.92,8.));
#76339=CARTESIAN_POINT('',(18.3,82.04,8.));
#76340=CARTESIAN_POINT('',(18.18,94.08,8.));
#76341=CARTESIAN_POINT('',(18.3,94.08,8.));
#76342=CARTESIAN_POINT('',(18.18,93.92,8.));
#76343=CARTESIAN_POINT('',(18.18,93.92,8.));
#76344=CARTESIAN_POINT('',(18.3,93.92,8.));
#76345=CARTESIAN_POINT('Origin',(18.3,94.08,9.4));
#76346=CARTESIAN_POINT('',(18.3,94.08,9.4));
#76347=CARTESIAN_POINT('',(18.3,94.08,7.45));
#76348=CARTESIAN_POINT('',(18.18,94.08,9.4));
#76349=CARTESIAN_POINT('',(18.3,94.08,9.4));
#76350=CARTESIAN_POINT('',(18.18,94.08,8.));
#76351=CARTESIAN_POINT('Origin',(18.3,93.92,9.4));
#76352=CARTESIAN_POINT('',(18.3,93.92,9.4));
#76353=CARTESIAN_POINT('',(18.3,81.96,9.4));
#76354=CARTESIAN_POINT('',(18.18,93.92,9.4));
#76355=CARTESIAN_POINT('',(18.3,93.92,9.4));
#76356=CARTESIAN_POINT('',(18.18,94.08,9.4));
#76357=CARTESIAN_POINT('Origin',(18.3,93.92,8.));
#76358=CARTESIAN_POINT('',(18.3,93.92,6.75));
#76359=CARTESIAN_POINT('',(18.18,93.92,9.4));
#76360=CARTESIAN_POINT('Origin',(18.18,94.,8.7));
#76361=CARTESIAN_POINT('Origin',(18.3,96.08,8.));
#76362=CARTESIAN_POINT('',(18.3,96.08,8.));
#76363=CARTESIAN_POINT('',(18.3,95.92,8.));
#76364=CARTESIAN_POINT('',(18.3,83.04,8.));
#76365=CARTESIAN_POINT('',(18.18,96.08,8.));
#76366=CARTESIAN_POINT('',(18.3,96.08,8.));
#76367=CARTESIAN_POINT('',(18.18,95.92,8.));
#76368=CARTESIAN_POINT('',(18.18,95.92,8.));
#76369=CARTESIAN_POINT('',(18.3,95.92,8.));
#76370=CARTESIAN_POINT('Origin',(18.3,96.08,9.4));
#76371=CARTESIAN_POINT('',(18.3,96.08,9.4));
#76372=CARTESIAN_POINT('',(18.3,96.08,7.45));
#76373=CARTESIAN_POINT('',(18.18,96.08,9.4));
#76374=CARTESIAN_POINT('',(18.3,96.08,9.4));
#76375=CARTESIAN_POINT('',(18.18,96.08,8.));
#76376=CARTESIAN_POINT('Origin',(18.3,95.92,9.4));
#76377=CARTESIAN_POINT('',(18.3,95.92,9.4));
#76378=CARTESIAN_POINT('',(18.3,82.96,9.4));
#76379=CARTESIAN_POINT('',(18.18,95.92,9.4));
#76380=CARTESIAN_POINT('',(18.3,95.92,9.4));
#76381=CARTESIAN_POINT('',(18.18,96.08,9.4));
#76382=CARTESIAN_POINT('Origin',(18.3,95.92,8.));
#76383=CARTESIAN_POINT('',(18.3,95.92,6.75));
#76384=CARTESIAN_POINT('',(18.18,95.92,9.4));
#76385=CARTESIAN_POINT('Origin',(18.18,96.,8.7));
#76386=CARTESIAN_POINT('Origin',(18.3,98.08,8.));
#76387=CARTESIAN_POINT('',(18.3,98.08,8.));
#76388=CARTESIAN_POINT('',(18.3,97.92,8.));
#76389=CARTESIAN_POINT('',(18.3,84.04,8.));
#76390=CARTESIAN_POINT('',(18.18,98.08,8.));
#76391=CARTESIAN_POINT('',(18.3,98.08,8.));
#76392=CARTESIAN_POINT('',(18.18,97.92,8.));
#76393=CARTESIAN_POINT('',(18.18,97.92,8.));
#76394=CARTESIAN_POINT('',(18.3,97.92,8.));
#76395=CARTESIAN_POINT('Origin',(18.3,98.08,9.4));
#76396=CARTESIAN_POINT('',(18.3,98.08,9.4));
#76397=CARTESIAN_POINT('',(18.3,98.08,7.45));
#76398=CARTESIAN_POINT('',(18.18,98.08,9.4));
#76399=CARTESIAN_POINT('',(18.3,98.08,9.4));
#76400=CARTESIAN_POINT('',(18.18,98.08,8.));
#76401=CARTESIAN_POINT('Origin',(18.3,97.92,9.4));
#76402=CARTESIAN_POINT('',(18.3,97.92,9.4));
#76403=CARTESIAN_POINT('',(18.3,83.96,9.4));
#76404=CARTESIAN_POINT('',(18.18,97.92,9.4));
#76405=CARTESIAN_POINT('',(18.3,97.92,9.4));
#76406=CARTESIAN_POINT('',(18.18,98.08,9.4));
#76407=CARTESIAN_POINT('Origin',(18.3,97.92,8.));
#76408=CARTESIAN_POINT('',(18.3,97.92,6.75));
#76409=CARTESIAN_POINT('',(18.18,97.92,9.4));
#76410=CARTESIAN_POINT('Origin',(18.18,98.,8.7));
#76411=CARTESIAN_POINT('Origin',(18.3,100.08,6.4));
#76412=CARTESIAN_POINT('',(18.3,100.08,6.4));
#76413=CARTESIAN_POINT('',(18.3,99.92,6.4));
#76414=CARTESIAN_POINT('',(18.3,85.04,6.4));
#76415=CARTESIAN_POINT('',(18.18,100.08,6.4));
#76416=CARTESIAN_POINT('',(18.3,100.08,6.4));
#76417=CARTESIAN_POINT('',(18.18,99.92,6.4));
#76418=CARTESIAN_POINT('',(18.18,99.92,6.4));
#76419=CARTESIAN_POINT('',(18.3,99.92,6.4));
#76420=CARTESIAN_POINT('Origin',(18.3,100.08,9.4));
#76421=CARTESIAN_POINT('',(18.3,100.08,9.4));
#76422=CARTESIAN_POINT('',(18.3,100.08,7.45));
#76423=CARTESIAN_POINT('',(18.18,100.08,9.4));
#76424=CARTESIAN_POINT('',(18.3,100.08,9.4));
#76425=CARTESIAN_POINT('',(18.18,100.08,6.4));
#76426=CARTESIAN_POINT('Origin',(18.3,99.92,9.4));
#76427=CARTESIAN_POINT('',(18.3,99.92,9.4));
#76428=CARTESIAN_POINT('',(18.3,84.96,9.4));
#76429=CARTESIAN_POINT('',(18.18,99.92,9.4));
#76430=CARTESIAN_POINT('',(18.3,99.92,9.4));
#76431=CARTESIAN_POINT('',(18.18,100.08,9.4));
#76432=CARTESIAN_POINT('Origin',(18.3,99.92,6.4));
#76433=CARTESIAN_POINT('',(18.3,99.92,5.95));
#76434=CARTESIAN_POINT('',(18.18,99.92,9.4));
#76435=CARTESIAN_POINT('Origin',(18.18,100.,7.9));
#76436=CARTESIAN_POINT('Origin',(18.3,102.08,8.));
#76437=CARTESIAN_POINT('',(18.3,102.08,8.));
#76438=CARTESIAN_POINT('',(18.3,101.92,8.));
#76439=CARTESIAN_POINT('',(18.3,86.04,8.));
#76440=CARTESIAN_POINT('',(18.18,102.08,8.));
#76441=CARTESIAN_POINT('',(18.3,102.08,8.));
#76442=CARTESIAN_POINT('',(18.18,101.92,8.));
#76443=CARTESIAN_POINT('',(18.18,101.92,8.));
#76444=CARTESIAN_POINT('',(18.3,101.92,8.));
#76445=CARTESIAN_POINT('Origin',(18.3,102.08,9.4));
#76446=CARTESIAN_POINT('',(18.3,102.08,9.4));
#76447=CARTESIAN_POINT('',(18.3,102.08,7.45));
#76448=CARTESIAN_POINT('',(18.18,102.08,9.4));
#76449=CARTESIAN_POINT('',(18.3,102.08,9.4));
#76450=CARTESIAN_POINT('',(18.18,102.08,8.));
#76451=CARTESIAN_POINT('Origin',(18.3,101.92,9.4));
#76452=CARTESIAN_POINT('',(18.3,101.92,9.4));
#76453=CARTESIAN_POINT('',(18.3,85.96,9.4));
#76454=CARTESIAN_POINT('',(18.18,101.92,9.4));
#76455=CARTESIAN_POINT('',(18.3,101.92,9.4));
#76456=CARTESIAN_POINT('',(18.18,102.08,9.4));
#76457=CARTESIAN_POINT('Origin',(18.3,101.92,8.));
#76458=CARTESIAN_POINT('',(18.3,101.92,6.75));
#76459=CARTESIAN_POINT('',(18.18,101.92,9.4));
#76460=CARTESIAN_POINT('Origin',(18.18,102.,8.7));
#76461=CARTESIAN_POINT('Origin',(18.3,104.08,8.));
#76462=CARTESIAN_POINT('',(18.3,104.08,8.));
#76463=CARTESIAN_POINT('',(18.3,103.92,8.));
#76464=CARTESIAN_POINT('',(18.3,87.04,8.));
#76465=CARTESIAN_POINT('',(18.18,104.08,8.));
#76466=CARTESIAN_POINT('',(18.3,104.08,8.));
#76467=CARTESIAN_POINT('',(18.18,103.92,8.));
#76468=CARTESIAN_POINT('',(18.18,103.92,8.));
#76469=CARTESIAN_POINT('',(18.3,103.92,8.));
#76470=CARTESIAN_POINT('Origin',(18.3,104.08,9.4));
#76471=CARTESIAN_POINT('',(18.3,104.08,9.4));
#76472=CARTESIAN_POINT('',(18.3,104.08,7.45));
#76473=CARTESIAN_POINT('',(18.18,104.08,9.4));
#76474=CARTESIAN_POINT('',(18.3,104.08,9.4));
#76475=CARTESIAN_POINT('',(18.18,104.08,8.));
#76476=CARTESIAN_POINT('Origin',(18.3,103.92,9.4));
#76477=CARTESIAN_POINT('',(18.3,103.92,9.4));
#76478=CARTESIAN_POINT('',(18.3,86.96,9.4));
#76479=CARTESIAN_POINT('',(18.18,103.92,9.4));
#76480=CARTESIAN_POINT('',(18.3,103.92,9.4));
#76481=CARTESIAN_POINT('',(18.18,104.08,9.4));
#76482=CARTESIAN_POINT('Origin',(18.3,103.92,8.));
#76483=CARTESIAN_POINT('',(18.3,103.92,6.75));
#76484=CARTESIAN_POINT('',(18.18,103.92,9.4));
#76485=CARTESIAN_POINT('Origin',(18.18,104.,8.7));
#76486=CARTESIAN_POINT('Origin',(18.3,106.08,8.));
#76487=CARTESIAN_POINT('',(18.3,106.08,8.));
#76488=CARTESIAN_POINT('',(18.3,105.92,8.));
#76489=CARTESIAN_POINT('',(18.3,88.04,8.));
#76490=CARTESIAN_POINT('',(18.18,106.08,8.));
#76491=CARTESIAN_POINT('',(18.3,106.08,8.));
#76492=CARTESIAN_POINT('',(18.18,105.92,8.));
#76493=CARTESIAN_POINT('',(18.18,105.92,8.));
#76494=CARTESIAN_POINT('',(18.3,105.92,8.));
#76495=CARTESIAN_POINT('Origin',(18.3,106.08,9.4));
#76496=CARTESIAN_POINT('',(18.3,106.08,9.4));
#76497=CARTESIAN_POINT('',(18.3,106.08,7.45));
#76498=CARTESIAN_POINT('',(18.18,106.08,9.4));
#76499=CARTESIAN_POINT('',(18.3,106.08,9.4));
#76500=CARTESIAN_POINT('',(18.18,106.08,8.));
#76501=CARTESIAN_POINT('Origin',(18.3,105.92,9.4));
#76502=CARTESIAN_POINT('',(18.3,105.92,9.4));
#76503=CARTESIAN_POINT('',(18.3,87.96,9.4));
#76504=CARTESIAN_POINT('',(18.18,105.92,9.4));
#76505=CARTESIAN_POINT('',(18.3,105.92,9.4));
#76506=CARTESIAN_POINT('',(18.18,106.08,9.4));
#76507=CARTESIAN_POINT('Origin',(18.3,105.92,8.));
#76508=CARTESIAN_POINT('',(18.3,105.92,6.75));
#76509=CARTESIAN_POINT('',(18.18,105.92,9.4));
#76510=CARTESIAN_POINT('Origin',(18.18,106.,8.7));
#76511=CARTESIAN_POINT('Origin',(18.3,108.08,8.));
#76512=CARTESIAN_POINT('',(18.3,108.08,8.));
#76513=CARTESIAN_POINT('',(18.3,107.92,8.));
#76514=CARTESIAN_POINT('',(18.3,89.04,8.));
#76515=CARTESIAN_POINT('',(18.18,108.08,8.));
#76516=CARTESIAN_POINT('',(18.3,108.08,8.));
#76517=CARTESIAN_POINT('',(18.18,107.92,8.));
#76518=CARTESIAN_POINT('',(18.18,107.92,8.));
#76519=CARTESIAN_POINT('',(18.3,107.92,8.));
#76520=CARTESIAN_POINT('Origin',(18.3,108.08,9.4));
#76521=CARTESIAN_POINT('',(18.3,108.08,9.4));
#76522=CARTESIAN_POINT('',(18.3,108.08,7.45));
#76523=CARTESIAN_POINT('',(18.18,108.08,9.4));
#76524=CARTESIAN_POINT('',(18.3,108.08,9.4));
#76525=CARTESIAN_POINT('',(18.18,108.08,8.));
#76526=CARTESIAN_POINT('Origin',(18.3,107.92,9.4));
#76527=CARTESIAN_POINT('',(18.3,107.92,9.4));
#76528=CARTESIAN_POINT('',(18.3,88.96,9.4));
#76529=CARTESIAN_POINT('',(18.18,107.92,9.4));
#76530=CARTESIAN_POINT('',(18.3,107.92,9.4));
#76531=CARTESIAN_POINT('',(18.18,108.08,9.4));
#76532=CARTESIAN_POINT('Origin',(18.3,107.92,8.));
#76533=CARTESIAN_POINT('',(18.3,107.92,6.75));
#76534=CARTESIAN_POINT('',(18.18,107.92,9.4));
#76535=CARTESIAN_POINT('Origin',(18.18,108.,8.7));
#76536=CARTESIAN_POINT('Origin',(18.3,110.08,6.4));
#76537=CARTESIAN_POINT('',(18.3,110.08,6.4));
#76538=CARTESIAN_POINT('',(18.3,109.92,6.4));
#76539=CARTESIAN_POINT('',(18.3,90.04,6.4));
#76540=CARTESIAN_POINT('',(18.18,110.08,6.4));
#76541=CARTESIAN_POINT('',(18.3,110.08,6.4));
#76542=CARTESIAN_POINT('',(18.18,109.92,6.4));
#76543=CARTESIAN_POINT('',(18.18,109.92,6.4));
#76544=CARTESIAN_POINT('',(18.3,109.92,6.4));
#76545=CARTESIAN_POINT('Origin',(18.3,110.08,9.4));
#76546=CARTESIAN_POINT('',(18.3,110.08,9.4));
#76547=CARTESIAN_POINT('',(18.3,110.08,7.45));
#76548=CARTESIAN_POINT('',(18.18,110.08,9.4));
#76549=CARTESIAN_POINT('',(18.3,110.08,9.4));
#76550=CARTESIAN_POINT('',(18.18,110.08,6.4));
#76551=CARTESIAN_POINT('Origin',(18.3,109.92,9.4));
#76552=CARTESIAN_POINT('',(18.3,109.92,9.4));
#76553=CARTESIAN_POINT('',(18.3,89.96,9.4));
#76554=CARTESIAN_POINT('',(18.18,109.92,9.4));
#76555=CARTESIAN_POINT('',(18.3,109.92,9.4));
#76556=CARTESIAN_POINT('',(18.18,110.08,9.4));
#76557=CARTESIAN_POINT('Origin',(18.3,109.92,6.4));
#76558=CARTESIAN_POINT('',(18.3,109.92,5.95));
#76559=CARTESIAN_POINT('',(18.18,109.92,9.4));
#76560=CARTESIAN_POINT('Origin',(18.18,110.,7.9));
#76561=CARTESIAN_POINT('Origin',(18.3,112.08,8.));
#76562=CARTESIAN_POINT('',(18.3,112.08,8.));
#76563=CARTESIAN_POINT('',(18.3,111.92,8.));
#76564=CARTESIAN_POINT('',(18.3,91.04,8.));
#76565=CARTESIAN_POINT('',(18.18,112.08,8.));
#76566=CARTESIAN_POINT('',(18.3,112.08,8.));
#76567=CARTESIAN_POINT('',(18.18,111.92,8.));
#76568=CARTESIAN_POINT('',(18.18,111.92,8.));
#76569=CARTESIAN_POINT('',(18.3,111.92,8.));
#76570=CARTESIAN_POINT('Origin',(18.3,112.08,9.4));
#76571=CARTESIAN_POINT('',(18.3,112.08,9.4));
#76572=CARTESIAN_POINT('',(18.3,112.08,7.45));
#76573=CARTESIAN_POINT('',(18.18,112.08,9.4));
#76574=CARTESIAN_POINT('',(18.3,112.08,9.4));
#76575=CARTESIAN_POINT('',(18.18,112.08,8.));
#76576=CARTESIAN_POINT('Origin',(18.3,111.92,9.4));
#76577=CARTESIAN_POINT('',(18.3,111.92,9.4));
#76578=CARTESIAN_POINT('',(18.3,90.96,9.4));
#76579=CARTESIAN_POINT('',(18.18,111.92,9.4));
#76580=CARTESIAN_POINT('',(18.3,111.92,9.4));
#76581=CARTESIAN_POINT('',(18.18,112.08,9.4));
#76582=CARTESIAN_POINT('Origin',(18.3,111.92,8.));
#76583=CARTESIAN_POINT('',(18.3,111.92,6.75));
#76584=CARTESIAN_POINT('',(18.18,111.92,9.4));
#76585=CARTESIAN_POINT('Origin',(18.18,112.,8.7));
#76586=CARTESIAN_POINT('Origin',(17.5,15.,5.5));
#76587=CARTESIAN_POINT('',(17.5,15.,6.6));
#76588=CARTESIAN_POINT('Origin',(17.5,15.,5.5));
#76589=CARTESIAN_POINT('',(18.3,15.,6.6));
#76590=CARTESIAN_POINT('',(17.5,15.,6.6));
#76591=CARTESIAN_POINT('Origin',(18.3,15.,5.5));
#76592=CARTESIAN_POINT('Origin',(17.5,125.,5.5));
#76593=CARTESIAN_POINT('',(17.5,125.,6.6));
#76594=CARTESIAN_POINT('Origin',(17.5,125.,5.5));
#76595=CARTESIAN_POINT('',(18.3,125.,6.6));
#76596=CARTESIAN_POINT('',(17.5,125.,6.6));
#76597=CARTESIAN_POINT('Origin',(18.3,125.,5.5));
#76598=CARTESIAN_POINT('Origin',(17.5,11.,9.2));
#76599=CARTESIAN_POINT('',(17.5,11.,9.2));
#76600=CARTESIAN_POINT('',(17.5,11.,1.8));
#76601=CARTESIAN_POINT('',(17.5,11.,9.2));
#76602=CARTESIAN_POINT('',(18.3,11.,1.8));
#76603=CARTESIAN_POINT('',(17.5,11.,1.8));
#76604=CARTESIAN_POINT('',(18.3,11.,9.2));
#76605=CARTESIAN_POINT('',(18.3,11.,9.2));
#76606=CARTESIAN_POINT('',(17.5,11.,9.2));
#76607=CARTESIAN_POINT('Origin',(17.5,11.8,9.2));
#76608=CARTESIAN_POINT('',(17.5,11.8,10.));
#76609=CARTESIAN_POINT('Origin',(17.5,11.8,9.2));
#76610=CARTESIAN_POINT('',(18.3,11.8,10.));
#76611=CARTESIAN_POINT('Origin',(18.3,11.8,9.2));
#76612=CARTESIAN_POINT('',(17.5,11.8,10.));
#76613=CARTESIAN_POINT('Origin',(17.5,128.2,10.));
#76614=CARTESIAN_POINT('',(17.5,128.2,10.));
#76615=CARTESIAN_POINT('',(17.5,128.2,10.));
#76616=CARTESIAN_POINT('',(18.3,128.2,10.));
#76617=CARTESIAN_POINT('',(18.3,128.2,10.));
#76618=CARTESIAN_POINT('',(17.5,128.2,10.));
#76619=CARTESIAN_POINT('Origin',(17.5,128.2,9.19999999999997));
#76620=CARTESIAN_POINT('',(17.5,129.,9.2));
#76621=CARTESIAN_POINT('Origin',(17.5,128.2,9.19999999999997));
#76622=CARTESIAN_POINT('',(18.3,129.,9.2));
#76623=CARTESIAN_POINT('Origin',(18.3,128.2,9.19999999999997));
#76624=CARTESIAN_POINT('',(17.5,129.,9.2));
#76625=CARTESIAN_POINT('Origin',(17.5,129.,1.8));
#76626=CARTESIAN_POINT('',(17.5,129.,1.8));
#76627=CARTESIAN_POINT('',(17.5,129.,1.8));
#76628=CARTESIAN_POINT('',(18.3,129.,1.8));
#76629=CARTESIAN_POINT('',(18.3,129.,1.8));
#76630=CARTESIAN_POINT('',(17.5,129.,1.8));
#76631=CARTESIAN_POINT('Origin',(17.5,128.2,1.80000000000003));
#76632=CARTESIAN_POINT('',(17.5,128.2,1.));
#76633=CARTESIAN_POINT('Origin',(17.5,128.2,1.80000000000003));
#76634=CARTESIAN_POINT('',(18.3,128.2,1.));
#76635=CARTESIAN_POINT('Origin',(18.3,128.2,1.80000000000003));
#76636=CARTESIAN_POINT('',(17.5,128.2,1.));
#76637=CARTESIAN_POINT('Origin',(17.5,11.8,1.));
#76638=CARTESIAN_POINT('',(17.5,11.8,1.));
#76639=CARTESIAN_POINT('',(17.5,11.8,1.));
#76640=CARTESIAN_POINT('',(18.3,11.8,1.));
#76641=CARTESIAN_POINT('',(18.3,11.8,1.));
#76642=CARTESIAN_POINT('',(17.5,11.8,1.));
#76643=CARTESIAN_POINT('Origin',(17.5,11.8,1.8));
#76644=CARTESIAN_POINT('Origin',(17.5,11.8,1.8));
#76645=CARTESIAN_POINT('Origin',(18.3,11.8,1.8));
#76646=CARTESIAN_POINT('Origin',(18.3,70.,5.5));
#76647=CARTESIAN_POINT('Origin',(17.5,70.,5.5));
#135259=UNCERTAINTY_MEASURE_WITH_UNIT(LENGTH_MEASURE(0.01),#135283,
'DISTANCE_ACCURACY_VALUE',
'Maximum model space distance between geometric entities at asserted c
onnectivities');
#135267=UNCERTAINTY_MEASURE_WITH_UNIT(LENGTH_MEASURE(0.01),#135283,
'DISTANCE_ACCURACY_VALUE',
'Maximum model space distance between geometric entities at asserted c
onnectivities');
#135274=(
GEOMETRIC_REPRESENTATION_CONTEXT(3)
GLOBAL_UNCERTAINTY_ASSIGNED_CONTEXT((#135259))
GLOBAL_UNIT_ASSIGNED_CONTEXT((#135283,#135285,#135286))
REPRESENTATION_CONTEXT('','3D')
);
#135282=(
GEOMETRIC_REPRESENTATION_CONTEXT(3)
GLOBAL_UNCERTAINTY_ASSIGNED_CONTEXT((#135267))
GLOBAL_UNIT_ASSIGNED_CONTEXT((#135283,#135285,#135286))
REPRESENTATION_CONTEXT('','3D')
);
#135283=(
LENGTH_UNIT()
NAMED_UNIT(*)
SI_UNIT(.MILLI.,.METRE.)
);
#135285=(
NAMED_UNIT(*)
PLANE_ANGLE_UNIT()
SI_UNIT($,.RADIAN.)
);
#135286=(
NAMED_UNIT(*)
SI_UNIT($,.STERADIAN.)
SOLID_ANGLE_UNIT()
);
#135293=SHAPE_DEFINITION_REPRESENTATION(#135307,#135342);
#135307=PRODUCT_DEFINITION_SHAPE('',$,#135357);
#135342=SHAPE_REPRESENTATION('',(#32757),#135274);
#135350=PRODUCT_DEFINITION_CONTEXT('part definition',#135394,'design');
#135357=PRODUCT_DEFINITION('2026-10-15-19-09-11-261',
'Stainless Scale Plate 0.1 mm Vernier',#135371,#135350);
#135371=PRODUCT_DEFINITION_FORMATION('',$,#135402);
#135394=APPLICATION_CONTEXT(
'Core Data for Automotive Mechanical Design Process');
#135395=PRODUCT_CONTEXT('part definition',#135394,'mechanical');
#135402=PRODUCT('2026-10-15-19-09-11-261',
'Stainless Scale Plate 0.1 mm Vernier',$,(#135395));
#135416=PRESENTATION_STYLE_ASSIGNMENT((#135430));
#135430=SURFACE_STYLE_USAGE(.BOTH.,#135444);
#135444=SURFACE_SIDE_STYLE('',(#135458));
#135458=SURFACE_STYLE_FILL_AREA(#135472);
#135472=FILL_AREA_STYLE('Opaque(238,239,241)',(#135486));
#135486=FILL_AREA_STYLE_COLOUR('Opaque(238,239,241)',#135500);
#135500=COLOUR_RGB('Opaque(238,239,241)', 0.08235294, 0.09019608, 0.10196078);
ENDSEC;
END-ISO-10303-21;
